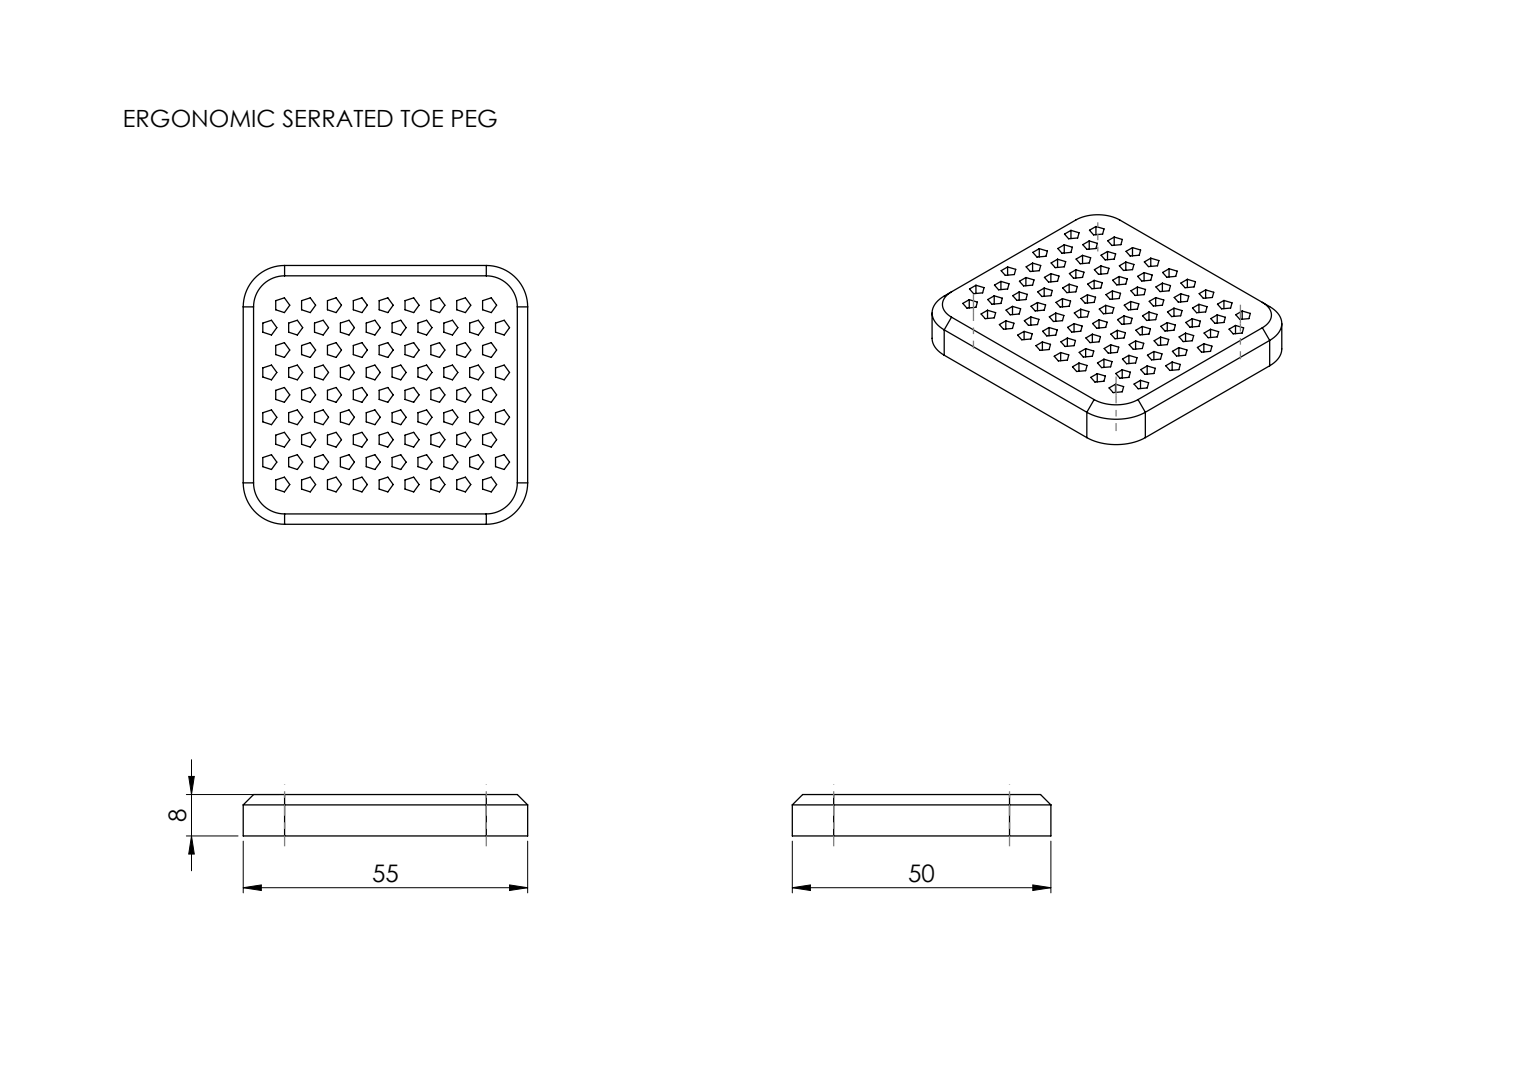
ISO-10303-21;
HEADER;
FILE_DESCRIPTION (('STEP AP214'),
    '1' );
FILE_NAME ('Ergonomic Serrated Toe Peg.step',
    '2026-09-30T16:28:02',
    ( '' ),
    ( '' ),
    'SwSTEP 2.0',
    'SolidWorks 2026',
    '' );
FILE_SCHEMA (( 'AUTOMOTIVE_DESIGN' ));
ENDSEC;

DATA;
#1=CARTESIAN_POINT ( 'NONE',  ( 171.1922820468852819, -9.999999999999996447, -4.936203717676158398 ) ) ;
#2=LINE ( 'NONE', #9287, #2166 ) ;
#6=ORIENTED_EDGE ( 'NONE', *, *, #8201, .T. ) ;
#8=EDGE_LOOP ( 'NONE', ( #13410, #18933, #24855, #7147 ) ) ;
#9=CARTESIAN_POINT ( 'NONE',  ( 158.6922820468853104, -1.999999999999974909, -0.6060766987539614181 ) ) ;
#13=AXIS2_PLACEMENT_3D ( 'NONE', #28994, #19329, #14737 ) ;
#14=VERTEX_POINT ( 'NONE', #15281 ) ;
#16=CARTESIAN_POINT ( 'NONE',  ( 176.1922820468852535, -9.999999999999994671, -4.936203717676158398 ) ) ;
#19=CARTESIAN_POINT ( 'NONE',  ( 129.5152310637605524, -10.00000000000000888, -21.71180489736090991 ) ) ;
#20=LINE ( 'NONE', #28431, #3804 ) ;
#22=ORIENTED_EDGE ( 'NONE', *, *, #9858, .T. ) ;
#23=DIRECTION ( 'NONE',  ( -0.5877852522924731371, 0.000000000000000000, 0.8090169943749474513 ) ) ;
#24=EDGE_LOOP ( 'NONE', ( #18208, #203, #15820, #9762, #20509 ) ) ;
#27=EDGE_CURVE ( 'NONE', #25495, #12783, #12701, .T. ) ;
#30=ORIENTED_EDGE ( 'NONE', *, *, #5505, .F. ) ;
#31=EDGE_CURVE ( 'NONE', #25811, #28060, #3559, .T. ) ;
#32=FACE_OUTER_BOUND ( 'NONE', #14723, .T. ) ;
#33=CARTESIAN_POINT ( 'NONE',  ( 142.0152310637605524, -1.999999999999978684, 1.702185954127501066 ) ) ;
#34=VECTOR ( 'NONE', #18733, 1000.000000000000000 ) ;
#36=AXIS2_PLACEMENT_3D ( 'NONE', #24795, #28817, #15305 ) ;
#38=VECTOR ( 'NONE', #16062, 999.9999999999998863 ) ;
#40=ORIENTED_EDGE ( 'NONE', *, *, #8836, .F. ) ;
#41=DIRECTION ( 'NONE',  ( -2.698458740408365879E-16, 1.000000000000000000, 0.000000000000000000 ) ) ;
#43=EDGE_LOOP ( 'NONE', ( #10791, #17120, #27313, #27403, #18272 ) ) ;
#45=DIRECTION ( 'NONE',  ( 2.908569913943825554E-16, -1.000000000000000000, 0.000000000000000000 ) ) ;
#46=ORIENTED_EDGE ( 'NONE', *, *, #12896, .F. ) ;
#47=CARTESIAN_POINT ( 'NONE',  ( 149.7287565553229456, -10.00000000000000355, 0.8205080756887930260 ) ) ;
#49=LINE ( 'NONE', #2798, #15810 ) ;
#50=EDGE_LOOP ( 'NONE', ( #6565, #21196, #16941, #11430, #26912 ) ) ;
#52=EDGE_LOOP ( 'NONE', ( #7879, #12886, #2199, #3337, #17093, #20123 ) ) ;
#55=ORIENTED_EDGE ( 'NONE', *, *, #7367, .F. ) ;
#57=CARTESIAN_POINT ( 'NONE',  ( 142.2287565553230309, -10.00000000000000533, -29.49038105676660138 ) ) ;
#59=ORIENTED_EDGE ( 'NONE', *, *, #1895, .T. ) ;
#60=LINE ( 'NONE', #7229, #30116 ) ;
#62=EDGE_CURVE ( 'NONE', #29710, #22500, #27244, .T. ) ;
#65=ADVANCED_FACE ( 'NONE', ( #1579 ), #24770, .T. ) ;
#69=EDGE_LOOP ( 'NONE', ( #19720, #1724, #9767, #14173 ) ) ;
#70=PLANE ( 'NONE',  #26676 ) ;
#71=ORIENTED_EDGE ( 'NONE', *, *, #5370, .F. ) ;
#75=ORIENTED_EDGE ( 'NONE', *, *, #15408, .T. ) ;
#76=VECTOR ( 'NONE', #4215, 1000.000000000000000 ) ;
#77=CARTESIAN_POINT ( 'NONE',  ( 133.7287565553229456, -4.999999999999982236, 3.500000000000003109 ) ) ;
#78=VECTOR ( 'NONE', #21293, 999.9999999999998863 ) ;
#79=LINE ( 'NONE', #18686, #13812 ) ;
#80=DIRECTION ( 'NONE',  ( 0.9510565162951536422, 0.000000000000000000, -0.3090169943749475623 ) ) ;
#81=CARTESIAN_POINT ( 'NONE',  ( 164.5152310637605240, -9.999999999999996447, -28.60870317832789667 ) ) ;
#82=DIRECTION ( 'NONE',  ( -1.110223024625156540E-16, 0.000000000000000000, -1.000000000000000000 ) ) ;
#86=EDGE_CURVE ( 'NONE', #12166, #722, #15592, .T. ) ;
#90=PLANE ( 'NONE',  #29362 ) ;
#91=DIRECTION ( 'NONE',  ( -2.698458740408365879E-16, 1.000000000000000000, 0.000000000000000000 ) ) ;
#92=DIRECTION ( 'NONE',  ( -0.9510565162951536422, 0.000000000000000000, -0.3090169943749472292 ) ) ;
#93=ORIENTED_EDGE ( 'NONE', *, *, #14811, .T. ) ;
#96=ORIENTED_EDGE ( 'NONE', *, *, #21204, .F. ) ;
#97=CARTESIAN_POINT ( 'NONE',  ( 164.5152310637604671, -9.999999999999998224, -11.28819510263909542 ) ) ;
#98=CARTESIAN_POINT ( 'NONE',  ( 152.0152310637604671, -4.999999999999976907, -0.06116980274991495881 ) ) ;
#99=ADVANCED_FACE ( 'NONE', ( #8123 ), #7974, .T. ) ;
#102=VERTEX_POINT ( 'NONE', #17428 ) ;
#105=EDGE_LOOP ( 'NONE', ( #1685, #5636, #6833, #29745, #13110 ) ) ;
#110=ORIENTED_EDGE ( 'NONE', *, *, #8360, .T. ) ;
#113=EDGE_LOOP ( 'NONE', ( #1842, #6412, #14178, #16562 ) ) ;
#114=CARTESIAN_POINT ( 'NONE',  ( 141.1922820468854525, -10.00000000000000533, -30.91696583120935671 ) ) ;
#115=CARTESIAN_POINT ( 'NONE',  ( 171.1922820468853388, -4.999999999999971578, -19.40354224447947828 ) ) ;
#117=VERTEX_POINT ( 'NONE', #8423 ) ;
#118=CARTESIAN_POINT ( 'NONE',  ( 134.5152310637605524, -1.999999999999980460, -4.391296821672111328 ) ) ;
#119=FACE_OUTER_BOUND ( 'NONE', #9403, .T. ) ;
#122=ORIENTED_EDGE ( 'NONE', *, *, #28451, .T. ) ;
#123=AXIS2_PLACEMENT_3D ( 'NONE', #1550, #9129, #25482 ) ;
#124=DIRECTION ( 'NONE',  ( 0.9510565162951536422, 0.000000000000000000, -0.3090169943749475623 ) ) ;
#125=CARTESIAN_POINT ( 'NONE',  ( 158.6922820468854241, -1.999999999999973133, -35.24709285013155835 ) ) ;
#128=CARTESIAN_POINT ( 'NONE',  ( 174.5152310637604955, -1.999999999999968914, -28.60870317832789667 ) ) ;
#130=DIRECTION ( 'NONE',  ( -0.5877852522924731371, -1.586114251531760728E-16, -0.8090169943749474513 ) ) ;
#131=EDGE_CURVE ( 'NONE', #19668, #13066, #17725, .T. ) ;
#132=LINE ( 'NONE', #2726, #539 ) ;
#133=VECTOR ( 'NONE', #22097, 1000.000000000000000 ) ;
#134=VERTEX_POINT ( 'NONE', #3860 ) ;
#136=LINE ( 'NONE', #8159, #30161 ) ;
#142=ORIENTED_EDGE ( 'NONE', *, *, #977, .F. ) ;
#144=FACE_OUTER_BOUND ( 'NONE', #11125, .T. ) ;
#146=DIRECTION ( 'NONE',  ( 0.5877852522924731371, 1.586114251531760728E-16, 0.8090169943749474513 ) ) ;
#148=AXIS2_PLACEMENT_3D ( 'NONE', #18004, #8395, #8543 ) ;
#152=LINE ( 'NONE', #16311, #22917 ) ;
#154=VECTOR ( 'NONE', #27172, 1000.000000000000000 ) ;
#155=EDGE_CURVE ( 'NONE', #6429, #19044, #27953, .T. ) ;
#161=ORIENTED_EDGE ( 'NONE', *, *, #1761, .F. ) ;
#162=LINE ( 'NONE', #17082, #29052 ) ;
#165=CARTESIAN_POINT ( 'NONE',  ( 21.73040598723229877, -5.000000000000011546, -66.87931276303945083 ) ) ;
#166=EDGE_LOOP ( 'NONE', ( #11300, #21186, #18431, #15934 ) ) ;
#167=VECTOR ( 'NONE', #27934, 1000.000000000000000 ) ;
#168=ORIENTED_EDGE ( 'NONE', *, *, #18099, .T. ) ;
#170=CARTESIAN_POINT ( 'NONE',  ( 125.7287565553229172, -4.000000000000003553, -33.50000000000000000 ) ) ;
#172=DIRECTION ( 'NONE',  ( -0.9510565162951536422, -2.566386769018988323E-16, 0.3090169943749475623 ) ) ;
#173=CARTESIAN_POINT ( 'NONE',  ( 136.1922820468854241, -1.999999999999980460, -19.40354224447947473 ) ) ;
#176=CARTESIAN_POINT ( 'NONE',  ( 168.6922820468853104, -9.999999999999998224, -6.413161187712876909 ) ) ;
#177=ORIENTED_EDGE ( 'NONE', *, *, #22974, .T. ) ;
#178=EDGE_CURVE ( 'NONE', #21232, #6302, #23638, .T. ) ;
#180=ORIENTED_EDGE ( 'NONE', *, *, #14435, .F. ) ;
#185=LINE ( 'NONE', #484, #11097 ) ;
#187=DIRECTION ( 'NONE',  ( -0.5877852522924731371, -1.586114251531760728E-16, -0.8090169943749474513 ) ) ;
#191=ORIENTED_EDGE ( 'NONE', *, *, #12444, .F. ) ;
#192=FACE_BOUND ( 'NONE', #6466, .T. ) ;
#193=ORIENTED_EDGE ( 'NONE', *, *, #2861, .F. ) ;
#194=EDGE_CURVE ( 'NONE', #21176, #29420, #19051, .T. ) ;
#195=ADVANCED_FACE ( 'NONE', ( #2293 ), #12020, .T. ) ;
#196=FACE_OUTER_BOUND ( 'NONE', #7916, .T. ) ;
#197=DIRECTION ( 'NONE',  ( -0.5877852522924731371, -1.586114251531760728E-16, -0.8090169943749474513 ) ) ;
#198=LINE ( 'NONE', #11177, #23639 ) ;
#199=VECTOR ( 'NONE', #16621, 1000.000000000000000 ) ;
#201=CARTESIAN_POINT ( 'NONE',  ( 11.95300070842526274, -5.000000000000014211, 36.78755350016455594 ) ) ;
#203=ORIENTED_EDGE ( 'NONE', *, *, #27651, .T. ) ;
#205=ORIENTED_EDGE ( 'NONE', *, *, #21724, .F. ) ;
#207=DIRECTION ( 'NONE',  ( -0.9510565162951536422, -2.566386769018988323E-16, 0.3090169943749475623 ) ) ;
#208=CARTESIAN_POINT ( 'NONE',  ( 161.1922820468853388, -9.999999999999998224, -13.59645775552055902 ) ) ;
#209=VERTEX_POINT ( 'NONE', #7460 ) ;
#212=FACE_OUTER_BOUND ( 'NONE', #25235, .T. ) ;
#214=ORIENTED_EDGE ( 'NONE', *, *, #14160, .F. ) ;
#216=CARTESIAN_POINT ( 'NONE',  ( 172.7287565553229456, -1.999999999999974021, -33.50000000000000000 ) ) ;
#217=ORIENTED_EDGE ( 'NONE', *, *, #1804, .F. ) ;
#218=CARTESIAN_POINT ( 'NONE',  ( 164.5152310637604671, -4.999999999999973355, -1.826485974285146553E-14 ) ) ;
#220=VERTEX_POINT ( 'NONE', #14001 ) ;
#221=DIRECTION ( 'NONE',  ( 0.9510565162951536422, 0.000000000000000000, -0.3090169943749475623 ) ) ;
#222=ORIENTED_EDGE ( 'NONE', *, *, #14772, .T. ) ;
#225=VECTOR ( 'NONE', #26675, 1000.000000000000000 ) ;
#226=ORIENTED_EDGE ( 'NONE', *, *, #24841, .F. ) ;
#227=ORIENTED_EDGE ( 'NONE', *, *, #21857, .F. ) ;
#228=CARTESIAN_POINT ( 'NONE',  ( 163.6922820468852819, -9.999999999999998224, -0.6060766987539614181 ) ) ;
#229=CARTESIAN_POINT ( 'NONE',  ( 151.1922820468853672, -1.999999999999976685, -2.083034168790677043 ) ) ;
#230=EDGE_CURVE ( 'NONE', #17843, #12321, #21337, .T. ) ;
#231=EDGE_CURVE ( 'NONE', #23545, #23604, #24924, .T. ) ;
#232=DIRECTION ( 'NONE',  ( -2.698458740408365879E-16, 1.000000000000000000, 0.000000000000000000 ) ) ;
#233=DIRECTION ( 'NONE',  ( -2.698458740408365879E-16, 1.000000000000000000, 0.000000000000000000 ) ) ;
#234=EDGE_CURVE ( 'NONE', #25907, #1746, #23486, .T. ) ;
#235=DIRECTION ( 'NONE',  ( 0.3090169943749475623, 8.338696094058001131E-17, 0.9510565162951536422 ) ) ;
#236=EDGE_LOOP ( 'NONE', ( #22910, #13879, #24086, #12025 ) ) ;
#237=ADVANCED_FACE ( 'NONE', ( #2593 ), #18453, .T. ) ;
#244=DIRECTION ( 'NONE',  ( 0.3090169943749475623, 8.338696094058001131E-17, 0.9510565162951536422 ) ) ;
#245=VECTOR ( 'NONE', #20484, 999.9999999999998863 ) ;
#246=CARTESIAN_POINT ( 'NONE',  ( 157.0152310637605808, -4.999999999999975131, -32.93883019725009120 ) ) ;
#247=DIRECTION ( 'NONE',  ( -0.9510565162951536422, -2.566386769018988816E-16, -0.3090169943749472292 ) ) ;
#250=CARTESIAN_POINT ( 'NONE',  ( 169.5152310637604955, -1.999999999999970024, -30.37205893520531319 ) ) ;
#252=EDGE_LOOP ( 'NONE', ( #8891, #22753, #23266, #17300 ) ) ;
#253=LINE ( 'NONE', #12283, #20751 ) ;
#254=LINE ( 'NONE', #28368, #19057 ) ;
#263=ORIENTED_EDGE ( 'NONE', *, *, #16267, .F. ) ;
#264=AXIS2_PLACEMENT_3D ( 'NONE', #8989, #18309, #27664 ) ;
#265=ORIENTED_EDGE ( 'NONE', *, *, #4022, .T. ) ;
#266=DIRECTION ( 'NONE',  ( 0.9510565162951536422, 0.000000000000000000, -0.3090169943749475623 ) ) ;
#267=PLANE ( 'NONE',  #1442 ) ;
#269=PLANE ( 'NONE',  #1205 ) ;
#270=EDGE_CURVE ( 'NONE', #13418, #14798, #2444, .T. ) ;
#271=DIRECTION ( 'NONE',  ( -2.698458740408365879E-16, 1.000000000000000000, 0.000000000000000000 ) ) ;
#274=ORIENTED_EDGE ( 'NONE', *, *, #12172, .T. ) ;
#275=LINE ( 'NONE', #12157, #28348 ) ;
#276=DIRECTION ( 'NONE',  ( 0.9510565162951536422, 0.000000000000000000, -0.3090169943749475623 ) ) ;
#278=DIRECTION ( 'NONE',  ( -2.698458740408365879E-16, 1.000000000000000000, 0.000000000000000000 ) ) ;
#279=DIRECTION ( 'NONE',  ( -0.5877852522924731371, -1.586114251531760728E-16, -0.8090169943749474513 ) ) ;
#280=VERTEX_POINT ( 'NONE', #21039 ) ;
#281=VECTOR ( 'NONE', #14887, 1000.000000000000000 ) ;
#282=DIRECTION ( 'NONE',  ( -0.8090169943749474513, -2.183098979609982436E-16, 0.5877852522924731371 ) ) ;
#284=LINE ( 'NONE', #14293, #25869 ) ;
#285=ORIENTED_EDGE ( 'NONE', *, *, #11613, .T. ) ;
#286=ORIENTED_EDGE ( 'NONE', *, *, #25521, .T. ) ;
#287=DIRECTION ( 'NONE',  ( 0.9510565162951536422, 2.566386769018988816E-16, 0.3090169943749472292 ) ) ;
#288=VERTEX_POINT ( 'NONE', #4857 ) ;
#292=DIRECTION ( 'NONE',  ( -0.5877852522924731371, -1.586114251531760235E-16, 0.8090169943749474513 ) ) ;
#294=CARTESIAN_POINT ( 'NONE',  ( 176.1922820468852535, -1.999999999999970024, -4.936203717676158398 ) ) ;
#295=EDGE_CURVE ( 'NONE', #18615, #29151, #11869, .T. ) ;
#297=VECTOR ( 'NONE', #130, 1000.000000000000000 ) ;
#298=ORIENTED_EDGE ( 'NONE', *, *, #1039, .F. ) ;
#299=DIRECTION ( 'NONE',  ( -0.9510565162951536422, -2.566386769018988323E-16, 0.3090169943749475623 ) ) ;
#300=LINE ( 'NONE', #23185, #15709 ) ;
#301=VECTOR ( 'NONE', #6965, 1000.000000000000000 ) ;
#305=AXIS2_PLACEMENT_3D ( 'NONE', #1101, #17395, #12671 ) ;
#306=CARTESIAN_POINT ( 'NONE',  ( 169.7287565553228887, -9.999999999999998224, -7.839745962155603820 ) ) ;
#307=EDGE_CURVE ( 'NONE', #30043, #633, #23795, .T. ) ;
#308=EDGE_CURVE ( 'NONE', #11681, #9083, #21945, .T. ) ;
#315=DIRECTION ( 'NONE',  ( -0.5877852522924731371, -1.586114251531760728E-16, -0.8090169943749474513 ) ) ;
#318=FACE_BOUND ( 'NONE', #13580, .T. ) ;
#319=VERTEX_POINT ( 'NONE', #1201 ) ;
#320=ORIENTED_EDGE ( 'NONE', *, *, #6013, .F. ) ;
#322=CARTESIAN_POINT ( 'NONE',  ( 174.7287565553229172, -9.999999999999994671, -25.16025403784440329 ) ) ;
#325=DIRECTION ( 'NONE',  ( -0.5877852522924731371, -1.586114251531760235E-16, 0.8090169943749474513 ) ) ;
#326=PLANE ( 'NONE',  #24744 ) ;
#327=ORIENTED_EDGE ( 'NONE', *, *, #10733, .F. ) ;
#332=VECTOR ( 'NONE', #22511, 1000.000000000000000 ) ;
#336=VECTOR ( 'NONE', #15406, 1000.000000000000000 ) ;
#343=FACE_BOUND ( 'NONE', #27021, .T. ) ;
#344=VECTOR ( 'NONE', #10715, 1000.000000000000000 ) ;
#345=ORIENTED_EDGE ( 'NONE', *, *, #10601, .T. ) ;
#346=ADVANCED_FACE ( 'NONE', ( #19194 ), #5318, .T. ) ;
#348=PLANE ( 'NONE',  #22330 ) ;
#349=LINE ( 'NONE', #4913, #4348 ) ;
#350=VECTOR ( 'NONE', #1226, 1000.000000000000000 ) ;
#352=AXIS2_PLACEMENT_3D ( 'NONE', #15421, #11403, #30099 ) ;
#354=CARTESIAN_POINT ( 'NONE',  ( 151.1922820468853672, -4.999999999999976907, -4.936203717676158398 ) ) ;
#355=AXIS2_PLACEMENT_3D ( 'NONE', #20040, #29561, #1592 ) ;
#356=FACE_OUTER_BOUND ( 'NONE', #20596, .T. ) ;
#357=VERTEX_POINT ( 'NONE', #9882 ) ;
#362=CARTESIAN_POINT ( 'NONE',  ( 180.7287565553229456, -3.999999999999989786, 0.5000000000000029976 ) ) ;
#364=LINE ( 'NONE', #23553, #20283 ) ;
#366=ORIENTED_EDGE ( 'NONE', *, *, #25702, .F. ) ;
#368=LINE ( 'NONE', #18674, #9316 ) ;
#369=CARTESIAN_POINT ( 'NONE',  ( 173.6922820468853104, -9.999999999999994671, -17.92658477444275889 ) ) ;
#372=ORIENTED_EDGE ( 'NONE', *, *, #2420, .F. ) ;
#374=EDGE_CURVE ( 'NONE', #25209, #19520, #2893, .T. ) ;
#376=CIRCLE ( 'NONE', #18872, 3.000000000000002665 ) ;
#378=ORIENTED_EDGE ( 'NONE', *, *, #6683, .T. ) ;
#380=CARTESIAN_POINT ( 'NONE',  ( 144.5152310637605240, -4.999999999999978684, -4.391296821672111328 ) ) ;
#381=CARTESIAN_POINT ( 'NONE',  ( 172.7287565553229456, -3.999999999999989786, -41.50000000000000711 ) ) ;
#384=CARTESIAN_POINT ( 'NONE',  ( 174.5152310637604103, -4.999999999999970690, -1.937508276747661576E-14 ) ) ;
#385=AXIS2_PLACEMENT_3D ( 'NONE', #29992, #3996, #22923 ) ;
#386=ORIENTED_EDGE ( 'NONE', *, *, #10034, .F. ) ;
#391=ORIENTED_EDGE ( 'NONE', *, *, #6783, .T. ) ;
#393=LINE ( 'NONE', #19002, #17550 ) ;
#394=CARTESIAN_POINT ( 'NONE',  ( 151.1922820468853956, -10.00000000000000178, -10.74328820663507678 ) ) ;
#402=EDGE_LOOP ( 'NONE', ( #24156, #22408, #9241, #18567 ) ) ;
#406=ORIENTED_EDGE ( 'NONE', *, *, #21308, .T. ) ;
#408=ADVANCED_FACE ( 'NONE', ( #24392 ), #12626, .T. ) ;
#411=EDGE_CURVE ( 'NONE', #18619, #29440, #26701, .T. ) ;
#413=VECTOR ( 'NONE', #9450, 1000.000000000000000 ) ;
#415=VECTOR ( 'NONE', #2292, 1000.000000000000000 ) ;
#416=ORIENTED_EDGE ( 'NONE', *, *, #15789, .T. ) ;
#417=DIRECTION ( 'NONE',  ( 0.3090169943749475623, 8.338696094058001131E-17, 0.9510565162951536422 ) ) ;
#418=DIRECTION ( 'NONE',  ( -2.698458740408365879E-16, 1.000000000000000000, 0.000000000000000000 ) ) ;
#419=EDGE_LOOP ( 'NONE', ( #26721, #25285, #4227, #20986 ) ) ;
#420=DIRECTION ( 'NONE',  ( 0.3090169943749475623, 8.338696094058001131E-17, 0.9510565162951536422 ) ) ;
#421=LINE ( 'NONE', #18729, #12178 ) ;
#424=ORIENTED_EDGE ( 'NONE', *, *, #5508, .F. ) ;
#425=CARTESIAN_POINT ( 'NONE',  ( 18.07240892486890615, -5.000000000000012434, -55.62115542516819744 ) ) ;
#426=CARTESIAN_POINT ( 'NONE',  ( 131.1922820468854241, -1.999999999999981792, -28.06379628232387446 ) ) ;
#429=LINE ( 'NONE', #19037, #21295 ) ;
#430=ORIENTED_EDGE ( 'NONE', *, *, #4985, .T. ) ;
#431=VECTOR ( 'NONE', #12408, 1000.000000000000000 ) ;
#432=CARTESIAN_POINT ( 'NONE',  ( 159.5152310637604955, -4.999999999999974243, -11.28819510263909542 ) ) ;
#435=CARTESIAN_POINT ( 'NONE',  ( 134.5152310637605524, -1.999999999999980460, -13.05155085951650840 ) ) ;
#436=VERTEX_POINT ( 'NONE', #19791 ) ;
#439=EDGE_CURVE ( 'NONE', #26227, #4517, #895, .T. ) ;
#442=EDGE_CURVE ( 'NONE', #18552, #1065, #26238, .T. ) ;
#444=LINE ( 'NONE', #2443, #25266 ) ;
#446=EDGE_CURVE ( 'NONE', #20723, #20491, #23957, .T. ) ;
#449=ORIENTED_EDGE ( 'NONE', *, *, #11568, .T. ) ;
#450=DIRECTION ( 'NONE',  ( -1.110223024625156540E-16, 0.000000000000000000, -1.000000000000000000 ) ) ;
#452=VECTOR ( 'NONE', #19393, 1000.000000000000000 ) ;
#453=DIRECTION ( 'NONE',  ( 0.3090169943749472292, 8.338696094057992503E-17, -0.9510565162951536422 ) ) ;
#455=LINE ( 'NONE', #21049, #14790 ) ;
#457=DIRECTION ( 'NONE',  ( 1.000000000000000000, 2.698458740408365879E-16, -1.110223024625156540E-16 ) ) ;
#459=ORIENTED_EDGE ( 'NONE', *, *, #24414, .T. ) ;
#468=ORIENTED_EDGE ( 'NONE', *, *, #9842, .F. ) ;
#470=FACE_OUTER_BOUND ( 'NONE', #17896, .T. ) ;
#472=FACE_OUTER_BOUND ( 'NONE', #16901, .T. ) ;
#473=ORIENTED_EDGE ( 'NONE', *, *, #13528, .T. ) ;
#475=VERTEX_POINT ( 'NONE', #12779 ) ;
#477=ORIENTED_EDGE ( 'NONE', *, *, #15791, .T. ) ;
#482=ORIENTED_EDGE ( 'NONE', *, *, #14397, .T. ) ;
#483=EDGE_CURVE ( 'NONE', #29391, #7152, #10029, .T. ) ;
#484=CARTESIAN_POINT ( 'NONE',  ( 12.50940683846913970, -5.000000000000014211, 38.49999548658399107 ) ) ;
#485=EDGE_CURVE ( 'NONE', #18308, #9388, #28550, .T. ) ;
#486=VERTEX_POINT ( 'NONE', #7602 ) ;
#487=EDGE_CURVE ( 'NONE', #4418, #10786, #7903, .T. ) ;
#490=DIRECTION ( 'NONE',  ( -2.698458740408365879E-16, 1.000000000000000000, 0.000000000000000000 ) ) ;
#494=ORIENTED_EDGE ( 'NONE', *, *, #2114, .T. ) ;
#495=FACE_BOUND ( 'NONE', #28944, .T. ) ;
#499=VECTOR ( 'NONE', #27812, 1000.000000000000000 ) ;
#500=DIRECTION ( 'NONE',  ( 0.9510565162951536422, 2.566386769018988816E-16, 0.3090169943749472292 ) ) ;
#504=DIRECTION ( 'NONE',  ( -2.698458740408365879E-16, 1.000000000000000000, 0.000000000000000000 ) ) ;
#505=CARTESIAN_POINT ( 'NONE',  ( 162.0152310637605240, -9.999999999999998224, -34.70218595412750773 ) ) ;
#506=VERTEX_POINT ( 'NONE', #26086 ) ;
#509=LINE ( 'NONE', #21850, #18033 ) ;
#510=LINE ( 'NONE', #23703, #12518 ) ;
#511=CARTESIAN_POINT ( 'NONE',  ( 137.0152310637605808, -1.999999999999980016, 1.702185954127501066 ) ) ;
#512=ORIENTED_EDGE ( 'NONE', *, *, #5043, .F. ) ;
#513=LINE ( 'NONE', #12092, #15899 ) ;
#518=VECTOR ( 'NONE', #4177, 1000.000000000000000 ) ;
#520=EDGE_CURVE ( 'NONE', #12932, #5386, #5166, .T. ) ;
#521=CARTESIAN_POINT ( 'NONE',  ( 130.7287565553229456, -4.999999999999983125, 3.500000000000003109 ) ) ;
#524=ADVANCED_FACE ( 'NONE', ( #22562 ), #3633, .T. ) ;
#525=ORIENTED_EDGE ( 'NONE', *, *, #27075, .F. ) ;
#526=ADVANCED_FACE ( 'NONE', ( #15359 ), #12926, .T. ) ;
#527=LINE ( 'NONE', #9813, #17849 ) ;
#532=VECTOR ( 'NONE', #22824, 1000.000000000000000 ) ;
#534=LINE ( 'NONE', #822, #24024 ) ;
#535=EDGE_LOOP ( 'NONE', ( #7211, #6231, #28486, #4893 ) ) ;
#536=ORIENTED_EDGE ( 'NONE', *, *, #4318, .F. ) ;
#537=CARTESIAN_POINT ( 'NONE',  ( 146.1922820468854525, -10.00000000000000178, -22.25671179336496053 ) ) ;
#538=CARTESIAN_POINT ( 'NONE',  ( 139.5152310637605808, -10.00000000000000533, -21.71180489736090991 ) ) ;
#539=VECTOR ( 'NONE', #19186, 999.9999999999998863 ) ;
#541=DIRECTION ( 'NONE',  ( 0.000000000000000000, 0.000000000000000000, -1.000000000000000000 ) ) ;
#542=VECTOR ( 'NONE', #24235, 1000.000000000000000 ) ;
#543=CARTESIAN_POINT ( 'NONE',  ( 12.10607290817362092, -5.000000000000014211, -37.25866128932931787 ) ) ;
#544=ORIENTED_EDGE ( 'NONE', *, *, #13525, .F. ) ;
#548=EDGE_CURVE ( 'NONE', #20384, #24083, #19953, .T. ) ;
#550=ORIENTED_EDGE ( 'NONE', *, *, #23991, .F. ) ;
#552=DIRECTION ( 'NONE',  ( 0.9510565162951536422, 0.000000000000000000, -0.3090169943749475623 ) ) ;
#554=CARTESIAN_POINT ( 'NONE',  ( 148.6922820468854525, -4.999999999999976907, -23.73366926340167637 ) ) ;
#556=EDGE_LOOP ( 'NONE', ( #3105, #12356, #15207, #22632, #19486 ) ) ;
#557=FACE_OUTER_BOUND ( 'NONE', #419, .T. ) ;
#559=LINE ( 'NONE', #9844, #18339 ) ;
#560=DIRECTION ( 'NONE',  ( 2.698458740408365879E-16, -1.000000000000000000, 0.000000000000000000 ) ) ;
#563=VERTEX_POINT ( 'NONE', #10643 ) ;
#567=AXIS2_PLACEMENT_3D ( 'NONE', #11521, #19011, #13959 ) ;
#571=CARTESIAN_POINT ( 'NONE',  ( 129.5152310637605808, -10.00000000000000888, -11.28819510263909187 ) ) ;
#572=DIRECTION ( 'NONE',  ( -0.9510565162951536422, 0.000000000000000000, -0.3090169943749472292 ) ) ;
#573=ORIENTED_EDGE ( 'NONE', *, *, #19437, .T. ) ;
#574=DIRECTION ( 'NONE',  ( -0.8090169943749474513, -2.183098979609982436E-16, -0.5877852522924731371 ) ) ;
#575=DIRECTION ( 'NONE',  ( 0.9510565162951536422, 0.000000000000000000, -0.3090169943749475623 ) ) ;
#576=ADVANCED_FACE ( 'NONE', ( #3939 ), #15213, .T. ) ;
#581=DIRECTION ( 'NONE',  ( 0.3090169943749472292, 8.338696094057992503E-17, -0.9510565162951536422 ) ) ;
#582=CARTESIAN_POINT ( 'NONE',  ( 106.2677862141057545, -4.999999999999988454, -77.20806604152963359 ) ) ;
#584=CARTESIAN_POINT ( 'NONE',  ( 138.6922820468854525, -4.999999999999980460, -23.73366926340167282 ) ) ;
#585=CARTESIAN_POINT ( 'NONE',  ( 153.6922820468854241, -1.999999999999974465, -23.73366926340167637 ) ) ;
#587=DIRECTION ( 'NONE',  ( -0.5877852522924731371, 0.000000000000000000, 0.8090169943749474513 ) ) ;
#588=CARTESIAN_POINT ( 'NONE',  ( 142.0152310637605808, -1.999999999999978018, -26.04193191628310800 ) ) ;
#590=VERTEX_POINT ( 'NONE', #3789 ) ;
#591=EDGE_LOOP ( 'NONE', ( #6929, #8428, #23827, #25905 ) ) ;
#592=ORIENTED_EDGE ( 'NONE', *, *, #18201, .T. ) ;
#596=CARTESIAN_POINT ( 'NONE',  ( 143.6922820468854525, -10.00000000000000355, -17.92658477444275889 ) ) ;
#598=VECTOR ( 'NONE', #146, 1000.000000000000000 ) ;
#599=CARTESIAN_POINT ( 'NONE',  ( 15.12871522451188788, -5.000000000000013323, -46.56139778509288618 ) ) ;
#600=VERTEX_POINT ( 'NONE', #24546 ) ;
#601=CARTESIAN_POINT ( 'NONE',  ( 175.7287565553229456, -4.999999999999969802, -4.785595155761525277 ) ) ;
#604=CARTESIAN_POINT ( 'NONE',  ( 148.6922820468854525, -1.999999999999977129, -32.39392330124607611 ) ) ;
#606=ADVANCED_FACE ( 'NONE', ( #5928 ), #17657, .T. ) ;
#607=ADVANCED_FACE ( 'NONE', ( #6073 ), #13083, .T. ) ;
#608=PLANE ( 'NONE',  #6779 ) ;
#610=ORIENTED_EDGE ( 'NONE', *, *, #3790, .F. ) ;
#612=EDGE_CURVE ( 'NONE', #12774, #3207, #13241, .T. ) ;
#613=FACE_OUTER_BOUND ( 'NONE', #14035, .T. ) ;
#614=AXIS2_PLACEMENT_3D ( 'NONE', #19499, #24547, #12781 ) ;
#615=ADVANCED_FACE ( 'NONE', ( #17802 ), #27165, .T. ) ;
#618=CARTESIAN_POINT ( 'NONE',  ( 162.0152310637604955, -4.999999999999974243, -26.04193191628311155 ) ) ;
#619=VERTEX_POINT ( 'NONE', #5420 ) ;
#623=CARTESIAN_POINT ( 'NONE',  ( 175.7287565553229456, -9.999999999999971578, 0.5000000000000029976 ) ) ;
#624=ORIENTED_EDGE ( 'NONE', *, *, #10904, .F. ) ;
#625=CARTESIAN_POINT ( 'NONE',  ( 173.6922820468853388, -9.999999999999994671, -26.58683881228715862 ) ) ;
#626=ORIENTED_EDGE ( 'NONE', *, *, #26015, .T. ) ;
#628=ORIENTED_EDGE ( 'NONE', *, *, #27617, .T. ) ;
#633=VERTEX_POINT ( 'NONE', #8295 ) ;
#635=CARTESIAN_POINT ( 'NONE',  ( 112.3900446700832845, -4.999999999999986677, -81.65614717723775584 ) ) ;
#638=VECTOR ( 'NONE', #15059, 1000.000000000000000 ) ;
#640=FACE_BOUND ( 'NONE', #17221, .T. ) ;
#641=ORIENTED_EDGE ( 'NONE', *, *, #6603, .T. ) ;
#642=CARTESIAN_POINT ( 'NONE',  ( 17.67390002678752126, -5.000000000000013323, -54.39467115012526932 ) ) ;
#644=CARTESIAN_POINT ( 'NONE',  ( 95.18167920860219056, -4.999999999999991118, -69.15353783201314286 ) ) ;
#646=DIRECTION ( 'NONE',  ( -0.9510565162951536422, -2.566386769018988323E-16, 0.3090169943749475623 ) ) ;
#647=EDGE_CURVE ( 'NONE', #21669, #19416, #14705, .T. ) ;
#652=FACE_OUTER_BOUND ( 'NONE', #21709, .T. ) ;
#655=VECTOR ( 'NONE', #19725, 1000.000000000000000 ) ;
#658=CARTESIAN_POINT ( 'NONE',  ( 10.52062816623737618, -5.000000000000015099, 32.37916410797102884 ) ) ;
#659=DIRECTION ( 'NONE',  ( -0.8090169943749474513, -2.183098979609982436E-16, -0.5877852522924731371 ) ) ;
#660=DIRECTION ( 'NONE',  ( 0.9510565162951536422, 0.000000000000000000, -0.3090169943749475623 ) ) ;
#665=DIRECTION ( 'NONE',  ( -0.5877852522924731371, 0.000000000000000000, 0.8090169943749474513 ) ) ;
#667=EDGE_LOOP ( 'NONE', ( #22957, #26404, #26057, #11822 ) ) ;
#668=PLANE ( 'NONE',  #10055 ) ;
#672=FACE_OUTER_BOUND ( 'NONE', #3393, .T. ) ;
#673=ORIENTED_EDGE ( 'NONE', *, *, #5089, .F. ) ;
#676=AXIS2_PLACEMENT_3D ( 'NONE', #24862, #20114, #1970 ) ;
#679=LINE ( 'NONE', #23575, #7743 ) ;
#680=EDGE_CURVE ( 'NONE', #19492, #2298, #29262, .T. ) ;
#681=EDGE_CURVE ( 'NONE', #10452, #25209, #7995, .T. ) ;
#685=EDGE_CURVE ( 'NONE', #16894, #18003, #12723, .T. ) ;
#689=ORIENTED_EDGE ( 'NONE', *, *, #5256, .F. ) ;
#690=CARTESIAN_POINT ( 'NONE',  ( 173.6922820468853388, -1.999999999999969580, -26.58683881228715862 ) ) ;
#693=DIRECTION ( 'NONE',  ( -2.698458740408365879E-16, 1.000000000000000000, 0.000000000000000000 ) ) ;
#696=ORIENTED_EDGE ( 'NONE', *, *, #23243, .F. ) ;
#697=CARTESIAN_POINT ( 'NONE',  ( 137.2287565553230309, -10.00000000000000533, -12.16987298107780013 ) ) ;
#699=DIRECTION ( 'NONE',  ( 1.000000000000000000, 2.908569913943825554E-16, -6.938893903907227392E-16 ) ) ;
#701=ORIENTED_EDGE ( 'NONE', *, *, #6410, .F. ) ;
#710=CARTESIAN_POINT ( 'NONE',  ( 143.6922820468854525, -1.999999999999977573, -32.39392330124607611 ) ) ;
#711=LINE ( 'NONE', #7438, #3635 ) ;
#712=VECTOR ( 'NONE', #11065, 1000.000000000000000 ) ;
#717=CARTESIAN_POINT ( 'NONE',  ( 174.5152310637604103, -9.999999999999994671, -13.05155085951651195 ) ) ;
#718=CARTESIAN_POINT ( 'NONE',  ( 19.66267869901929188, -5.000000000000012434, -60.51550252873825286 ) ) ;
#722=VERTEX_POINT ( 'NONE', #26337 ) ;
#723=FACE_OUTER_BOUND ( 'NONE', #23667, .T. ) ;
#724=PLANE ( 'NONE',  #2987 ) ;
#725=ORIENTED_EDGE ( 'NONE', *, *, #25327, .F. ) ;
#726=ORIENTED_EDGE ( 'NONE', *, *, #7705, .F. ) ;
#727=ORIENTED_EDGE ( 'NONE', *, *, #5882, .T. ) ;
#731=DIRECTION ( 'NONE',  ( -0.5877852522924731371, -1.586114251531760235E-16, 0.8090169943749474513 ) ) ;
#733=CARTESIAN_POINT ( 'NONE',  ( 175.7287565553229456, -9.999999999999971578, 3.500000000000003109 ) ) ;
#734=ADVANCED_FACE ( 'NONE', ( #24048 ), #17453, .T. ) ;
#735=PRODUCT_DEFINITION ( 'UNKNOWN', '', #23906, #23852 ) ;
#737=ORIENTED_EDGE ( 'NONE', *, *, #24223, .F. ) ;
#738=FACE_OUTER_BOUND ( 'NONE', #7045, .T. ) ;
#739=CARTESIAN_POINT ( 'NONE',  ( 162.0152310637604387, -9.999999999999998224, -8.721423840594312082 ) ) ;
#740=LINE ( 'NONE', #17220, #4845 ) ;
#741=LINE ( 'NONE', #28713, #2500 ) ;
#744=CARTESIAN_POINT ( 'NONE',  ( 173.6922820468853388, -1.999999999999969580, -26.58683881228715862 ) ) ;
#746=ORIENTED_EDGE ( 'NONE', *, *, #23165, .F. ) ;
#748=PLANE ( 'NONE',  #14393 ) ;
#749=VECTOR ( 'NONE', #646, 999.9999999999998863 ) ;
#754=ORIENTED_EDGE ( 'NONE', *, *, #14477, .F. ) ;
#755=ORIENTED_EDGE ( 'NONE', *, *, #24801, .T. ) ;
#756=VERTEX_POINT ( 'NONE', #10428 ) ;
#758=LINE ( 'NONE', #26413, #24784 ) ;
#760=PLANE ( 'NONE',  #1860 ) ;
#763=CARTESIAN_POINT ( 'NONE',  ( 154.7287565553229456, -10.00000000000000178, -7.839745962155603820 ) ) ;
#764=EDGE_LOOP ( 'NONE', ( #22617, #12498, #2134, #26269 ) ) ;
#766=VECTOR ( 'NONE', #5113, 1000.000000000000000 ) ;
#767=ORIENTED_EDGE ( 'NONE', *, *, #14651, .T. ) ;
#771=AXIS2_PLACEMENT_3D ( 'NONE', #11121, #24875, #20422 ) ;
#772=CARTESIAN_POINT ( 'NONE',  ( 131.1922820468854241, -10.00000000000000888, -28.06379628232387446 ) ) ;
#776=EDGE_CURVE ( 'NONE', #8035, #18677, #840, .T. ) ;
#778=VECTOR ( 'NONE', #13223, 1000.000000000000000 ) ;
#779=EDGE_CURVE ( 'NONE', #2626, #23142, #19737, .T. ) ;
#782=ORIENTED_EDGE ( 'NONE', *, *, #29502, .F. ) ;
#784=DIRECTION ( 'NONE',  ( -2.698458740408365879E-16, 1.000000000000000000, 0.000000000000000000 ) ) ;
#785=LINE ( 'NONE', #3830, #14240 ) ;
#787=CARTESIAN_POINT ( 'NONE',  ( 173.6922820468852819, -1.999999999999970468, -9.266330736598359152 ) ) ;
#788=DIRECTION ( 'NONE',  ( -0.5877852522924731371, -1.586114251531760235E-16, 0.8090169943749474513 ) ) ;
#791=VECTOR ( 'NONE', #22194, 1000.000000000000000 ) ;
#793=DIRECTION ( 'NONE',  ( -0.8090169943749474513, -2.183098979609982436E-16, 0.5877852522924731371 ) ) ;
#795=LINE ( 'NONE', #12527, #27612 ) ;
#796=ORIENTED_EDGE ( 'NONE', *, *, #28150, .F. ) ;
#797=CIRCLE ( 'NONE', #26173, 8.000000000000003553 ) ;
#799=EDGE_LOOP ( 'NONE', ( #24798, #19228, #20118, #16821 ) ) ;
#800=VECTOR ( 'NONE', #21735, 1000.000000000000000 ) ;
#802=CARTESIAN_POINT ( 'NONE',  ( 152.0152310637604955, -4.999999999999976907, 1.702185954127501066 ) ) ;
#803=LINE ( 'NONE', #7961, #4727 ) ;
#804=CARTESIAN_POINT ( 'NONE',  ( 133.6922820468854241, -10.00000000000000711, -23.73366926340167282 ) ) ;
#805=LINE ( 'NONE', #26606, #5198 ) ;
#806=ORIENTED_EDGE ( 'NONE', *, *, #20326, .T. ) ;
#808=ORIENTED_EDGE ( 'NONE', *, *, #14405, .T. ) ;
#811=CARTESIAN_POINT ( 'NONE',  ( 132.2287565553230024, -1.999999999999981348, -20.83012701892220164 ) ) ;
#813=ORIENTED_EDGE ( 'NONE', *, *, #2594, .T. ) ;
#814=CARTESIAN_POINT ( 'NONE',  ( 137.0152310637605808, -4.999999999999980460, -8.721423840594312082 ) ) ;
#817=EDGE_CURVE ( 'NONE', #1754, #23532, #7703, .T. ) ;
#819=EDGE_CURVE ( 'NONE', #18037, #28074, #13165, .T. ) ;
#822=CARTESIAN_POINT ( 'NONE',  ( 168.6922820468853388, -9.999999999999996447, -17.92658477444275889 ) ) ;
#823=EDGE_CURVE ( 'NONE', #15263, #5003, #24622, .T. ) ;
#824=EDGE_LOOP ( 'NONE', ( #12649, #746, #9170, #22264 ) ) ;
#825=CARTESIAN_POINT ( 'NONE',  ( 134.7287565553230024, -10.00000000000000711, -16.50000000000000000 ) ) ;
#826=AXIS2_PLACEMENT_3D ( 'NONE', #24727, #13267, #11272 ) ;
#829=CARTESIAN_POINT ( 'NONE',  ( 110.8088082477345750, -4.999999999999987566, -80.50731166957035612 ) ) ;
#830=VECTOR ( 'NONE', #26631, 1000.000000000000000 ) ;
#831=LINE ( 'NONE', #16848, #1420 ) ;
#838=DIRECTION ( 'NONE',  ( 0.5877852522924731371, 1.586114251531760728E-16, -0.8090169943749474513 ) ) ;
#839=FACE_OUTER_BOUND ( 'NONE', #11884, .T. ) ;
#840=LINE ( 'NONE', #12570, #26282 ) ;
#842=VECTOR ( 'NONE', #21103, 1000.000000000000000 ) ;
#843=LINE ( 'NONE', #28961, #20475 ) ;
#847=DIRECTION ( 'NONE',  ( -0.9510565162951536422, -2.566386769018988323E-16, 0.3090169943749475623 ) ) ;
#850=LINE ( 'NONE', #11826, #24678 ) ;
#851=DIRECTION ( 'NONE',  ( -0.9510565162951536422, -2.566386769018988323E-16, 0.3090169943749475623 ) ) ;
#855=ORIENTED_EDGE ( 'NONE', *, *, #1035, .F. ) ;
#860=ADVANCED_FACE ( 'NONE', ( #29558 ), #23186, .T. ) ;
#861=EDGE_CURVE ( 'NONE', #7930, #18591, #27811, .T. ) ;
#862=ADVANCED_FACE ( 'NONE', ( #11571 ), #27254, .T. ) ;
#863=ORIENTED_EDGE ( 'NONE', *, *, #8321, .F. ) ;
#865=VECTOR ( 'NONE', #21365, 1000.000000000000000 ) ;
#866=ORIENTED_EDGE ( 'NONE', *, *, #19340, .T. ) ;
#868=ORIENTED_EDGE ( 'NONE', *, *, #10306, .T. ) ;
#872=PLANE ( 'NONE',  #23612 ) ;
#877=DIRECTION ( 'NONE',  ( 0.5877852522924731371, 0.000000000000000000, 0.8090169943749474513 ) ) ;
#880=FACE_OUTER_BOUND ( 'NONE', #27488, .T. ) ;
#881=DIRECTION ( 'NONE',  ( 0.3090169943749472292, 8.338696094057992503E-17, -0.9510565162951536422 ) ) ;
#882=EDGE_LOOP ( 'NONE', ( #8366, #4789, #29727, #9280 ) ) ;
#884=CARTESIAN_POINT ( 'NONE',  ( 153.6922820468854525, -4.999999999999976907, -35.24709285013155835 ) ) ;
#886=DIRECTION ( 'NONE',  ( -2.698458740408365879E-16, 1.000000000000000000, 0.000000000000000000 ) ) ;
#888=VERTEX_POINT ( 'NONE', #12859 ) ;
#890=VECTOR ( 'NONE', #25219, 1000.000000000000000 ) ;
#892=EDGE_CURVE ( 'NONE', #29509, #10549, #17732, .T. ) ;
#894=CARTESIAN_POINT ( 'NONE',  ( 161.1922820468853672, -4.999999999999974243, -22.25671179336496053 ) ) ;
#895=LINE ( 'NONE', #15056, #12119 ) ;
#896=DIRECTION ( 'NONE',  ( -2.698458740408365879E-16, 1.000000000000000000, 0.000000000000000000 ) ) ;
#897=EDGE_CURVE ( 'NONE', #28202, #19572, #20324, .T. ) ;
#898=DIRECTION ( 'NONE',  ( -0.9510565162951536422, 0.000000000000000000, -0.3090169943749472292 ) ) ;
#899=DIRECTION ( 'NONE',  ( -0.8090169943749474513, -2.183098979609982436E-16, 0.5877852522924731371 ) ) ;
#900=LINE ( 'NONE', #27023, #12161 ) ;
#901=CIRCLE ( 'NONE', #17942, 3.000000000000002665 ) ;
#902=FACE_OUTER_BOUND ( 'NONE', #26467, .T. ) ;
#903=DIRECTION ( 'NONE',  ( -0.9510565162951536422, -2.566386769018988323E-16, 0.3090169943749475623 ) ) ;
#907=ORIENTED_EDGE ( 'NONE', *, *, #8004, .T. ) ;
#911=FACE_BOUND ( 'NONE', #4279, .T. ) ;
#912=VECTOR ( 'NONE', #20314, 1000.000000000000000 ) ;
#914=VECTOR ( 'NONE', #25269, 1000.000000000000000 ) ;
#915=ORIENTED_EDGE ( 'NONE', *, *, #8153, .T. ) ;
#916=CARTESIAN_POINT ( 'NONE',  ( 162.0152310637604671, -1.999999999999973133, -6.958068083716895558 ) ) ;
#918=LINE ( 'NONE', #1085, #25237 ) ;
#919=ORIENTED_EDGE ( 'NONE', *, *, #21721, .F. ) ;
#920=ORIENTED_EDGE ( 'NONE', *, *, #6229, .F. ) ;
#921=DIRECTION ( 'NONE',  ( 0.9510565162951535312, 2.566386769018988816E-16, -0.3090169943749475623 ) ) ;
#924=EDGE_LOOP ( 'NONE', ( #4638, #12101, #16492, #28325 ) ) ;
#929=VERTEX_POINT ( 'NONE', #8132 ) ;
#932=DIRECTION ( 'NONE',  ( -1.000000000000000000, -2.698458740408365879E-16, -0.000000000000000000 ) ) ;
#933=ORIENTED_EDGE ( 'NONE', *, *, #13523, .T. ) ;
#934=ADVANCED_FACE ( 'NONE', ( #1735 ), #10868, .T. ) ;
#935=CARTESIAN_POINT ( 'NONE',  ( 116.9310667037121618, -4.999999999999985789, -84.95539280527852100 ) ) ;
#939=VECTOR ( 'NONE', #6224, 1000.000000000000000 ) ;
#943=FACE_BOUND ( 'NONE', #7642, .T. ) ;
#944=LINE ( 'NONE', #28304, #14996 ) ;
#946=DIRECTION ( 'NONE',  ( 0.000000000000000000, -0.000000000000000000, 1.000000000000000000 ) ) ;
#947=DIRECTION ( 'NONE',  ( -0.8090169943749474513, -2.183098979609982436E-16, 0.5877852522924731371 ) ) ;
#950=EDGE_CURVE ( 'NONE', #2754, #23037, #3716, .T. ) ;
#954=DIRECTION ( 'NONE',  ( 0.5877852522924731371, 1.586114251531760728E-16, -0.8090169943749474513 ) ) ;
#955=ORIENTED_EDGE ( 'NONE', *, *, #19484, .F. ) ;
#957=EDGE_CURVE ( 'NONE', #10350, #9967, #5858, .T. ) ;
#960=LINE ( 'NONE', #16817, #5391 ) ;
#961=FACE_OUTER_BOUND ( 'NONE', #9465, .T. ) ;
#962=LINE ( 'NONE', #19256, #20960 ) ;
#963=AXIS2_PLACEMENT_3D ( 'NONE', #19317, #1029, #19468 ) ;
#964=ORIENTED_EDGE ( 'NONE', *, *, #15893, .F. ) ;
#965=CARTESIAN_POINT ( 'NONE',  ( 130.7287565553229456, -4.999999999999983125, -13.44584919360585928 ) ) ;
#966=VERTEX_POINT ( 'NONE', #15601 ) ;
#968=VERTEX_POINT ( 'NONE', #15141 ) ;
#972=LINE ( 'NONE', #10255, #5266 ) ;
#975=CARTESIAN_POINT ( 'NONE',  ( 168.6922820468853104, -9.999999999999998224, -9.266330736598359152 ) ) ;
#977=EDGE_CURVE ( 'NONE', #15701, #26572, #20177, .T. ) ;
#983=VERTEX_POINT ( 'NONE', #25625 ) ;
#985=AXIS2_PLACEMENT_3D ( 'NONE', #22908, #27222, #11143 ) ;
#987=DIRECTION ( 'NONE',  ( -0.9510565162951536422, -2.566386769018988816E-16, -0.3090169943749472292 ) ) ;
#990=DIRECTION ( 'NONE',  ( -2.698458740408365879E-16, 1.000000000000000000, 0.000000000000000000 ) ) ;
#991=LINE ( 'NONE', #3138, #6095 ) ;
#996=VECTOR ( 'NONE', #1452, 1000.000000000000000 ) ;
#998=ORIENTED_EDGE ( 'NONE', *, *, #19067, .T. ) ;
#1000=CARTESIAN_POINT ( 'NONE',  ( 91.73376360168730059, -4.999999999999992006, 66.64848051061605361 ) ) ;
#1001=DIRECTION ( 'NONE',  ( 0.5877852522924731371, 1.586114251531760728E-16, -0.8090169943749474513 ) ) ;
#1002=VECTOR ( 'NONE', #17125, 1000.000000000000000 ) ;
#1003=DIRECTION ( 'NONE',  ( 1.000000000000000000, 2.698458740408365879E-16, -1.110223024625156540E-16 ) ) ;
#1005=DIRECTION ( 'NONE',  ( -2.698458740408365879E-16, 1.000000000000000000, 0.000000000000000000 ) ) ;
#1006=CARTESIAN_POINT ( 'NONE',  ( 169.5152310637604671, -9.999999999999996447, -11.28819510263909542 ) ) ;
#1007=ADVANCED_FACE ( 'NONE', ( #23338 ), #28556, .T. ) ;
#1009=ORIENTED_EDGE ( 'NONE', *, *, #19272, .F. ) ;
#1010=LINE ( 'NONE', #28820, #28606 ) ;
#1012=VECTOR ( 'NONE', #14521, 1000.000000000000000 ) ;
#1013=LINE ( 'NONE', #17759, #10031 ) ;
#1014=CARTESIAN_POINT ( 'NONE',  ( 146.1922820468853956, -1.999999999999978018, -4.936203717676158398 ) ) ;
#1015=VECTOR ( 'NONE', #8319, 1000.000000000000000 ) ;
#1017=LINE ( 'NONE', #22058, #24247 ) ;
#1019=ORIENTED_EDGE ( 'NONE', *, *, #21791, .T. ) ;
#1026=VECTOR ( 'NONE', #2101, 1000.000000000000000 ) ;
#1027=PLANE ( 'NONE',  #29947 ) ;
#1028=ORIENTED_EDGE ( 'NONE', *, *, #20544, .T. ) ;
#1029=DIRECTION ( 'NONE',  ( 0.3090169943749475623, 8.338696094058001131E-17, 0.9510565162951536422 ) ) ;
#1030=PLANE ( 'NONE',  #3315 ) ;
#1031=DIRECTION ( 'NONE',  ( -0.9510565162951536422, 0.000000000000000000, -0.3090169943749472292 ) ) ;
#1032=CARTESIAN_POINT ( 'NONE',  ( 137.0152310637605808, -1.999999999999979572, -8.721423840594312082 ) ) ;
#1035=EDGE_CURVE ( 'NONE', #19382, #17985, #28108, .T. ) ;
#1036=CARTESIAN_POINT ( 'NONE',  ( 175.7287565553229456, -4.999999999999970690, -13.44584919360591257 ) ) ;
#1039=EDGE_CURVE ( 'NONE', #12109, #19638, #23490, .T. ) ;
#1042=EDGE_CURVE ( 'NONE', #18885, #9954, #9589, .T. ) ;
#1043=CARTESIAN_POINT ( 'NONE',  ( 175.7287565553229456, -4.999999999999970690, 3.500000000000003109 ) ) ;
#1044=VECTOR ( 'NONE', #19933, 999.9999999999998863 ) ;
#1045=EDGE_LOOP ( 'NONE', ( #15324, #2019, #2265, #5446 ) ) ;
#1048=DIRECTION ( 'NONE',  ( -0.8090169943749474513, -2.183098979609982436E-16, 0.5877852522924731371 ) ) ;
#1049=CARTESIAN_POINT ( 'NONE',  ( 15.37415192284491638, -5.000000000000013323, 47.31677427097104527 ) ) ;
#1051=ORIENTED_EDGE ( 'NONE', *, *, #13820, .T. ) ;
#1058=CARTESIAN_POINT ( 'NONE',  ( 136.1922820468854241, -1.999999999999980460, -13.59645775552055547 ) ) ;
#1059=LINE ( 'NONE', #26702, #13282 ) ;
#1060=ORIENTED_EDGE ( 'NONE', *, *, #27134, .T. ) ;
#1061=DIRECTION ( 'NONE',  ( -2.698458740408365879E-16, 1.000000000000000000, 0.000000000000000000 ) ) ;
#1063=CARTESIAN_POINT ( 'NONE',  ( 157.2287565553229456, -1.999999999999974021, -12.16987298107780369 ) ) ;
#1065=VERTEX_POINT ( 'NONE', #9889 ) ;
#1068=CARTESIAN_POINT ( 'NONE',  ( 142.0152310637605524, -10.00000000000000355, -8.721423840594312082 ) ) ;
#1070=EDGE_LOOP ( 'NONE', ( #27500, #26319, #424, #13784 ) ) ;
#1072=ORIENTED_EDGE ( 'NONE', *, *, #2270, .F. ) ;
#1074=PRODUCT ( 'Ergonomic Serrated Toe Peg', 'Ergonomic Serrated Toe Peg', '', ( #14944 ) ) ;
#1075=EDGE_CURVE ( 'NONE', #18592, #20355, #19201, .T. ) ;
#1077=ADVANCED_FACE ( 'NONE', ( #25938 ), #14310, .T. ) ;
#1079=FACE_BOUND ( 'NONE', #21974, .T. ) ;
#1081=VERTEX_POINT ( 'NONE', #21346 ) ;
#1082=EDGE_LOOP ( 'NONE', ( #14610, #10358, #28180, #8654 ) ) ;
#1085=CARTESIAN_POINT ( 'NONE',  ( 18.47091782295028395, -5.000000000000012434, -56.84763970021110424 ) ) ;
#1086=ORIENTED_EDGE ( 'NONE', *, *, #25834, .F. ) ;
#1087=CARTESIAN_POINT ( 'NONE',  ( 161.1922820468853956, -9.999999999999998224, -28.06379628232387802 ) ) ;
#1088=VERTEX_POINT ( 'NONE', #16914 ) ;
#1090=ORIENTED_EDGE ( 'NONE', *, *, #23380, .T. ) ;
#1094=ORIENTED_EDGE ( 'NONE', *, *, #17074, .F. ) ;
#1097=ORIENTED_EDGE ( 'NONE', *, *, #3574, .T. ) ;
#1101=CARTESIAN_POINT ( 'NONE',  ( 168.6922820468853956, -9.999999999999996447, -35.24709285013155835 ) ) ;
#1102=FACE_BOUND ( 'NONE', #26455, .T. ) ;
#1104=LINE ( 'NONE', #24437, #1621 ) ;
#1105=CARTESIAN_POINT ( 'NONE',  ( 132.0152310637605524, -1.999999999999981348, -0.06116980274991495881 ) ) ;
#1106=CARTESIAN_POINT ( 'NONE',  ( 153.6922820468853672, -10.00000000000000178, -6.413161187712876909 ) ) ;
#1107=LINE ( 'NONE', #19843, #27108 ) ;
#1109=EDGE_CURVE ( 'NONE', #15010, #3555, #29256, .T. ) ;
#1110=CARTESIAN_POINT ( 'NONE',  ( 157.0152310637604671, -10.00000000000000000, 1.702185954127501066 ) ) ;
#1111=CARTESIAN_POINT ( 'NONE',  ( 148.6922820468854525, -10.00000000000000178, -32.39392330124607611 ) ) ;
#1112=EDGE_LOOP ( 'NONE', ( #26693, #23174, #25311, #28389 ) ) ;
#1114=VERTEX_POINT ( 'NONE', #16770 ) ;
#1115=VECTOR ( 'NONE', #2153, 1000.000000000000000 ) ;
#1120=EDGE_LOOP ( 'NONE', ( #11525, #6792, #20761, #8444 ) ) ;
#1122=ORIENTED_EDGE ( 'NONE', *, *, #9629, .T. ) ;
#1126=CARTESIAN_POINT ( 'NONE',  ( 163.6922820468853956, -4.999999999999973355, -35.24709285013155835 ) ) ;
#1127=VECTOR ( 'NONE', #896, 1000.000000000000000 ) ;
#1130=DIRECTION ( 'NONE',  ( -2.698458740408365879E-16, 1.000000000000000000, 0.000000000000000000 ) ) ;
#1134=ADVANCED_FACE ( 'NONE', ( #23801 ), #21499, .T. ) ;
#1135=EDGE_CURVE ( 'NONE', #14797, #15637, #8052, .T. ) ;
#1136=CARTESIAN_POINT ( 'NONE',  ( 161.1922820468853672, -9.999999999999998224, -19.40354224447947828 ) ) ;
#1137=DIRECTION ( 'NONE',  ( 1.000000000000000000, 2.698458740408365879E-16, 0.000000000000000000 ) ) ;
#1141=AXIS2_PLACEMENT_3D ( 'NONE', #20849, #9242, #6980 ) ;
#1145=ORIENTED_EDGE ( 'NONE', *, *, #2863, .T. ) ;
#1146=CARTESIAN_POINT ( 'NONE',  ( 125.7287565553229456, -4.000000000000003553, 0.5000000000000143219 ) ) ;
#1147=CARTESIAN_POINT ( 'NONE',  ( 133.6922820468854241, -10.00000000000000711, -0.6060766987539614181 ) ) ;
#1149=DIRECTION ( 'NONE',  ( -2.698458740408365879E-16, 1.000000000000000000, 0.000000000000000000 ) ) ;
#1150=CARTESIAN_POINT ( 'NONE',  ( 175.7287565553229456, -9.999999999999994671, -28.21440484423853690 ) ) ;
#1151=CARTESIAN_POINT ( 'NONE',  ( 174.7287565553228319, -1.999999999999970024, 0.8205080756887930260 ) ) ;
#1153=ORIENTED_EDGE ( 'NONE', *, *, #17753, .F. ) ;
#1154=ORIENTED_EDGE ( 'NONE', *, *, #23808, .T. ) ;
#1155=CARTESIAN_POINT ( 'NONE',  ( 139.5152310637606092, -1.999999999999978684, -28.60870317832789311 ) ) ;
#1158=CARTESIAN_POINT ( 'NONE',  ( 132.0152310637605524, -1.999999999999981348, -34.70218595412750773 ) ) ;
#1160=LINE ( 'NONE', #1616, #29159 ) ;
#1162=ORIENTED_EDGE ( 'NONE', *, *, #30234, .F. ) ;
#1163=CARTESIAN_POINT ( 'NONE',  ( 147.2287565553230309, -1.999999999999976241, -29.49038105676660138 ) ) ;
#1166=VECTOR ( 'NONE', #19580, 1000.000000000000000 ) ;
#1167=ORIENTED_EDGE ( 'NONE', *, *, #26607, .F. ) ;
#1170=CARTESIAN_POINT ( 'NONE',  ( 151.1922820468854525, -1.999999999999974909, -28.06379628232387802 ) ) ;
#1171=ADVANCED_FACE ( 'NONE', ( #19504 ), #21952, .T. ) ;
#1173=ADVANCED_FACE ( 'NONE', ( #24550 ), #12478, .T. ) ;
#1174=DIRECTION ( 'NONE',  ( 0.3090169943749472292, 8.338696094057992503E-17, -0.9510565162951536422 ) ) ;
#1177=CARTESIAN_POINT ( 'NONE',  ( 143.6922820468854525, -4.999999999999978684, -35.24709285013155835 ) ) ;
#1178=DIRECTION ( 'NONE',  ( 0.5877852522924731371, 1.586114251531760728E-16, 0.8090169943749474513 ) ) ;
#1188=CARTESIAN_POINT ( 'NONE',  ( 174.5152310637604103, -1.999999999999969580, -13.05155085951651195 ) ) ;
#1189=EDGE_LOOP ( 'NONE', ( #30137, #13203, #16635, #25070, #21703 ) ) ;
#1190=CARTESIAN_POINT ( 'NONE',  ( 129.5152310637605524, -10.00000000000000888, -13.05155085951650840 ) ) ;
#1191=CARTESIAN_POINT ( 'NONE',  ( 10.44167955025612926, -5.000000000000015099, 32.13618525228277889 ) ) ;
#1192=DIRECTION ( 'NONE',  ( -2.698458740408365879E-16, 1.000000000000000000, 0.000000000000000000 ) ) ;
#1193=EDGE_LOOP ( 'NONE', ( #18358, #3083, #23610, #782 ) ) ;
#1194=VERTEX_POINT ( 'NONE', #21803 ) ;
#1195=ORIENTED_EDGE ( 'NONE', *, *, #86, .T. ) ;
#1197=ORIENTED_EDGE ( 'NONE', *, *, #25697, .T. ) ;
#1200=CARTESIAN_POINT ( 'NONE',  ( 138.6922820468854525, -1.999999999999979572, -26.58683881228715506 ) ) ;
#1201=CARTESIAN_POINT ( 'NONE',  ( 138.6922820468854525, -4.999999999999980460, -9.266330736598359152 ) ) ;
#1202=DIRECTION ( 'NONE',  ( 0.3090169943749472292, 8.338696094057992503E-17, -0.9510565162951536422 ) ) ;
#1203=EDGE_CURVE ( 'NONE', #20918, #28729, #900, .T. ) ;
#1204=ADVANCED_FACE ( 'NONE', ( #14760 ), #29330, .T. ) ;
#1205=AXIS2_PLACEMENT_3D ( 'NONE', #17330, #24367, #28843 ) ;
#1206=ORIENTED_EDGE ( 'NONE', *, *, #21520, .T. ) ;
#1208=DIRECTION ( 'NONE',  ( 0.9510565162951536422, 2.566386769018988816E-16, 0.3090169943749472292 ) ) ;
#1210=CARTESIAN_POINT ( 'NONE',  ( 168.6922820468853388, -1.999999999999971356, -15.07341522555727664 ) ) ;
#1211=CARTESIAN_POINT ( 'NONE',  ( 131.1922820468854241, -10.00000000000000888, -2.083034168790677043 ) ) ;
#1214=ORIENTED_EDGE ( 'NONE', *, *, #194, .T. ) ;
#1218=FACE_BOUND ( 'NONE', #105, .T. ) ;
#1219=EDGE_LOOP ( 'NONE', ( #14532, #205, #5357, #26295 ) ) ;
#1220=PLANE ( 'NONE',  #21848 ) ;
#1221=VECTOR ( 'NONE', #25377, 1000.000000000000000 ) ;
#1223=DIRECTION ( 'NONE',  ( 0.5877852522924731371, 1.586114251531760728E-16, 0.8090169943749474513 ) ) ;
#1224=ORIENTED_EDGE ( 'NONE', *, *, #18694, .F. ) ;
#1225=ORIENTED_EDGE ( 'NONE', *, *, #29517, .T. ) ;
#1226=DIRECTION ( 'NONE',  ( -2.698458740408365879E-16, 1.000000000000000000, 0.000000000000000000 ) ) ;
#1229=EDGE_LOOP ( 'NONE', ( #14138, #4239, #19331, #10820, #23032 ) ) ;
#1232=ORIENTED_EDGE ( 'NONE', *, *, #25979, .F. ) ;
#1234=ORIENTED_EDGE ( 'NONE', *, *, #23247, .T. ) ;
#1237=VECTOR ( 'NONE', #26071, 1000.000000000000000 ) ;
#1240=EDGE_CURVE ( 'NONE', #9967, #24305, #740, .T. ) ;
#1241=CARTESIAN_POINT ( 'NONE',  ( 144.5152310637605240, -10.00000000000000355, -4.391296821672111328 ) ) ;
#1242=EDGE_CURVE ( 'NONE', #20723, #18076, #17360, .T. ) ;
#1243=CARTESIAN_POINT ( 'NONE',  ( 162.0152310637605240, -9.999999999999998224, -24.27857615940569502 ) ) ;
#1244=VECTOR ( 'NONE', #10046, 1000.000000000000000 ) ;
#1245=DIRECTION ( 'NONE',  ( -2.698458740408365879E-16, 1.000000000000000000, 0.000000000000000000 ) ) ;
#1247=LINE ( 'NONE', #10385, #19941 ) ;
#1248=CARTESIAN_POINT ( 'NONE',  ( 161.1922820468853104, -10.00000000000000000, -4.936203717676158398 ) ) ;
#1250=CARTESIAN_POINT ( 'NONE',  ( 143.6922820468854525, -4.999999999999978684, -32.39392330124607611 ) ) ;
#1254=EDGE_LOOP ( 'NONE', ( #813, #8774, #21079, #1162 ) ) ;
#1256=ORIENTED_EDGE ( 'NONE', *, *, #10863, .F. ) ;
#1257=AXIS2_PLACEMENT_3D ( 'NONE', #13555, #9262, #9415 ) ;
#1259=DIRECTION ( 'NONE',  ( 0.5877852522924731371, 1.586114251531760728E-16, 0.8090169943749474513 ) ) ;
#1260=CARTESIAN_POINT ( 'NONE',  ( 167.2287565553228887, -9.999999999999998224, -3.509618943233403510 ) ) ;
#1261=ORIENTED_EDGE ( 'NONE', *, *, #2384, .T. ) ;
#1262=ORIENTED_EDGE ( 'NONE', *, *, #18176, .T. ) ;
#1263=CARTESIAN_POINT ( 'NONE',  ( 130.7287565553229172, -4.999999999999983125, -4.785595155761463104 ) ) ;
#1264=ORIENTED_EDGE ( 'NONE', *, *, #29614, .F. ) ;
#1266=VECTOR ( 'NONE', #954, 1000.000000000000000 ) ;
#1269=ORIENTED_EDGE ( 'NONE', *, *, #25835, .F. ) ;
#1270=ORIENTED_EDGE ( 'NONE', *, *, #7022, .T. ) ;
#1271=LINE ( 'NONE', #10560, #11580 ) ;
#1273=CARTESIAN_POINT ( 'NONE',  ( 151.1922820468854525, -10.00000000000000178, -30.91696583120936026 ) ) ;
#1277=EDGE_CURVE ( 'NONE', #21320, #24253, #5934, .T. ) ;
#1279=ORIENTED_EDGE ( 'NONE', *, *, #13693, .T. ) ;
#1280=ORIENTED_EDGE ( 'NONE', *, *, #28806, .T. ) ;
#1282=CARTESIAN_POINT ( 'NONE',  ( 153.6922820468853672, -1.999999999999975797, -9.266330736598359152 ) ) ;
#1283=VECTOR ( 'NONE', #27792, 1000.000000000000000 ) ;
#1284=CARTESIAN_POINT ( 'NONE',  ( 167.0152310637605240, -4.999999999999972466, -24.27857615940569502 ) ) ;
#1285=DIRECTION ( 'NONE',  ( 0.5877852522924731371, 1.586114251531760728E-16, 0.8090169943749474513 ) ) ;
#1286=LINE ( 'NONE', #10577, #5814 ) ;
#1288=CARTESIAN_POINT ( 'NONE',  ( 142.0152310637606092, -4.999999999999979572, -24.27857615940569147 ) ) ;
#1294=DIRECTION ( 'NONE',  ( -0.8090169943749474513, -2.183098979609982436E-16, 0.5877852522924731371 ) ) ;
#1296=DIRECTION ( 'NONE',  ( 0.9510565162951535312, 2.566386769018988816E-16, -0.3090169943749475623 ) ) ;
#1300=ORIENTED_EDGE ( 'NONE', *, *, #3032, .F. ) ;
#1302=CARTESIAN_POINT ( 'NONE',  ( 148.6922820468854525, -4.999999999999977796, -32.39392330124607611 ) ) ;
#1307=DIRECTION ( 'NONE',  ( 0.9510565162951535312, 2.566386769018988816E-16, -0.3090169943749475623 ) ) ;
#1310=DIRECTION ( 'NONE',  ( -2.698458740408365879E-16, 1.000000000000000000, 0.000000000000000000 ) ) ;
#1312=ORIENTED_EDGE ( 'NONE', *, *, #16099, .F. ) ;
#1313=CARTESIAN_POINT ( 'NONE',  ( 166.1922820468853672, -4.999999999999973355, -30.91696583120936026 ) ) ;
#1315=VECTOR ( 'NONE', #24304, 1000.000000000000000 ) ;
#1317=VECTOR ( 'NONE', #2050, 1000.000000000000000 ) ;
#1319=ORIENTED_EDGE ( 'NONE', *, *, #27218, .F. ) ;
#1321=DIRECTION ( 'NONE',  ( 0.5877852522924731371, 0.000000000000000000, 0.8090169943749474513 ) ) ;
#1322=PLANE ( 'NONE',  #24864 ) ;
#1323=CARTESIAN_POINT ( 'NONE',  ( 153.6922820468853672, -1.999999999999975797, -6.413161187712877798 ) ) ;
#1324=CARTESIAN_POINT ( 'NONE',  ( 158.6922820468853388, -10.00000000000000000, -6.413161187712876909 ) ) ;
#1326=CARTESIAN_POINT ( 'NONE',  ( 154.5152310637604671, -10.00000000000000178, -4.391296821672111328 ) ) ;
#1330=CARTESIAN_POINT ( 'NONE',  ( 169.5152310637604103, -1.999999999999971356, -4.391296821672111328 ) ) ;
#1333=VECTOR ( 'NONE', #15989, 1000.000000000000000 ) ;
#1335=FACE_OUTER_BOUND ( 'NONE', #23321, .T. ) ;
#1341=ORIENTED_EDGE ( 'NONE', *, *, #24841, .T. ) ;
#1342=ADVANCED_FACE ( 'NONE', ( #19799 ), #12325, .T. ) ;
#1343=EDGE_LOOP ( 'NONE', ( #9182, #27199, #3969, #12528, #1225 ) ) ;
#1345=DIRECTION ( 'NONE',  ( -0.9510565162951536422, -2.566386769018988816E-16, -0.3090169943749472292 ) ) ;
#1346=EDGE_CURVE ( 'NONE', #13830, #17432, #3201, .T. ) ;
#1347=LINE ( 'NONE', #5613, #2489 ) ;
#1348=ORIENTED_EDGE ( 'NONE', *, *, #20074, .F. ) ;
#1350=ORIENTED_EDGE ( 'NONE', *, *, #7117, .F. ) ;
#1353=AXIS2_PLACEMENT_3D ( 'NONE', #29693, #27677, #13439 ) ;
#1354=FACE_OUTER_BOUND ( 'NONE', #2002, .T. ) ;
#1355=CARTESIAN_POINT ( 'NONE',  ( 101.7267641804769056, -4.999999999999989342, -73.90882041348888265 ) ) ;
#1356=LINE ( 'NONE', #19643, #3062 ) ;
#1358=EDGE_LOOP ( 'NONE', ( #8368, #24068, #2089, #226 ) ) ;
#1359=CARTESIAN_POINT ( 'NONE',  ( 143.6922820468854525, -4.999999999999978684, -15.07341522555727664 ) ) ;
#1361=CARTESIAN_POINT ( 'NONE',  ( 152.0152310637605808, -10.00000000000000000, -24.27857615940569502 ) ) ;
#1363=LINE ( 'NONE', #8657, #3133 ) ;
#1366=VERTEX_POINT ( 'NONE', #1668 ) ;
#1369=VECTOR ( 'NONE', #21068, 1000.000000000000000 ) ;
#1372=FACE_BOUND ( 'NONE', #2319, .T. ) ;
#1373=EDGE_CURVE ( 'NONE', #26457, #18739, #13247, .T. ) ;
#1375=DIRECTION ( 'NONE',  ( -0.9510565162951536422, -2.566386769018988323E-16, 0.3090169943749475623 ) ) ;
#1376=EDGE_CURVE ( 'NONE', #20136, #19188, #29491, .T. ) ;
#1378=DIRECTION ( 'NONE',  ( 1.110223024625156540E-16, 2.995891024602366092E-32, 1.000000000000000000 ) ) ;
#1379=EDGE_CURVE ( 'NONE', #9909, #26420, #29640, .T. ) ;
#1380=ORIENTED_EDGE ( 'NONE', *, *, #6468, .F. ) ;
#1381=ORIENTED_EDGE ( 'NONE', *, *, #25320, .T. ) ;
#1382=CARTESIAN_POINT ( 'NONE',  ( 139.5152310637605808, -10.00000000000000533, -21.71180489736090991 ) ) ;
#1383=ORIENTED_EDGE ( 'NONE', *, *, #3958, .F. ) ;
#1385=ORIENTED_EDGE ( 'NONE', *, *, #24357, .T. ) ;
#1388=ORIENTED_EDGE ( 'NONE', *, *, #13725, .F. ) ;
#1389=DIRECTION ( 'NONE',  ( -0.5877852522924731371, -1.586114251531760728E-16, -0.8090169943749474513 ) ) ;
#1390=ORIENTED_EDGE ( 'NONE', *, *, #27011, .F. ) ;
#1391=FACE_OUTER_BOUND ( 'NONE', #22443, .T. ) ;
#1394=LINE ( 'NONE', #11136, #2747 ) ;
#1395=FACE_BOUND ( 'NONE', #5957, .T. ) ;
#1396=VECTOR ( 'NONE', #22128, 1000.000000000000000 ) ;
#1397=VERTEX_POINT ( 'NONE', #18266 ) ;
#1399=PLANE ( 'NONE',  #23067 ) ;
#1403=VERTEX_POINT ( 'NONE', #27621 ) ;
#1404=LINE ( 'NONE', #24903, #16830 ) ;
#1407=VERTEX_POINT ( 'NONE', #11252 ) ;
#1409=VERTEX_POINT ( 'NONE', #4241 ) ;
#1412=PLANE ( 'NONE',  #7355 ) ;
#1415=EDGE_CURVE ( 'NONE', #24408, #23323, #4094, .T. ) ;
#1417=EDGE_CURVE ( 'NONE', #18587, #23159, #20697, .T. ) ;
#1418=ORIENTED_EDGE ( 'NONE', *, *, #6948, .T. ) ;
#1420=VECTOR ( 'NONE', #541, 1000.000000000000000 ) ;
#1423=ORIENTED_EDGE ( 'NONE', *, *, #28318, .F. ) ;
#1425=DIRECTION ( 'NONE',  ( -0.5877852522924731371, -1.586114251531760235E-16, 0.8090169943749474513 ) ) ;
#1426=ORIENTED_EDGE ( 'NONE', *, *, #17039, .T. ) ;
#1427=VECTOR ( 'NONE', #29243, 999.9999999999998863 ) ;
#1428=PLANE ( 'NONE',  #29908 ) ;
#1431=ORIENTED_EDGE ( 'NONE', *, *, #20132, .F. ) ;
#1435=DIRECTION ( 'NONE',  ( -2.698458740408365879E-16, 1.000000000000000000, 0.000000000000000000 ) ) ;
#1436=LINE ( 'NONE', #17593, #25213 ) ;
#1437=VECTOR ( 'NONE', #500, 1000.000000000000000 ) ;
#1439=DIRECTION ( 'NONE',  ( 0.5877852522924731371, 1.586114251531760728E-16, 0.8090169943749474513 ) ) ;
#1442=AXIS2_PLACEMENT_3D ( 'NONE', #27922, #25750, #6981 ) ;
#1446=DIRECTION ( 'NONE',  ( -1.110223024625156540E-16, 0.000000000000000000, -1.000000000000000000 ) ) ;
#1448=EDGE_LOOP ( 'NONE', ( #28288, #1390, #21032, #9698 ) ) ;
#1449=DIRECTION ( 'NONE',  ( -1.110223024625156540E-16, 0.000000000000000000, -1.000000000000000000 ) ) ;
#1450=EDGE_CURVE ( 'NONE', #2343, #15349, #27174, .T. ) ;
#1451=DIRECTION ( 'NONE',  ( 0.3090169943749475623, 8.338696094058001131E-17, 0.9510565162951536422 ) ) ;
#1452=DIRECTION ( 'NONE',  ( -2.698458740408365879E-16, 1.000000000000000000, 0.000000000000000000 ) ) ;
#1456=EDGE_LOOP ( 'NONE', ( #22399, #8781, #21563, #9519 ) ) ;
#1457=DIRECTION ( 'NONE',  ( -0.8090169943749474513, -2.183098979609982436E-16, -0.5877852522924731371 ) ) ;
#1458=EDGE_CURVE ( 'NONE', #28897, #29710, #30085, .T. ) ;
#1461=DIRECTION ( 'NONE',  ( 1.110223024625156540E-16, 2.995891024602366092E-32, 1.000000000000000000 ) ) ;
#1463=CARTESIAN_POINT ( 'NONE',  ( 132.0152310637605524, -4.999999999999982236, -1.465663491281971624E-14 ) ) ;
#1465=ORIENTED_EDGE ( 'NONE', *, *, #3746, .T. ) ;
#1470=VECTOR ( 'NONE', #4280, 1000.000000000000000 ) ;
#1471=VECTOR ( 'NONE', #20519, 1000.000000000000000 ) ;
#1472=EDGE_LOOP ( 'NONE', ( #27548, #7434, #25385, #2470 ) ) ;
#1474=DIRECTION ( 'NONE',  ( 0.3090169943749475623, 8.338696094058001131E-17, 0.9510565162951536422 ) ) ;
#1475=EDGE_LOOP ( 'NONE', ( #18969, #23899, #5441, #13330, #15759 ) ) ;
#1476=ORIENTED_EDGE ( 'NONE', *, *, #11789, .T. ) ;
#1478=FACE_OUTER_BOUND ( 'NONE', #12827, .T. ) ;
#1480=DIRECTION ( 'NONE',  ( 0.9510565162951536422, 0.000000000000000000, -0.3090169943749475623 ) ) ;
#1481=DIRECTION ( 'NONE',  ( 0.5877852522924731371, 1.586114251531760728E-16, -0.8090169943749474513 ) ) ;
#1485=DIRECTION ( 'NONE',  ( 0.5877852522924731371, 1.586114251531760728E-16, -0.8090169943749474513 ) ) ;
#1487=VECTOR ( 'NONE', #6963, 1000.000000000000000 ) ;
#1488=FACE_OUTER_BOUND ( 'NONE', #26207, .T. ) ;
#1490=VECTOR ( 'NONE', #16844, 1000.000000000000000 ) ;
#1491=CARTESIAN_POINT ( 'NONE',  ( 149.7287565553230309, -1.999999999999975353, -25.16025403784440329 ) ) ;
#1492=CARTESIAN_POINT ( 'NONE',  ( 7.817546131999246306, -5.000000000000015987, 24.05993303156214935 ) ) ;
#1494=LINE ( 'NONE', #10782, #14605 ) ;
#1495=LINE ( 'NONE', #24378, #14460 ) ;
#1497=EDGE_LOOP ( 'NONE', ( #806, #13423, #22171, #19869 ) ) ;
#1498=CARTESIAN_POINT ( 'NONE',  ( 169.5152310637604387, -1.999999999999971356, -2.627941064794695691 ) ) ;
#1499=CARTESIAN_POINT ( 'NONE',  ( 156.1922820468854241, -4.999999999999975131, -30.91696583120936026 ) ) ;
#1507=AXIS2_PLACEMENT_3D ( 'NONE', #14519, #26299, #14367 ) ;
#1509=LINE ( 'NONE', #27327, #12596 ) ;
#1510=DIRECTION ( 'NONE',  ( 0.5877852522924731371, 0.000000000000000000, 0.8090169943749474513 ) ) ;
#1513=ORIENTED_EDGE ( 'NONE', *, *, #29997, .T. ) ;
#1515=EDGE_CURVE ( 'NONE', #16280, #12464, #8946, .T. ) ;
#1517=ADVANCED_FACE ( 'NONE', ( #19026 ), #13971, .T. ) ;
#1520=CARTESIAN_POINT ( 'NONE',  ( 148.6922820468854525, -4.999999999999977796, -35.24709285013155835 ) ) ;
#1521=EDGE_LOOP ( 'NONE', ( #9352, #12123, #6100, #25034, #22361 ) ) ;
#1524=ORIENTED_EDGE ( 'NONE', *, *, #16902, .T. ) ;
#1527=ORIENTED_EDGE ( 'NONE', *, *, #18894, .T. ) ;
#1530=FACE_BOUND ( 'NONE', #1675, .T. ) ;
#1532=ORIENTED_EDGE ( 'NONE', *, *, #22031, .F. ) ;
#1533=FACE_OUTER_BOUND ( 'NONE', #8235, .T. ) ;
#1536=CARTESIAN_POINT ( 'NONE',  ( 129.5152310637605524, -10.00000000000000888, -21.71180489736090991 ) ) ;
#1537=ORIENTED_EDGE ( 'NONE', *, *, #14272, .F. ) ;
#1542=CARTESIAN_POINT ( 'NONE',  ( 137.2287565553230309, -10.00000000000000533, -3.509618943233403510 ) ) ;
#1543=ORIENTED_EDGE ( 'NONE', *, *, #3915, .F. ) ;
#1544=DIRECTION ( 'NONE',  ( -0.9510565162951536422, -2.566386769018988323E-16, 0.3090169943749475623 ) ) ;
#1546=VECTOR ( 'NONE', #15312, 1000.000000000000000 ) ;
#1548=DIRECTION ( 'NONE',  ( 0.3090169943749475623, 8.338696094058001131E-17, 0.9510565162951536422 ) ) ;
#1550=CARTESIAN_POINT ( 'NONE',  ( 133.6922820468854241, -10.00000000000000711, -32.39392330124607611 ) ) ;
#1551=ADVANCED_FACE ( 'NONE', ( #25908 ), #267, .T. ) ;
#1553=EDGE_CURVE ( 'NONE', #17394, #5801, #23609, .T. ) ;
#1554=VERTEX_POINT ( 'NONE', #21009 ) ;
#1555=DIRECTION ( 'NONE',  ( -2.698458740408365879E-16, 1.000000000000000000, 0.000000000000000000 ) ) ;
#1557=DIRECTION ( 'NONE',  ( -0.9510565162951536422, -2.566386769018988323E-16, 0.3090169943749475623 ) ) ;
#1558=VERTEX_POINT ( 'NONE', #115 ) ;
#1559=VERTEX_POINT ( 'NONE', #11990 ) ;
#1560=CARTESIAN_POINT ( 'NONE',  ( 142.2287565553230309, -10.00000000000000533, -20.83012701892220164 ) ) ;
#1563=ORIENTED_EDGE ( 'NONE', *, *, #29487, .F. ) ;
#1566=CARTESIAN_POINT ( 'NONE',  ( 147.0152310637605808, -4.999999999999977796, -1.632196944975745421E-14 ) ) ;
#1567=CARTESIAN_POINT ( 'NONE',  ( 159.5152310637605240, -4.999999999999974243, -1.770974823053889357E-14 ) ) ;
#1568=ORIENTED_EDGE ( 'NONE', *, *, #25832, .F. ) ;
#1569=CARTESIAN_POINT ( 'NONE',  ( 171.1922820468853672, -9.999999999999994671, -28.06379628232387802 ) ) ;
#1570=EDGE_LOOP ( 'NONE', ( #4552, #9961, #24216, #10666 ) ) ;
#1574=ORIENTED_EDGE ( 'NONE', *, *, #24026, .F. ) ;
#1576=VECTOR ( 'NONE', #20176, 1000.000000000000000 ) ;
#1577=ORIENTED_EDGE ( 'NONE', *, *, #23516, .F. ) ;
#1578=CARTESIAN_POINT ( 'NONE',  ( 175.7287565553229456, -4.999999999999970690, 3.500000000000003109 ) ) ;
#1579=FACE_OUTER_BOUND ( 'NONE', #11118, .T. ) ;
#1580=CARTESIAN_POINT ( 'NONE',  ( 157.0152310637605524, -1.999999999999973133, -34.70218595412750773 ) ) ;
#1584=AXIS2_PLACEMENT_3D ( 'NONE', #13450, #6749, #9158 ) ;
#1585=ORIENTED_EDGE ( 'NONE', *, *, #27651, .F. ) ;
#1587=EDGE_CURVE ( 'NONE', #4687, #30106, #5136, .T. ) ;
#1588=CARTESIAN_POINT ( 'NONE',  ( 172.0152310637604955, -4.999999999999970690, -1.909752701132033609E-14 ) ) ;
#1589=EDGE_CURVE ( 'NONE', #633, #15422, #14131, .T. ) ;
#1590=EDGE_CURVE ( 'NONE', #2176, #22297, #21310, .T. ) ;
#1591=LINE ( 'NONE', #26788, #10873 ) ;
#1592=DIRECTION ( 'NONE',  ( 0.5877852522924731371, 0.000000000000000000, 0.8090169943749474513 ) ) ;
#1593=LINE ( 'NONE', #17594, #22869 ) ;
#1594=AXIS2_PLACEMENT_3D ( 'NONE', #24585, #19543, #12977 ) ;
#1595=DIRECTION ( 'NONE',  ( -2.698458740408365879E-16, 1.000000000000000000, 0.000000000000000000 ) ) ;
#1600=ORIENTED_EDGE ( 'NONE', *, *, #8987, .F. ) ;
#1602=FACE_OUTER_BOUND ( 'NONE', #25544, .T. ) ;
#1605=VECTOR ( 'NONE', #1061, 1000.000000000000000 ) ;
#1606=DIRECTION ( 'NONE',  ( 0.5877852522924731371, 0.000000000000000000, 0.8090169943749474513 ) ) ;
#1608=CARTESIAN_POINT ( 'NONE',  ( 172.0152310637604387, -1.999999999999970468, -6.958068083716895558 ) ) ;
#1611=FACE_OUTER_BOUND ( 'NONE', #1958, .T. ) ;
#1616=CARTESIAN_POINT ( 'NONE',  ( 134.5152310637605808, -10.00000000000000533, -2.627941064794695691 ) ) ;
#1618=ORIENTED_EDGE ( 'NONE', *, *, #23668, .T. ) ;
#1621=VECTOR ( 'NONE', #1245, 1000.000000000000000 ) ;
#1623=VERTEX_POINT ( 'NONE', #11844 ) ;
#1624=ORIENTED_EDGE ( 'NONE', *, *, #12930, .T. ) ;
#1626=ADVANCED_FACE ( 'NONE', ( #28073 ), #2866, .T. ) ;
#1627=VECTOR ( 'NONE', #13245, 1000.000000000000000 ) ;
#1629=DIRECTION ( 'NONE',  ( -0.9510565162951536422, -2.566386769018988816E-16, -0.3090169943749472292 ) ) ;
#1631=CARTESIAN_POINT ( 'NONE',  ( 142.0152310637605808, -4.999999999999979572, -26.04193191628310800 ) ) ;
#1632=LINE ( 'NONE', #10768, #26740 ) ;
#1633=CARTESIAN_POINT ( 'NONE',  ( 161.1922820468853388, -9.999999999999998224, -10.74328820663507678 ) ) ;
#1638=LINE ( 'NONE', #26993, #5641 ) ;
#1640=LINE ( 'NONE', #10920, #10784 ) ;
#1641=PLANE ( 'NONE',  #21233 ) ;
#1643=CARTESIAN_POINT ( 'NONE',  ( 147.0152310637605240, -1.999999999999977573, 1.702185954127501066 ) ) ;
#1644=ORIENTED_EDGE ( 'NONE', *, *, #5603, .F. ) ;
#1647=VERTEX_POINT ( 'NONE', #7281 ) ;
#1650=CARTESIAN_POINT ( 'NONE',  ( 137.0152310637606092, -1.999999999999979572, -32.93883019725009120 ) ) ;
#1653=ORIENTED_EDGE ( 'NONE', *, *, #21161, .T. ) ;
#1656=EDGE_LOOP ( 'NONE', ( #22291, #16181, #17608, #21411, #15076, #18095 ) ) ;
#1659=CARTESIAN_POINT ( 'NONE',  ( 136.1922820468854241, -10.00000000000000533, -28.06379628232387446 ) ) ;
#1660=CARTESIAN_POINT ( 'NONE',  ( 138.6922820468854241, -10.00000000000000533, 2.247092850131519715 ) ) ;
#1661=EDGE_CURVE ( 'NONE', #22694, #16928, #9245, .T. ) ;
#1662=LINE ( 'NONE', #18415, #5967 ) ;
#1667=EDGE_CURVE ( 'NONE', #9897, #3706, #23152, .T. ) ;
#1668=CARTESIAN_POINT ( 'NONE',  ( 175.7287565553229456, -9.999999999999994671, -13.44584919360591613 ) ) ;
#1669=CARTESIAN_POINT ( 'NONE',  ( 172.0152310637604387, -1.999999999999970024, -17.38167787843871182 ) ) ;
#1670=VECTOR ( 'NONE', #23341, 1000.000000000000000 ) ;
#1673=ORIENTED_EDGE ( 'NONE', *, *, #15719, .T. ) ;
#1675=EDGE_LOOP ( 'NONE', ( #4454, #5179, #6577, #7624, #5321 ) ) ;
#1678=LINE ( 'NONE', #8960, #7786 ) ;
#1681=DIRECTION ( 'NONE',  ( 0.5877852522924731371, 1.586114251531760728E-16, -0.8090169943749474513 ) ) ;
#1682=CARTESIAN_POINT ( 'NONE',  ( 133.7287565553229456, -4.000000000000003553, 0.5000000000000029976 ) ) ;
#1683=DIRECTION ( 'NONE',  ( -2.908569913943826047E-16, 1.000000000000000000, 6.826925868028084813E-18 ) ) ;
#1685=ORIENTED_EDGE ( 'NONE', *, *, #7603, .T. ) ;
#1691=VECTOR ( 'NONE', #10005, 1000.000000000000000 ) ;
#1692=LINE ( 'NONE', #15707, #4010 ) ;
#1694=VECTOR ( 'NONE', #29059, 1000.000000000000000 ) ;
#1696=FACE_OUTER_BOUND ( 'NONE', #24882, .T. ) ;
#1697=ORIENTED_EDGE ( 'NONE', *, *, #3987, .T. ) ;
#1698=DIRECTION ( 'NONE',  ( -2.698458740408365879E-16, 1.000000000000000000, 0.000000000000000000 ) ) ;
#1700=FACE_OUTER_BOUND ( 'NONE', #16788, .T. ) ;
#1701=ORIENTED_EDGE ( 'NONE', *, *, #9372, .F. ) ;
#1702=EDGE_LOOP ( 'NONE', ( #19013, #20985, #21361, #6119 ) ) ;
#1703=LINE ( 'NONE', #9295, #18767 ) ;
#1704=VECTOR ( 'NONE', #23386, 999.9999999999998863 ) ;
#1708=ORIENTED_EDGE ( 'NONE', *, *, #13482, .T. ) ;
#1709=CARTESIAN_POINT ( 'NONE',  ( 154.5152310637605240, -10.00000000000000000, -21.71180489736091346 ) ) ;
#1711=LINE ( 'NONE', #8408, #3955 ) ;
#1712=CARTESIAN_POINT ( 'NONE',  ( 130.7287565553229456, -9.999999999999982236, 3.500000000000003109 ) ) ;
#1713=EDGE_LOOP ( 'NONE', ( #18662, #11561, #14399, #9198 ) ) ;
#1716=ORIENTED_EDGE ( 'NONE', *, *, #30020, .F. ) ;
#1718=ADVANCED_FACE ( 'NONE', ( #17188 ), #24069, .T. ) ;
#1722=ORIENTED_EDGE ( 'NONE', *, *, #27731, .T. ) ;
#1723=EDGE_CURVE ( 'NONE', #26303, #5191, #22214, .T. ) ;
#1724=ORIENTED_EDGE ( 'NONE', *, *, #2251, .F. ) ;
#1725=CARTESIAN_POINT ( 'NONE',  ( 127.7287565553229740, -1.999999999999982681, 0.5000000000000115463 ) ) ;
#1726=CARTESIAN_POINT ( 'NONE',  ( 118.5123031260608286, -4.999999999999985789, -86.10422831294586388 ) ) ;
#1727=CARTESIAN_POINT ( 'NONE',  ( 166.1922820468853672, -1.999999999999971356, -30.91696583120936026 ) ) ;
#1728=ORIENTED_EDGE ( 'NONE', *, *, #12623, .T. ) ;
#1732=VECTOR ( 'NONE', #11918, 1000.000000000000000 ) ;
#1733=ORIENTED_EDGE ( 'NONE', *, *, #15202, .F. ) ;
#1734=LINE ( 'NONE', #20322, #4017 ) ;
#1735=FACE_OUTER_BOUND ( 'NONE', #26670, .T. ) ;
#1737=DIRECTION ( 'NONE',  ( -2.698458740408365879E-16, 1.000000000000000000, 0.000000000000000000 ) ) ;
#1738=LINE ( 'NONE', #20328, #16512 ) ;
#1739=CARTESIAN_POINT ( 'NONE',  ( 84.45309523925811845, -4.999999999999994671, 61.35876531300809944 ) ) ;
#1743=ORIENTED_EDGE ( 'NONE', *, *, #23303, .T. ) ;
#1744=FACE_OUTER_BOUND ( 'NONE', #6476, .T. ) ;
#1746=VERTEX_POINT ( 'NONE', #19762 ) ;
#1748=VECTOR ( 'NONE', #8922, 1000.000000000000000 ) ;
#1749=CARTESIAN_POINT ( 'NONE',  ( 175.7287565553229456, -9.999999999999994671, -22.10610323145030520 ) ) ;
#1750=DIRECTION ( 'NONE',  ( -2.698458740408365879E-16, 1.000000000000000000, 0.000000000000000000 ) ) ;
#1751=CARTESIAN_POINT ( 'NONE',  ( 172.0152310637603819, -1.999999999999970912, -0.06116980274991495881 ) ) ;
#1753=VERTEX_POINT ( 'NONE', #28677 ) ;
#1754=VERTEX_POINT ( 'NONE', #26673 ) ;
#1755=CARTESIAN_POINT ( 'NONE',  ( 174.7287565553228887, -1.999999999999969358, -16.50000000000000355 ) ) ;
#1757=EDGE_CURVE ( 'NONE', #24463, #26115, #12750, .T. ) ;
#1759=CARTESIAN_POINT ( 'NONE',  ( 132.2287565553230024, -4.999999999999982236, -12.16987298107780013 ) ) ;
#1761=EDGE_CURVE ( 'NONE', #1908, #20048, #5901, .T. ) ;
#1765=ADVANCED_FACE ( 'NONE', ( #26366 ), #18502, .T. ) ;
#1767=ORIENTED_EDGE ( 'NONE', *, *, #11879, .T. ) ;
#1768=CARTESIAN_POINT ( 'NONE',  ( 162.0152310637604387, -1.999999999999973577, 1.702185954127501066 ) ) ;
#1769=VECTOR ( 'NONE', #19625, 1000.000000000000000 ) ;
#1773=ORIENTED_EDGE ( 'NONE', *, *, #21581, .T. ) ;
#1774=FACE_OUTER_BOUND ( 'NONE', #29876, .T. ) ;
#1777=CARTESIAN_POINT ( 'NONE',  ( 168.6922820468853956, -4.999999999999971578, -35.24709285013155835 ) ) ;
#1778=LINE ( 'NONE', #1932, #23891 ) ;
#1779=VECTOR ( 'NONE', #26176, 1000.000000000000000 ) ;
#1780=DIRECTION ( 'NONE',  ( 1.110223024625156540E-16, 2.995891024602366092E-32, 1.000000000000000000 ) ) ;
#1781=CARTESIAN_POINT ( 'NONE',  ( 102.9952437281683757, -4.999999999999989342, -74.83042475079173528 ) ) ;
#1786=DIRECTION ( 'NONE',  ( 0.5877852522924731371, 1.586114251531760728E-16, -0.8090169943749474513 ) ) ;
#1788=CARTESIAN_POINT ( 'NONE',  ( 149.7287565553230024, -4.999999999999976907, -16.50000000000000000 ) ) ;
#1789=CARTESIAN_POINT ( 'NONE',  ( 138.6922820468854525, -1.999999999999979572, -35.24709285013155835 ) ) ;
#1793=CARTESIAN_POINT ( 'NONE',  ( 102.3970440912936795, -4.999999999999989342, 74.39580727436489838 ) ) ;
#1795=EDGE_LOOP ( 'NONE', ( #21831, #6319, #22373, #27502 ) ) ;
#1796=VECTOR ( 'NONE', #6285, 1000.000000000000000 ) ;
#1797=CARTESIAN_POINT ( 'NONE',  ( 99.72270124223099685, -4.999999999999990230, -72.45278346005385117 ) ) ;
#1798=DIRECTION ( 'NONE',  ( -2.698458740408365879E-16, 1.000000000000000000, 0.000000000000000000 ) ) ;
#1800=ADVANCED_FACE ( 'NONE', ( #12441 ), #1322, .T. ) ;
#1801=VECTOR ( 'NONE', #14004, 1000.000000000000000 ) ;
#1802=PLANE ( 'NONE',  #16117 ) ;
#1804=EDGE_CURVE ( 'NONE', #8129, #28570, #17479, .T. ) ;
#1805=ORIENTED_EDGE ( 'NONE', *, *, #411, .T. ) ;
#1806=EDGE_CURVE ( 'NONE', #14013, #17474, #10613, .T. ) ;
#1815=VECTOR ( 'NONE', #20958, 1000.000000000000000 ) ;
#1817=CARTESIAN_POINT ( 'NONE',  ( 20.06118759710066968, -5.000000000000012434, -61.74198680378115967 ) ) ;
#1818=CARTESIAN_POINT ( 'NONE',  ( 172.0152310637604387, -9.999999999999994671, -17.38167787843871182 ) ) ;
#1820=VECTOR ( 'NONE', #18891, 1000.000000000000000 ) ;
#1821=CARTESIAN_POINT ( 'NONE',  ( 157.0152310637605524, -9.999999999999998224, -24.27857615940569502 ) ) ;
#1822=AXIS2_PLACEMENT_3D ( 'NONE', #4692, #24755, #24596 ) ;
#1823=CARTESIAN_POINT ( 'NONE',  ( 138.6922820468854525, -1.999999999999979572, -6.413161187712876909 ) ) ;
#1824=DIRECTION ( 'NONE',  ( -2.698458740408365879E-16, 1.000000000000000000, 0.000000000000000000 ) ) ;
#1826=VECTOR ( 'NONE', #28497, 1000.000000000000000 ) ;
#1827=ORIENTED_EDGE ( 'NONE', *, *, #10230, .F. ) ;
#1829=VERTEX_POINT ( 'NONE', #5594 ) ;
#1831=CARTESIAN_POINT ( 'NONE',  ( 172.7287565553229456, -1.999999999999970468, -39.49999999999997158 ) ) ;
#1833=FACE_BOUND ( 'NONE', #13395, .T. ) ;
#1836=CARTESIAN_POINT ( 'NONE',  ( 167.0152310637604955, -1.999999999999971356, -15.61832212156129707 ) ) ;
#1840=CARTESIAN_POINT ( 'NONE',  ( 163.6922820468853672, -9.999999999999998224, -23.73366926340167637 ) ) ;
#1841=ORIENTED_EDGE ( 'NONE', *, *, #2900, .T. ) ;
#1842=ORIENTED_EDGE ( 'NONE', *, *, #27520, .T. ) ;
#1843=VERTEX_POINT ( 'NONE', #5292 ) ;
#1844=ADVANCED_FACE ( 'NONE', ( #18082 ), #13209, .T. ) ;
#1847=EDGE_CURVE ( 'NONE', #1403, #28891, #27443, .T. ) ;
#1849=EDGE_LOOP ( 'NONE', ( #23058, #3665, #6405, #3848 ) ) ;
#1850=VECTOR ( 'NONE', #8309, 1000.000000000000000 ) ;
#1855=DIRECTION ( 'NONE',  ( -2.698458740408365879E-16, 1.000000000000000000, 0.000000000000000000 ) ) ;
#1856=VECTOR ( 'NONE', #11459, 1000.000000000000000 ) ;
#1860=AXIS2_PLACEMENT_3D ( 'NONE', #26887, #14779, #26725 ) ;
#1861=ORIENTED_EDGE ( 'NONE', *, *, #15291, .T. ) ;
#1862=ADVANCED_FACE ( 'NONE', ( #6043 ), #11358, .T. ) ;
#1865=DIRECTION ( 'NONE',  ( 0.5877852522924731371, 0.000000000000000000, 0.8090169943749474513 ) ) ;
#1866=VECTOR ( 'NONE', #5960, 1000.000000000000000 ) ;
#1868=FACE_OUTER_BOUND ( 'NONE', #6254, .T. ) ;
#1872=ORIENTED_EDGE ( 'NONE', *, *, #19852, .F. ) ;
#1873=DIRECTION ( 'NONE',  ( -1.110223024625156540E-16, 0.000000000000000000, -1.000000000000000000 ) ) ;
#1875=LINE ( 'NONE', #13882, #16600 ) ;
#1877=DIRECTION ( 'NONE',  ( -0.8090169943749474513, -2.183098979609982436E-16, 0.5877852522924731371 ) ) ;
#1878=VERTEX_POINT ( 'NONE', #10910 ) ;
#1884=LINE ( 'NONE', #30151, #4283 ) ;
#1885=DIRECTION ( 'NONE',  ( -0.9510565162951536422, -2.566386769018988816E-16, -0.3090169943749472292 ) ) ;
#1890=VERTEX_POINT ( 'NONE', #24976 ) ;
#1891=DIRECTION ( 'NONE',  ( -0.9510565162951536422, -2.566386769018988816E-16, -0.3090169943749472292 ) ) ;
#1892=EDGE_CURVE ( 'NONE', #2137, #10985, #13501, .T. ) ;
#1893=LINE ( 'NONE', #13314, #9588 ) ;
#1895=EDGE_CURVE ( 'NONE', #5625, #4687, #13652, .T. ) ;
#1896=DIRECTION ( 'NONE',  ( -2.698458740408365879E-16, 1.000000000000000000, 0.000000000000000000 ) ) ;
#1897=UNCERTAINTY_MEASURE_WITH_UNIT (LENGTH_MEASURE( 1.000000000000000082E-05 ), #9281, 'distance_accuracy_value', 'NONE');
#1900=EDGE_LOOP ( 'NONE', ( #16044, #14481, #10590, #25713, #21287 ) ) ;
#1901=VECTOR ( 'NONE', #29105, 1000.000000000000000 ) ;
#1902=CARTESIAN_POINT ( 'NONE',  ( 161.1922820468853672, -9.999999999999998224, -22.25671179336496053 ) ) ;
#1903=ORIENTED_EDGE ( 'NONE', *, *, #17786, .F. ) ;
#1906=DIRECTION ( 'NONE',  ( -1.110223024625156540E-16, 0.000000000000000000, -1.000000000000000000 ) ) ;
#1907=CARTESIAN_POINT ( 'NONE',  ( 177.2287565553228603, -1.999999999999968914, -12.16987298107780369 ) ) ;
#1908=VERTEX_POINT ( 'NONE', #1631 ) ;
#1910=ORIENTED_EDGE ( 'NONE', *, *, #374, .F. ) ;
#1911=AXIS2_PLACEMENT_3D ( 'NONE', #5698, #17283, #13004 ) ;
#1913=LINE ( 'NONE', #18061, #14911 ) ;
#1918=DIRECTION ( 'NONE',  ( -0.8090169943749474513, -2.183098979609982436E-16, 0.5877852522924731371 ) ) ;
#1920=ORIENTED_EDGE ( 'NONE', *, *, #3574, .F. ) ;
#1925=EDGE_LOOP ( 'NONE', ( #19693, #19949, #3167, #6636 ) ) ;
#1926=LINE ( 'NONE', #25107, #26864 ) ;
#1927=VECTOR ( 'NONE', #25831, 1000.000000000000000 ) ;
#1930=ADVANCED_FACE ( 'NONE', ( #1478 ), #15938, .T. ) ;
#1931=EDGE_CURVE ( 'NONE', #16946, #18592, #17773, .T. ) ;
#1932=CARTESIAN_POINT ( 'NONE',  ( 154.7287565553230309, -10.00000000000000000, -33.82050807568879947 ) ) ;
#1935=DIRECTION ( 'NONE',  ( -2.698458740408365879E-16, 1.000000000000000000, 0.000000000000000000 ) ) ;
#1944=CARTESIAN_POINT ( 'NONE',  ( 147.0152310637606092, -4.999999999999978684, -32.93883019725009120 ) ) ;
#1946=DIRECTION ( 'NONE',  ( -2.698458740408365879E-16, 1.000000000000000000, 0.000000000000000000 ) ) ;
#1947=ORIENTED_EDGE ( 'NONE', *, *, #27396, .T. ) ;
#1948=LINE ( 'NONE', #22847, #301 ) ;
#1950=ORIENTED_EDGE ( 'NONE', *, *, #16125, .T. ) ;
#1952=LINE ( 'NONE', #1797, #4214 ) ;
#1953=DIRECTION ( 'NONE',  ( -0.9510565162951536422, -2.566386769018988816E-16, -0.3090169943749472292 ) ) ;
#1954=DIRECTION ( 'NONE',  ( -0.5877852522924731371, 0.000000000000000000, 0.8090169943749474513 ) ) ;
#1955=VERTEX_POINT ( 'NONE', #8765 ) ;
#1958=EDGE_LOOP ( 'NONE', ( #9691, #6511, #3022, #19742 ) ) ;
#1961=LINE ( 'NONE', #11243, #13754 ) ;
#1963=VERTEX_POINT ( 'NONE', #15329 ) ;
#1964=LINE ( 'NONE', #4538, #25018 ) ;
#1966=AXIS2_PLACEMENT_3D ( 'NONE', #3469, #17641, #10319 ) ;
#1967=DIRECTION ( 'NONE',  ( -2.698458740408365879E-16, 1.000000000000000000, 0.000000000000000000 ) ) ;
#1969=EDGE_CURVE ( 'NONE', #2119, #17207, #1778, .T. ) ;
#1970=DIRECTION ( 'NONE',  ( -0.9510565162951536422, 0.000000000000000000, -0.3090169943749472292 ) ) ;
#1971=EDGE_CURVE ( 'NONE', #1843, #11751, #20218, .T. ) ;
#1973=AXIS2_PLACEMENT_3D ( 'NONE', #5298, #14430, #4989 ) ;
#1974=VECTOR ( 'NONE', #15489, 1000.000000000000000 ) ;
#1975=EDGE_CURVE ( 'NONE', #22500, #6950, #4205, .T. ) ;
#1976=LINE ( 'NONE', #8950, #16082 ) ;
#1978=ORIENTED_EDGE ( 'NONE', *, *, #5256, .T. ) ;
#1980=ORIENTED_EDGE ( 'NONE', *, *, #3782, .F. ) ;
#1984=LINE ( 'NONE', #11265, #20453 ) ;
#1986=VECTOR ( 'NONE', #25170, 1000.000000000000000 ) ;
#1987=VERTEX_POINT ( 'NONE', #29604 ) ;
#1990=FACE_OUTER_BOUND ( 'NONE', #824, .T. ) ;
#1991=ORIENTED_EDGE ( 'NONE', *, *, #23209, .F. ) ;
#1992=CARTESIAN_POINT ( 'NONE',  ( 131.1922820468854241, -1.999999999999982236, -22.25671179336495697 ) ) ;
#1993=ORIENTED_EDGE ( 'NONE', *, *, #1723, .F. ) ;
#1995=VECTOR ( 'NONE', #18610, 999.9999999999998863 ) ;
#1999=CARTESIAN_POINT ( 'NONE',  ( 20.69654234312579533, -5.000000000000012434, -63.69740764588885185 ) ) ;
#2000=LINE ( 'NONE', #27804, #20081 ) ;
#2002=EDGE_LOOP ( 'NONE', ( #27202, #19220, #18719, #5417 ) ) ;
#2004=VECTOR ( 'NONE', #19632, 1000.000000000000000 ) ;
#2006=AXIS2_PLACEMENT_3D ( 'NONE', #8999, #16029, #4889 ) ;
#2007=EDGE_CURVE ( 'NONE', #26011, #21590, #27297, .T. ) ;
#2008=EDGE_CURVE ( 'NONE', #20426, #28522, #15644, .T. ) ;
#2009=EDGE_CURVE ( 'NONE', #17052, #16407, #4953, .T. ) ;
#2012=LINE ( 'NONE', #16170, #2927 ) ;
#2013=ORIENTED_EDGE ( 'NONE', *, *, #28246, .T. ) ;
#2014=ORIENTED_EDGE ( 'NONE', *, *, #6086, .T. ) ;
#2015=LINE ( 'NONE', #6578, #23655 ) ;
#2019=ORIENTED_EDGE ( 'NONE', *, *, #9336, .F. ) ;
#2023=LINE ( 'NONE', #1567, #14475 ) ;
#2024=ORIENTED_EDGE ( 'NONE', *, *, #20166, .T. ) ;
#2025=VERTEX_POINT ( 'NONE', #2227 ) ;
#2026=LINE ( 'NONE', #18321, #3254 ) ;
#2027=EDGE_LOOP ( 'NONE', ( #13919, #4831, #22546, #26614 ) ) ;
#2029=AXIS2_PLACEMENT_3D ( 'NONE', #4808, #7102, #6807 ) ;
#2031=VECTOR ( 'NONE', #25433, 1000.000000000000000 ) ;
#2034=FACE_OUTER_BOUND ( 'NONE', #1925, .T. ) ;
#2036=ORIENTED_EDGE ( 'NONE', *, *, #28323, .T. ) ;
#2040=VERTEX_POINT ( 'NONE', #16241 ) ;
#2041=DIRECTION ( 'NONE',  ( -0.8090169943749474513, -2.183098979609982436E-16, 0.5877852522924731371 ) ) ;
#2042=EDGE_CURVE ( 'NONE', #26513, #16825, #11500, .T. ) ;
#2044=LINE ( 'NONE', #30010, #16034 ) ;
#2046=DIRECTION ( 'NONE',  ( -0.8090169943749474513, -2.183098979609982436E-16, 0.5877852522924731371 ) ) ;
#2049=ORIENTED_EDGE ( 'NONE', *, *, #7802, .T. ) ;
#2050=DIRECTION ( 'NONE',  ( 0.5877852522924731371, 1.586114251531760728E-16, 0.8090169943749474513 ) ) ;
#2056=ORIENTED_EDGE ( 'NONE', *, *, #7085, .T. ) ;
#2058=ORIENTED_EDGE ( 'NONE', *, *, #23632, .T. ) ;
#2060=LINE ( 'NONE', #30028, #23231 ) ;
#2063=PLANE ( 'NONE',  #16133 ) ;
#2064=ORIENTED_EDGE ( 'NONE', *, *, #21308, .F. ) ;
#2066=CARTESIAN_POINT ( 'NONE',  ( 130.7287565553229172, -10.00000000000000888, -30.76635726929466585 ) ) ;
#2067=VECTOR ( 'NONE', #18751, 1000.000000000000000 ) ;
#2069=ORIENTED_EDGE ( 'NONE', *, *, #4771, .F. ) ;
#2070=DIRECTION ( 'NONE',  ( 0.5877852522924731371, 0.000000000000000000, 0.8090169943749474513 ) ) ;
#2071=EDGE_CURVE ( 'NONE', #23292, #10473, #9039, .T. ) ;
#2072=VECTOR ( 'NONE', #6617, 1000.000000000000000 ) ;
#2076=ORIENTED_EDGE ( 'NONE', *, *, #7497, .T. ) ;
#2077=DIRECTION ( 'NONE',  ( 1.110223024625156540E-16, 2.995891024602366092E-32, 1.000000000000000000 ) ) ;
#2078=AXIS2_PLACEMENT_3D ( 'NONE', #825, #9667, #12260 ) ;
#2079=CARTESIAN_POINT ( 'NONE',  ( 168.6922820468853388, -9.999999999999996447, -17.92658477444275889 ) ) ;
#2080=VERTEX_POINT ( 'NONE', #23574 ) ;
#2082=CARTESIAN_POINT ( 'NONE',  ( 174.5152310637604671, -9.999999999999994671, -19.94844914048349693 ) ) ;
#2083=CARTESIAN_POINT ( 'NONE',  ( 136.1922820468854241, -4.999999999999980460, -10.74328820663507322 ) ) ;
#2084=AXIS2_PLACEMENT_3D ( 'NONE', #2149, #27649, #13273 ) ;
#2085=DIRECTION ( 'NONE',  ( -0.9510565162951536422, -2.566386769018988323E-16, 0.3090169943749475623 ) ) ;
#2089=ORIENTED_EDGE ( 'NONE', *, *, #28976, .F. ) ;
#2092=DIRECTION ( 'NONE',  ( -2.698458740408365879E-16, 1.000000000000000000, 0.000000000000000000 ) ) ;
#2093=LINE ( 'NONE', #22688, #27122 ) ;
#2099=ORIENTED_EDGE ( 'NONE', *, *, #6954, .T. ) ;
#2100=DIRECTION ( 'NONE',  ( -0.9510565162951536422, -2.566386769018988816E-16, -0.3090169943749472292 ) ) ;
#2101=DIRECTION ( 'NONE',  ( -0.5877852522924731371, -1.586114251531760235E-16, 0.8090169943749474513 ) ) ;
#2104=PLANE ( 'NONE',  #4427 ) ;
#2105=ORIENTED_EDGE ( 'NONE', *, *, #1590, .F. ) ;
#2108=EDGE_CURVE ( 'NONE', #28209, #22503, #9210, .T. ) ;
#2113=VECTOR ( 'NONE', #12320, 1000.000000000000000 ) ;
#2114=EDGE_CURVE ( 'NONE', #21937, #14836, #2670, .T. ) ;
#2117=ORIENTED_EDGE ( 'NONE', *, *, #11471, .F. ) ;
#2118=PLANE ( 'NONE',  #24039 ) ;
#2119=VERTEX_POINT ( 'NONE', #16393 ) ;
#2120=CARTESIAN_POINT ( 'NONE',  ( 154.5152310637605524, -1.999999999999974465, -19.94844914048349693 ) ) ;
#2121=VERTEX_POINT ( 'NONE', #13940 ) ;
#2127=ORIENTED_EDGE ( 'NONE', *, *, #24104, .T. ) ;
#2128=AXIS2_PLACEMENT_3D ( 'NONE', #6346, #1174, #15641 ) ;
#2132=DIRECTION ( 'NONE',  ( 0.000000000000000000, 0.000000000000000000, -1.000000000000000000 ) ) ;
#2133=DIRECTION ( 'NONE',  ( -2.698458740408365879E-16, 1.000000000000000000, 0.000000000000000000 ) ) ;
#2134=ORIENTED_EDGE ( 'NONE', *, *, #23845, .F. ) ;
#2135=CARTESIAN_POINT ( 'NONE',  ( 164.7287565553229740, -1.999999999999970912, -33.82050807568879947 ) ) ;
#2137=VERTEX_POINT ( 'NONE', #9056 ) ;
#2139=ORIENTED_EDGE ( 'NONE', *, *, #18688, .T. ) ;
#2141=ADVANCED_FACE ( 'NONE', ( #16705 ), #28194, .T. ) ;
#2148=ADVANCED_FACE ( 'NONE', ( #4647 ), #14089, .T. ) ;
#2149=CARTESIAN_POINT ( 'NONE',  ( 162.2287565553229172, -9.999999999999998224, -12.16987298107780369 ) ) ;
#2152=CARTESIAN_POINT ( 'NONE',  ( 144.7287565553230024, -4.999999999999978684, -7.839745962155614478 ) ) ;
#2153=DIRECTION ( 'NONE',  ( 2.908569913943825554E-16, -1.000000000000000000, 0.000000000000000000 ) ) ;
#2155=CARTESIAN_POINT ( 'NONE',  ( 147.0152310637605240, -4.999999999999977796, 1.702185954127501066 ) ) ;
#2157=ORIENTED_EDGE ( 'NONE', *, *, #18939, .F. ) ;
#2158=ORIENTED_EDGE ( 'NONE', *, *, #5327, .F. ) ;
#2159=DIRECTION ( 'NONE',  ( 1.000000000000000000, 2.891205793294675861E-16, 0.000000000000000000 ) ) ;
#2164=ORIENTED_EDGE ( 'NONE', *, *, #27058, .T. ) ;
#2166=VECTOR ( 'NONE', #19653, 1000.000000000000000 ) ;
#2168=DIRECTION ( 'NONE',  ( -0.9510565162951536422, -2.566386769018988816E-16, -0.3090169943749472292 ) ) ;
#2170=ORIENTED_EDGE ( 'NONE', *, *, #5331, .F. ) ;
#2171=DIRECTION ( 'NONE',  ( -0.9510565162951536422, -2.566386769018988816E-16, -0.3090169943749472292 ) ) ;
#2172=VERTEX_POINT ( 'NONE', #7092 ) ;
#2176=VERTEX_POINT ( 'NONE', #11951 ) ;
#2177=EDGE_CURVE ( 'NONE', #29408, #24657, #2538, .T. ) ;
#2178=EDGE_LOOP ( 'NONE', ( #378, #21895, #3651, #22795, #9995 ) ) ;
#2179=EDGE_CURVE ( 'NONE', #29391, #30115, #11806, .T. ) ;
#2181=ORIENTED_EDGE ( 'NONE', *, *, #3371, .T. ) ;
#2183=ADVANCED_FACE ( 'NONE', ( #18383 ), #27737, .T. ) ;
#2184=CARTESIAN_POINT ( 'NONE',  ( 106.5152396090253148, -4.999999999999988454, 77.38785145663800336 ) ) ;
#2188=ORIENTED_EDGE ( 'NONE', *, *, #2274, .T. ) ;
#2189=PLANE ( 'NONE',  #18642 ) ;
#2190=VECTOR ( 'NONE', #14427, 1000.000000000000000 ) ;
#2191=CARTESIAN_POINT ( 'NONE',  ( 176.1922820468852819, -9.999999999999994671, -13.59645775552055902 ) ) ;
#2192=LINE ( 'NONE', #20772, #16546 ) ;
#2197=ORIENTED_EDGE ( 'NONE', *, *, #18377, .T. ) ;
#2198=DIRECTION ( 'NONE',  ( -1.110223024625156540E-16, 0.000000000000000000, -1.000000000000000000 ) ) ;
#2199=ORIENTED_EDGE ( 'NONE', *, *, #26218, .F. ) ;
#2202=DIRECTION ( 'NONE',  ( -0.9510565162951536422, -2.566386769018988323E-16, 0.3090169943749475623 ) ) ;
#2203=DIRECTION ( 'NONE',  ( -2.698458740408365879E-16, 1.000000000000000000, 0.000000000000000000 ) ) ;
#2205=EDGE_LOOP ( 'NONE', ( #16150, #2209, #7218, #11627 ) ) ;
#2206=VERTEX_POINT ( 'NONE', #14993 ) ;
#2207=DIRECTION ( 'NONE',  ( 6.938893903907227392E-16, -0.000000000000000000, 1.000000000000000000 ) ) ;
#2209=ORIENTED_EDGE ( 'NONE', *, *, #3675, .F. ) ;
#2211=CARTESIAN_POINT ( 'NONE',  ( 132.2287565553230024, -10.00000000000000888, -3.509618943233403510 ) ) ;
#2212=VERTEX_POINT ( 'NONE', #21875 ) ;
#2213=ADVANCED_FACE ( 'NONE', ( #7841 ), #23892, .T. ) ;
#2215=LINE ( 'NONE', #4189, #12522 ) ;
#2217=ORIENTED_EDGE ( 'NONE', *, *, #9890, .T. ) ;
#2220=ORIENTED_EDGE ( 'NONE', *, *, #2042, .T. ) ;
#2224=EDGE_LOOP ( 'NONE', ( #22672, #8764, #8225, #13266 ) ) ;
#2225=CARTESIAN_POINT ( 'NONE',  ( 151.1922820468853672, -1.999999999999976685, -4.936203717676158398 ) ) ;
#2226=DIRECTION ( 'NONE',  ( 0.9510565162951536422, 0.000000000000000000, -0.3090169943749475623 ) ) ;
#2227=CARTESIAN_POINT ( 'NONE',  ( 141.1922820468854525, -1.999999999999979128, -19.40354224447947473 ) ) ;
#2228=DIRECTION ( 'NONE',  ( -0.9510565162951536422, -2.566386769018988323E-16, 0.3090169943749475623 ) ) ;
#2229=DIRECTION ( 'NONE',  ( -0.9510565162951536422, 0.000000000000000000, -0.3090169943749472292 ) ) ;
#2234=EDGE_CURVE ( 'NONE', #26570, #10404, #12407, .T. ) ;
#2235=EDGE_CURVE ( 'NONE', #7797, #18644, #10269, .T. ) ;
#2239=DIRECTION ( 'NONE',  ( 0.9510565162951536422, 0.000000000000000000, -0.3090169943749475623 ) ) ;
#2240=CARTESIAN_POINT ( 'NONE',  ( 141.1922820468854525, -1.999999999999978684, -28.06379628232387446 ) ) ;
#2243=DIRECTION ( 'NONE',  ( -1.000000000000000000, -2.698458740408365879E-16, -0.000000000000000000 ) ) ;
#2245=VECTOR ( 'NONE', #13063, 1000.000000000000000 ) ;
#2246=EDGE_LOOP ( 'NONE', ( #6110, #5836, #1827, #7710 ) ) ;
#2247=CARTESIAN_POINT ( 'NONE',  ( 134.5152310637605808, -4.999999999999981348, -11.28819510263909187 ) ) ;
#2248=CARTESIAN_POINT ( 'NONE',  ( 152.2287565553230309, -1.999999999999974465, -29.49038105676660493 ) ) ;
#2249=AXIS2_PLACEMENT_3D ( 'NONE', #24723, #22430, #8220 ) ;
#2251=EDGE_CURVE ( 'NONE', #17576, #26769, #12711, .T. ) ;
#2252=ORIENTED_EDGE ( 'NONE', *, *, #18555, .T. ) ;
#2259=CARTESIAN_POINT ( 'NONE',  ( 149.5152310637605808, -10.00000000000000178, -30.37205893520531319 ) ) ;
#2261=VECTOR ( 'NONE', #232, 1000.000000000000000 ) ;
#2262=ORIENTED_EDGE ( 'NONE', *, *, #20668, .T. ) ;
#2263=PLANE ( 'NONE',  #1141 ) ;
#2264=DIRECTION ( 'NONE',  ( 0.5877852522924731371, 1.586114251531760728E-16, 0.8090169943749474513 ) ) ;
#2265=ORIENTED_EDGE ( 'NONE', *, *, #24913, .F. ) ;
#2267=CARTESIAN_POINT ( 'NONE',  ( 151.1922820468854525, -10.00000000000000178, -28.06379628232387802 ) ) ;
#2269=CARTESIAN_POINT ( 'NONE',  ( 149.7287565553229456, -10.00000000000000355, 0.8205080756887930260 ) ) ;
#2270=EDGE_CURVE ( 'NONE', #15678, #12642, #26790, .T. ) ;
#2272=VECTOR ( 'NONE', #6813, 1000.000000000000000 ) ;
#2274=EDGE_CURVE ( 'NONE', #16222, #18174, #5710, .T. ) ;
#2275=EDGE_LOOP ( 'NONE', ( #4680, #12647, #21018, #23137 ) ) ;
#2277=PLANE ( 'NONE',  #3934 ) ;
#2278=FACE_OUTER_BOUND ( 'NONE', #25468, .T. ) ;
#2280=CARTESIAN_POINT ( 'NONE',  ( 149.7287565553230309, -10.00000000000000178, -25.16025403784440329 ) ) ;
#2281=DIRECTION ( 'NONE',  ( -0.9510565162951536422, -2.566386769018988816E-16, -0.3090169943749472292 ) ) ;
#2283=CARTESIAN_POINT ( 'NONE',  ( 156.1922820468853956, -1.999999999999975353, -19.40354224447947828 ) ) ;
#2284=DIRECTION ( 'NONE',  ( -1.110223024625156540E-16, 0.000000000000000000, -1.000000000000000000 ) ) ;
#2285=DIRECTION ( 'NONE',  ( -2.908569913943826047E-16, 1.000000000000000000, 6.826925868028084813E-18 ) ) ;
#2286=VERTEX_POINT ( 'NONE', #22033 ) ;
#2291=VECTOR ( 'NONE', #13931, 999.9999999999998863 ) ;
#2292=DIRECTION ( 'NONE',  ( 0.9510565162951536422, 2.566386769018988816E-16, 0.3090169943749472292 ) ) ;
#2293=FACE_OUTER_BOUND ( 'NONE', #25182, .T. ) ;
#2294=PLANE ( 'NONE',  #2084 ) ;
#2295=VECTOR ( 'NONE', #18970, 1000.000000000000000 ) ;
#2298=VERTEX_POINT ( 'NONE', #5254 ) ;
#2299=PRESENTATION_STYLE_ASSIGNMENT (( #2742 ) ) ;
#2301=CARTESIAN_POINT ( 'NONE',  ( 148.6922820468854241, -10.00000000000000178, -17.92658477444275889 ) ) ;
#2303=DIRECTION ( 'NONE',  ( 0.000000000000000000, -0.7071067811865455743, 0.7071067811865495711 ) ) ;
#2306=PLANE ( 'NONE',  #25775 ) ;
#2307=CARTESIAN_POINT ( 'NONE',  ( 154.5152310637604955, -4.999999999999976019, -1.715463671822631215E-14 ) ) ;
#2308=ORIENTED_EDGE ( 'NONE', *, *, #19397, .F. ) ;
#2313=VECTOR ( 'NONE', #10243, 1000.000000000000000 ) ;
#2318=VERTEX_POINT ( 'NONE', #17438 ) ;
#2319=EDGE_LOOP ( 'NONE', ( #16188, #11098, #11207, #23126, #15990 ) ) ;
#2320=AXIS2_PLACEMENT_3D ( 'NONE', #7927, #26569, #26727 ) ;
#2322=DIRECTION ( 'NONE',  ( -0.5877852522924731371, 0.000000000000000000, 0.8090169943749474513 ) ) ;
#2324=CARTESIAN_POINT ( 'NONE',  ( 132.0152310637605808, -1.999999999999981348, -24.27857615940569147 ) ) ;
#2326=ORIENTED_EDGE ( 'NONE', *, *, #27824, .F. ) ;
#2327=EDGE_LOOP ( 'NONE', ( #6846, #6618, #28633, #9427 ) ) ;
#2333=ORIENTED_EDGE ( 'NONE', *, *, #24528, .F. ) ;
#2334=DIRECTION ( 'NONE',  ( -2.698458740408365879E-16, 1.000000000000000000, 0.000000000000000000 ) ) ;
#2339=VECTOR ( 'NONE', #1378, 1000.000000000000000 ) ;
#2340=ORIENTED_EDGE ( 'NONE', *, *, #1847, .T. ) ;
#2343=VERTEX_POINT ( 'NONE', #5409 ) ;
#2344=LINE ( 'NONE', #9016, #6234 ) ;
#2345=CARTESIAN_POINT ( 'NONE',  ( 162.0152310637604671, -4.999999999999974243, -17.38167787843871182 ) ) ;
#2346=EDGE_CURVE ( 'NONE', #22282, #18177, #5862, .T. ) ;
#2347=DIRECTION ( 'NONE',  ( -2.698458740408365879E-16, 1.000000000000000000, 0.000000000000000000 ) ) ;
#2348=EDGE_CURVE ( 'NONE', #28792, #14970, #24475, .T. ) ;
#2349=EDGE_CURVE ( 'NONE', #29672, #2431, #21431, .T. ) ;
#2351=EDGE_CURVE ( 'NONE', #11550, #15239, #24036, .T. ) ;
#2352=CARTESIAN_POINT ( 'NONE',  ( 137.0152310637606092, -1.999999999999979572, -24.27857615940569147 ) ) ;
#2353=ORIENTED_EDGE ( 'NONE', *, *, #483, .F. ) ;
#2354=CARTESIAN_POINT ( 'NONE',  ( 159.5152310637604955, -4.999999999999974243, -21.71180489736091346 ) ) ;
#2355=ORIENTED_EDGE ( 'NONE', *, *, #17783, .T. ) ;
#2357=VECTOR ( 'NONE', #11359, 1000.000000000000000 ) ;
#2359=CARTESIAN_POINT ( 'NONE',  ( 164.5152310637605240, -4.999999999999972466, -28.60870317832789667 ) ) ;
#2362=ORIENTED_EDGE ( 'NONE', *, *, #9665, .T. ) ;
#2363=VERTEX_POINT ( 'NONE', #19429 ) ;
#2366=EDGE_LOOP ( 'NONE', ( #17895, #10638, #12091, #6441 ) ) ;
#2367=VECTOR ( 'NONE', #30002, 1000.000000000000000 ) ;
#2369=DIRECTION ( 'NONE',  ( -0.8090169943749474513, -2.183098979609982436E-16, 0.5877852522924731371 ) ) ;
#2371=VERTEX_POINT ( 'NONE', #28802 ) ;
#2372=FACE_OUTER_BOUND ( 'NONE', #25370, .T. ) ;
#2375=VERTEX_POINT ( 'NONE', #18040 ) ;
#2376=CARTESIAN_POINT ( 'NONE',  ( 8.373952262043122374, -5.000000000000015099, 25.77237501798157737 ) ) ;
#2377=AXIS2_PLACEMENT_3D ( 'NONE', #19077, #24266, #16932 ) ;
#2379=DIRECTION ( 'NONE',  ( 0.3090169943749475623, 8.338696094058001131E-17, 0.9510565162951536422 ) ) ;
#2381=CARTESIAN_POINT ( 'NONE',  ( 2.885073759410454741, -5.000000000000016875, 8.879344012873866987 ) ) ;
#2382=EDGE_CURVE ( 'NONE', #14798, #28792, #12863, .T. ) ;
#2384=EDGE_CURVE ( 'NONE', #18677, #7083, #18191, .T. ) ;
#2386=VECTOR ( 'NONE', #10186, 1000.000000000000000 ) ;
#2392=DIRECTION ( 'NONE',  ( -2.698458740408365879E-16, 1.000000000000000000, 0.000000000000000000 ) ) ;
#2393=DIRECTION ( 'NONE',  ( -0.5877852522924731371, -1.586114251531760235E-16, 0.8090169943749474513 ) ) ;
#2397=DIRECTION ( 'NONE',  ( -2.698458740408365879E-16, 1.000000000000000000, 0.000000000000000000 ) ) ;
#2399=ORIENTED_EDGE ( 'NONE', *, *, #29176, .T. ) ;
#2400=CARTESIAN_POINT ( 'NONE',  ( 168.6922820468852819, -1.999999999999972244, -0.6060766987539614181 ) ) ;
#2403=ORIENTED_EDGE ( 'NONE', *, *, #29649, .F. ) ;
#2405=EDGE_LOOP ( 'NONE', ( #18466, #28383, #2939, #24172 ) ) ;
#2407=VECTOR ( 'NONE', #8647, 1000.000000000000000 ) ;
#2409=EDGE_LOOP ( 'NONE', ( #449, #9178, #16543, #29505 ) ) ;
#2413=EDGE_CURVE ( 'NONE', #28897, #6950, #1436, .T. ) ;
#2414=VECTOR ( 'NONE', #22022, 1000.000000000000000 ) ;
#2415=ORIENTED_EDGE ( 'NONE', *, *, #16103, .T. ) ;
#2416=FACE_OUTER_BOUND ( 'NONE', #535, .T. ) ;
#2418=ORIENTED_EDGE ( 'NONE', *, *, #16387, .T. ) ;
#2419=LINE ( 'NONE', #7283, #13858 ) ;
#2420=EDGE_CURVE ( 'NONE', #4823, #2890, #25228, .T. ) ;
#2421=FACE_OUTER_BOUND ( 'NONE', #19990, .T. ) ;
#2423=VECTOR ( 'NONE', #22294, 1000.000000000000000 ) ;
#2425=FACE_OUTER_BOUND ( 'NONE', #8742, .T. ) ;
#2426=DIRECTION ( 'NONE',  ( -2.698458740408365879E-16, 1.000000000000000000, 0.000000000000000000 ) ) ;
#2430=PLANE ( 'NONE',  #9028 ) ;
#2431=VERTEX_POINT ( 'NONE', #27406 ) ;
#2432=CARTESIAN_POINT ( 'NONE',  ( 153.6922820468853672, -4.999999999999976907, -6.413161187712876909 ) ) ;
#2434=LINE ( 'NONE', #19043, #19038 ) ;
#2435=ORIENTED_EDGE ( 'NONE', *, *, #26498, .T. ) ;
#2436=DIRECTION ( 'NONE',  ( 0.3090169943749472292, 8.338696094057992503E-17, -0.9510565162951536422 ) ) ;
#2437=ORIENTED_EDGE ( 'NONE', *, *, #21004, .T. ) ;
#2441=ORIENTED_EDGE ( 'NONE', *, *, #6056, .T. ) ;
#2443=CARTESIAN_POINT ( 'NONE',  ( 12.35150960650664942, -5.000000000000014211, 38.01403777520749117 ) ) ;
#2444=LINE ( 'NONE', #11721, #17476 ) ;
#2447=EDGE_CURVE ( 'NONE', #11751, #2343, #1893, .T. ) ;
#2452=VECTOR ( 'NONE', #1485, 1000.000000000000000 ) ;
#2456=CARTESIAN_POINT ( 'NONE',  ( 109.1175021841459056, -4.999999999999987566, -79.27850588649985752 ) ) ;
#2457=DIRECTION ( 'NONE',  ( 0.9510565162951536422, 2.566386769018988816E-16, 0.3090169943749472292 ) ) ;
#2461=VERTEX_POINT ( 'NONE', #11174 ) ;
#2463=ORIENTED_EDGE ( 'NONE', *, *, #18246, .F. ) ;
#2464=DIRECTION ( 'NONE',  ( -2.698458740408365879E-16, 1.000000000000000000, 0.000000000000000000 ) ) ;
#2469=ORIENTED_EDGE ( 'NONE', *, *, #17041, .T. ) ;
#2470=ORIENTED_EDGE ( 'NONE', *, *, #3402, .F. ) ;
#2473=CARTESIAN_POINT ( 'NONE',  ( 180.7287565553229456, -9.999999999999968026, -33.50000000000000000 ) ) ;
#2474=VECTOR ( 'NONE', #28033, 1000.000000000000000 ) ;
#2476=FACE_OUTER_BOUND ( 'NONE', #15120, .T. ) ;
#2477=CARTESIAN_POINT ( 'NONE',  ( 17.59495141080627789, -5.000000000000013323, -54.15169229443701937 ) ) ;
#2478=ORIENTED_EDGE ( 'NONE', *, *, #4864, .F. ) ;
#2482=EDGE_LOOP ( 'NONE', ( #907, #19784, #9447, #8535, #27642 ) ) ;
#2485=ORIENTED_EDGE ( 'NONE', *, *, #29448, .F. ) ;
#2486=CARTESIAN_POINT ( 'NONE',  ( 129.5152310637605808, -10.00000000000000888, -28.60870317832789311 ) ) ;
#2487=ORIENTED_EDGE ( 'NONE', *, *, #13895, .T. ) ;
#2489=VECTOR ( 'NONE', #1192, 1000.000000000000000 ) ;
#2491=EDGE_CURVE ( 'NONE', #25406, #23532, #15746, .T. ) ;
#2492=ADVANCED_FACE ( 'NONE', ( #22176 ), #11021, .T. ) ;
#2498=VERTEX_POINT ( 'NONE', #8285 ) ;
#2499=FACE_BOUND ( 'NONE', #5350, .T. ) ;
#2500=VECTOR ( 'NONE', #10038, 1000.000000000000000 ) ;
#2501=LINE ( 'NONE', #23088, #18403 ) ;
#2502=CARTESIAN_POINT ( 'NONE',  ( 164.5152310637604671, -1.999999999999971800, -21.71180489736091346 ) ) ;
#2503=LINE ( 'NONE', #4471, #13383 ) ;
#2506=CARTESIAN_POINT ( 'NONE',  ( 148.6922820468853956, -1.999999999999977129, -6.413161187712876909 ) ) ;
#2508=LINE ( 'NONE', #16812, #28637 ) ;
#2510=AXIS2_PLACEMENT_3D ( 'NONE', #5383, #24154, #3258 ) ;
#2512=ORIENTED_EDGE ( 'NONE', *, *, #3444, .F. ) ;
#2514=LINE ( 'NONE', #18355, #27847 ) ;
#2515=CARTESIAN_POINT ( 'NONE',  ( 132.2287565553230024, -1.999999999999981348, -29.49038105676660138 ) ) ;
#2517=EDGE_LOOP ( 'NONE', ( #10511, #28396, #2117, #6335 ) ) ;
#2520=ORIENTED_EDGE ( 'NONE', *, *, #15928, .F. ) ;
#2523=VERTEX_POINT ( 'NONE', #29715 ) ;
#2524=DIRECTION ( 'NONE',  ( 2.698458740408365879E-16, -1.000000000000000000, 0.000000000000000000 ) ) ;
#2526=EDGE_LOOP ( 'NONE', ( #15705, #23448, #8859, #2157 ) ) ;
#2530=EDGE_CURVE ( 'NONE', #14970, #1987, #4164, .T. ) ;
#2531=ADVANCED_FACE ( 'NONE', ( #22786 ), #24936, .T. ) ;
#2532=ORIENTED_EDGE ( 'NONE', *, *, #12787, .T. ) ;
#2533=ORIENTED_EDGE ( 'NONE', *, *, #4361, .T. ) ;
#2534=VECTOR ( 'NONE', #21135, 1000.000000000000000 ) ;
#2535=DIRECTION ( 'NONE',  ( 1.110223024625156540E-16, 2.995891024602366092E-32, 1.000000000000000000 ) ) ;
#2536=VECTOR ( 'NONE', #26811, 1000.000000000000000 ) ;
#2537=LINE ( 'NONE', #22978, #3109 ) ;
#2538=LINE ( 'NONE', #9669, #15388 ) ;
#2539=LINE ( 'NONE', #26328, #5787 ) ;
#2545=EDGE_LOOP ( 'NONE', ( #28044, #17103, #25529, #13775 ) ) ;
#2546=DIRECTION ( 'NONE',  ( -0.5877852522924731371, -1.586114251531760728E-16, -0.8090169943749474513 ) ) ;
#2548=DIRECTION ( 'NONE',  ( 0.9510565162951536422, 2.566386769018988816E-16, 0.3090169943749472292 ) ) ;
#2549=CARTESIAN_POINT ( 'NONE',  ( 142.0152310637606092, -10.00000000000000355, -15.61832212156129707 ) ) ;
#2552=DIRECTION ( 'NONE',  ( 0.5877852522924731371, 1.586114251531760728E-16, -0.8090169943749474513 ) ) ;
#2555=FACE_OUTER_BOUND ( 'NONE', #11801, .T. ) ;
#2556=DIRECTION ( 'NONE',  ( 0.3090169943749475623, 8.338696094058001131E-17, 0.9510565162951536422 ) ) ;
#2557=EDGE_CURVE ( 'NONE', #4895, #24305, #17735, .T. ) ;
#2560=VERTEX_POINT ( 'NONE', #19881 ) ;
#2564=ADVANCED_FACE ( 'NONE', ( #29245 ), #13018, .T. ) ;
#2565=EDGE_CURVE ( 'NONE', #26900, #9877, #22333, .T. ) ;
#2566=EDGE_CURVE ( 'NONE', #17684, #10350, #6157, .T. ) ;
#2568=VECTOR ( 'NONE', #22284, 1000.000000000000000 ) ;
#2569=VERTEX_POINT ( 'NONE', #9635 ) ;
#2570=CARTESIAN_POINT ( 'NONE',  ( 154.5152310637604955, -1.999999999999975353, -2.627941064794695691 ) ) ;
#2572=LINE ( 'NONE', #118, #27065 ) ;
#2573=LINE ( 'NONE', #14280, #6842 ) ;
#2577=VECTOR ( 'NONE', #41, 1000.000000000000000 ) ;
#2578=CARTESIAN_POINT ( 'NONE',  ( 137.2287565553230309, -1.999999999999979572, -29.49038105676660138 ) ) ;
#2581=CARTESIAN_POINT ( 'NONE',  ( 94.27072269707019814, -4.999999999999992006, 68.49168918522173044 ) ) ;
#2582=LINE ( 'NONE', #7142, #9582 ) ;
#2583=ORIENTED_EDGE ( 'NONE', *, *, #22381, .F. ) ;
#2585=DIRECTION ( 'NONE',  ( 0.5877852522924731371, 0.000000000000000000, 0.8090169943749474513 ) ) ;
#2587=LINE ( 'NONE', #30105, #14938 ) ;
#2588=EDGE_LOOP ( 'NONE', ( #26292, #8509, #22302, #16171, #6464 ) ) ;
#2592=DIRECTION ( 'NONE',  ( 1.000000000000000000, 2.698458740408365879E-16, -1.110223024625156540E-16 ) ) ;
#2593=FACE_OUTER_BOUND ( 'NONE', #19222, .T. ) ;
#2594=EDGE_CURVE ( 'NONE', #15731, #14637, #16047, .T. ) ;
#2595=LINE ( 'NONE', #16612, #21057 ) ;
#2596=EDGE_CURVE ( 'NONE', #2498, #5840, #13904, .T. ) ;
#2598=DIRECTION ( 'NONE',  ( 1.000000000000000000, 2.908569913943825554E-16, -6.938893903907227392E-16 ) ) ;
#2599=DIRECTION ( 'NONE',  ( -2.698458740408365879E-16, 1.000000000000000000, 0.000000000000000000 ) ) ;
#2600=CARTESIAN_POINT ( 'NONE',  ( 175.7287565553229456, -4.999999999999970690, 3.500000000000003109 ) ) ;
#2602=CARTESIAN_POINT ( 'NONE',  ( 159.7287565553230309, -4.999999999999974243, -33.82050807568879947 ) ) ;
#2605=CARTESIAN_POINT ( 'NONE',  ( 151.1922820468854525, -4.999999999999976907, -28.06379628232387802 ) ) ;
#2607=ORIENTED_EDGE ( 'NONE', *, *, #5320, .T. ) ;
#2610=CARTESIAN_POINT ( 'NONE',  ( 148.6922820468853672, -1.999999999999977129, 2.247092850131519715 ) ) ;
#2613=FACE_BOUND ( 'NONE', #4391, .T. ) ;
#2614=ORIENTED_EDGE ( 'NONE', *, *, #4600, .F. ) ;
#2616=ORIENTED_EDGE ( 'NONE', *, *, #27322, .F. ) ;
#2618=CARTESIAN_POINT ( 'NONE',  ( 174.5152310637604671, -9.999999999999994671, -30.37205893520531319 ) ) ;
#2620=LINE ( 'NONE', #29311, #4429 ) ;
#2622=ORIENTED_EDGE ( 'NONE', *, *, #6057, .T. ) ;
#2623=DIRECTION ( 'NONE',  ( -2.698458740408365879E-16, 1.000000000000000000, 0.000000000000000000 ) ) ;
#2626=VERTEX_POINT ( 'NONE', #28305 ) ;
#2631=VECTOR ( 'NONE', #18990, 1000.000000000000000 ) ;
#2632=DIRECTION ( 'NONE',  ( -2.698458740408365879E-16, 1.000000000000000000, 0.000000000000000000 ) ) ;
#2635=VERTEX_POINT ( 'NONE', #2191 ) ;
#2636=FACE_BOUND ( 'NONE', #7512, .T. ) ;
#2637=EDGE_LOOP ( 'NONE', ( #6521, #20563, #29066, #15430, #7898, #13260 ) ) ;
#2639=LINE ( 'NONE', #14509, #17992 ) ;
#2643=DIRECTION ( 'NONE',  ( 0.9510565162951536422, 2.566386769018988816E-16, 0.3090169943749472292 ) ) ;
#2644=EDGE_CURVE ( 'NONE', #4011, #6733, #9617, .T. ) ;
#2647=ORIENTED_EDGE ( 'NONE', *, *, #442, .F. ) ;
#2652=DIRECTION ( 'NONE',  ( 0.5877852522924731371, 1.586114251531760728E-16, -0.8090169943749474513 ) ) ;
#2653=FACE_OUTER_BOUND ( 'NONE', #5134, .T. ) ;
#2655=PLANE ( 'NONE',  #28635 ) ;
#2657=ORIENTED_EDGE ( 'NONE', *, *, #6571, .F. ) ;
#2659=CARTESIAN_POINT ( 'NONE',  ( 154.7287565553229172, -1.999999999999975353, -16.50000000000000000 ) ) ;
#2660=LINE ( 'NONE', #11793, #27223 ) ;
#2663=DIRECTION ( 'NONE',  ( 0.5877852522924731371, 1.586114251531760728E-16, -0.8090169943749474513 ) ) ;
#2666=VECTOR ( 'NONE', #11845, 1000.000000000000000 ) ;
#2667=ORIENTED_EDGE ( 'NONE', *, *, #11288, .T. ) ;
#2668=DIRECTION ( 'NONE',  ( -0.9510565162951536422, -2.566386769018988816E-16, -0.3090169943749472292 ) ) ;
#2669=LINE ( 'NONE', #21271, #24065 ) ;
#2670=LINE ( 'NONE', #25714, #12468 ) ;
#2671=CARTESIAN_POINT ( 'NONE',  ( 164.7287565553228887, -1.999999999999972689, 0.8205080756887930260 ) ) ;
#2678=ORIENTED_EDGE ( 'NONE', *, *, #23481, .T. ) ;
#2681=EDGE_CURVE ( 'NONE', #10405, #10807, #2501, .T. ) ;
#2683=DIRECTION ( 'NONE',  ( -0.9510565162951536422, -2.566386769018988323E-16, 0.3090169943749475623 ) ) ;
#2684=CARTESIAN_POINT ( 'NONE',  ( 151.1922820468854241, -1.999999999999975797, -22.25671179336496053 ) ) ;
#2686=CARTESIAN_POINT ( 'NONE',  ( 149.5152310637605524, -1.999999999999975797, -21.71180489736091346 ) ) ;
#2687=ORIENTED_EDGE ( 'NONE', *, *, #16523, .T. ) ;
#2688=DIRECTION ( 'NONE',  ( -0.5877852522924731371, -1.586114251531760235E-16, 0.8090169943749474513 ) ) ;
#2690=ORIENTED_EDGE ( 'NONE', *, *, #19611, .F. ) ;
#2692=LINE ( 'NONE', #2848, #19554 ) ;
#2694=VERTEX_POINT ( 'NONE', #23383 ) ;
#2696=EDGE_LOOP ( 'NONE', ( #19357, #4464, #18008, #2308 ) ) ;
#2700=ORIENTED_EDGE ( 'NONE', *, *, #23049, .F. ) ;
#2702=VECTOR ( 'NONE', #24441, 1000.000000000000000 ) ;
#2703=ORIENTED_EDGE ( 'NONE', *, *, #27450, .T. ) ;
#2704=DIRECTION ( 'NONE',  ( 1.110223024625156540E-16, 2.995891024602366092E-32, 1.000000000000000000 ) ) ;
#2705=CARTESIAN_POINT ( 'NONE',  ( 164.5152310637604671, -9.999999999999998224, -2.627941064794695691 ) ) ;
#2707=LINE ( 'NONE', #16587, #24077 ) ;
#2712=VERTEX_POINT ( 'NONE', #11321 ) ;
#2713=EDGE_CURVE ( 'NONE', #11968, #18587, #27852, .T. ) ;
#2715=CARTESIAN_POINT ( 'NONE',  ( 153.6922820468854241, -1.999999999999975797, -23.73366926340167282 ) ) ;
#2717=EDGE_CURVE ( 'NONE', #968, #26624, #2344, .T. ) ;
#2719=LINE ( 'NONE', #2581, #19985 ) ;
#2720=ADVANCED_FACE ( 'NONE', ( #16505 ), #28155, .T. ) ;
#2721=EDGE_LOOP ( 'NONE', ( #26013, #24206, #27600, #14580 ) ) ;
#2722=FACE_OUTER_BOUND ( 'NONE', #25105, .T. ) ;
#2723=VERTEX_POINT ( 'NONE', #23535 ) ;
#2725=CARTESIAN_POINT ( 'NONE',  ( 142.2287565553230024, -10.00000000000000533, -3.509618943233403510 ) ) ;
#2726=CARTESIAN_POINT ( 'NONE',  ( 14.02072799663827141, -5.000000000000014211, 43.15136373446576101 ) ) ;
#2730=ORIENTED_EDGE ( 'NONE', *, *, #21680, .T. ) ;
#2735=LINE ( 'NONE', #4709, #20367 ) ;
#2736=DIRECTION ( 'NONE',  ( 1.000000000000000000, 2.698458740408365879E-16, -1.110223024625156540E-16 ) ) ;
#2737=CARTESIAN_POINT ( 'NONE',  ( 143.6922820468854525, -1.999999999999978018, -26.58683881228715506 ) ) ;
#2742=SURFACE_STYLE_USAGE ( .BOTH. , #27809 ) ;
#2744=DIRECTION ( 'NONE',  ( -2.698458740408365879E-16, 1.000000000000000000, 0.000000000000000000 ) ) ;
#2746=LINE ( 'NONE', #20889, #499 ) ;
#2747=VECTOR ( 'NONE', #6423, 1000.000000000000000 ) ;
#2748=LINE ( 'NONE', #306, #11872 ) ;
#2750=CARTESIAN_POINT ( 'NONE',  ( 125.7287565553229456, -84.33034373659255323, -33.50000000000000000 ) ) ;
#2752=ORIENTED_EDGE ( 'NONE', *, *, #13723, .T. ) ;
#2754=VERTEX_POINT ( 'NONE', #7060 ) ;
#2755=EDGE_CURVE ( 'NONE', #14083, #2431, #16352, .T. ) ;
#2758=ADVANCED_FACE ( 'NONE', ( #196 ), #9476, .T. ) ;
#2761=ADVANCED_FACE ( 'NONE', ( #11915 ), #348, .T. ) ;
#2762=ORIENTED_EDGE ( 'NONE', *, *, #15166, .F. ) ;
#2763=ORIENTED_EDGE ( 'NONE', *, *, #13385, .F. ) ;
#2764=ORIENTED_EDGE ( 'NONE', *, *, #5295, .F. ) ;
#2766=PLANE ( 'NONE',  #14007 ) ;
#2767=VECTOR ( 'NONE', #26977, 1000.000000000000000 ) ;
#2769=LINE ( 'NONE', #12052, #865 ) ;
#2770=VERTEX_POINT ( 'NONE', #1105 ) ;
#2771=CARTESIAN_POINT ( 'NONE',  ( 149.5152310637605524, -4.999999999999976907, -11.28819510263909542 ) ) ;
#2772=VERTEX_POINT ( 'NONE', #7505 ) ;
#2774=VERTEX_POINT ( 'NONE', #14801 ) ;
#2775=VECTOR ( 'NONE', #28779, 1000.000000000000000 ) ;
#2779=VECTOR ( 'NONE', #18607, 1000.000000000000000 ) ;
#2780=CARTESIAN_POINT ( 'NONE',  ( 148.6922820468853672, -1.999999999999977573, -0.6060766987539614181 ) ) ;
#2786=EDGE_CURVE ( 'NONE', #26001, #27081, #5060, .T. ) ;
#2787=CARTESIAN_POINT ( 'NONE',  ( 169.7287565553229172, -9.999999999999996447, -16.50000000000000355 ) ) ;
#2790=CARTESIAN_POINT ( 'NONE',  ( 139.7287565553230309, -10.00000000000000533, -25.16025403784439973 ) ) ;
#2792=VECTOR ( 'NONE', #29034, 1000.000000000000000 ) ;
#2798=CARTESIAN_POINT ( 'NONE',  ( 154.5152310637605808, -1.999999999999974021, -28.60870317832789667 ) ) ;
#2799=ORIENTED_EDGE ( 'NONE', *, *, #16998, .F. ) ;
#2800=CARTESIAN_POINT ( 'NONE',  ( 172.0152310637604387, -1.999999999999970024, -17.38167787843871182 ) ) ;
#2801=ORIENTED_EDGE ( 'NONE', *, *, #647, .T. ) ;
#2803=ORIENTED_EDGE ( 'NONE', *, *, #2420, .T. ) ;
#2806=DIRECTION ( 'NONE',  ( 0.5877852522924731371, 0.000000000000000000, 0.8090169943749474513 ) ) ;
#2809=CARTESIAN_POINT ( 'NONE',  ( 133.6922820468854241, -10.00000000000000711, -6.413161187712875133 ) ) ;
#2811=ORIENTED_EDGE ( 'NONE', *, *, #7531, .T. ) ;
#2814=VECTOR ( 'NONE', #27532, 1000.000000000000000 ) ;
#2815=CARTESIAN_POINT ( 'NONE',  ( 133.6922820468854241, -4.999999999999981348, -26.58683881228715506 ) ) ;
#2818=VERTEX_POINT ( 'NONE', #28455 ) ;
#2823=DIRECTION ( 'NONE',  ( -0.5877852522924731371, 0.000000000000000000, 0.8090169943749474513 ) ) ;
#2824=EDGE_LOOP ( 'NONE', ( #1513, #5546, #4035, #7617, #25091 ) ) ;
#2826=EDGE_CURVE ( 'NONE', #4536, #3628, #9783, .T. ) ;
#2827=PLANE ( 'NONE',  #27440 ) ;
#2828=DIRECTION ( 'NONE',  ( 0.9510565162951536422, 0.000000000000000000, -0.3090169943749475623 ) ) ;
#2830=DIRECTION ( 'NONE',  ( 1.000000000000000000, 2.168404344971006896E-16, 0.000000000000000000 ) ) ;
#2831=FACE_OUTER_BOUND ( 'NONE', #8191, .T. ) ;
#2837=ORIENTED_EDGE ( 'NONE', *, *, #10306, .F. ) ;
#2839=AXIS2_PLACEMENT_3D ( 'NONE', #16651, #28295, #11604 ) ;
#2840=DIRECTION ( 'NONE',  ( 0.3090169943749475623, 8.338696094058001131E-17, 0.9510565162951536422 ) ) ;
#2841=CARTESIAN_POINT ( 'NONE',  ( 169.7287565553229172, -9.999999999999996447, -16.50000000000000355 ) ) ;
#2842=DIRECTION ( 'NONE',  ( -2.698458740408365879E-16, 1.000000000000000000, 0.000000000000000000 ) ) ;
#2844=EDGE_LOOP ( 'NONE', ( #9643, #26462, #23724, #7699 ) ) ;
#2845=DIRECTION ( 'NONE',  ( 0.000000000000000000, 0.7071067811865462405, -0.7071067811865489050 ) ) ;
#2847=CARTESIAN_POINT ( 'NONE',  ( 153.6922820468853388, -1.999999999999976241, -0.6060766987539614181 ) ) ;
#2848=CARTESIAN_POINT ( 'NONE',  ( 129.5152310637605524, -10.00000000000000888, -30.37205893520530964 ) ) ;
#2849=VERTEX_POINT ( 'NONE', #8092 ) ;
#2852=ORIENTED_EDGE ( 'NONE', *, *, #20783, .T. ) ;
#2858=ADVANCED_FACE ( 'NONE', ( #19098 ), #25984, .T. ) ;
#2859=EDGE_CURVE ( 'NONE', #7377, #1843, #14351, .T. ) ;
#2860=VECTOR ( 'NONE', #24545, 1000.000000000000000 ) ;
#2861=EDGE_CURVE ( 'NONE', #14702, #25081, #21996, .T. ) ;
#2863=EDGE_CURVE ( 'NONE', #7345, #8301, #5214, .T. ) ;
#2864=DIRECTION ( 'NONE',  ( -0.5877852522924731371, -1.586114251531760235E-16, 0.8090169943749474513 ) ) ;
#2866=PLANE ( 'NONE',  #29779 ) ;
#2868=LINE ( 'NONE', #23771, #19216 ) ;
#2869=DIRECTION ( 'NONE',  ( 0.3090169943749475623, 8.338696094058001131E-17, 0.9510565162951536422 ) ) ;
#2873=LINE ( 'NONE', #10012, #5127 ) ;
#2875=DIRECTION ( 'NONE',  ( -2.698458740408365879E-16, 1.000000000000000000, 0.000000000000000000 ) ) ;
#2879=VECTOR ( 'NONE', #21888, 1000.000000000000000 ) ;
#2880=LINE ( 'NONE', #14290, #25154 ) ;
#2882=ORIENTED_EDGE ( 'NONE', *, *, #11285, .T. ) ;
#2883=CARTESIAN_POINT ( 'NONE',  ( 147.2287565553230309, -4.999999999999977796, -20.83012701892220164 ) ) ;
#2884=AXIS2_PLACEMENT_3D ( 'NONE', #12421, #15005, #22044 ) ;
#2885=ORIENTED_EDGE ( 'NONE', *, *, #5510, .T. ) ;
#2890=VERTEX_POINT ( 'NONE', #5372 ) ;
#2893=LINE ( 'NONE', #1058, #28725 ) ;
#2896=EDGE_CURVE ( 'NONE', #11499, #983, #12520, .T. ) ;
#2898=VERTEX_POINT ( 'NONE', #19392 ) ;
#2899=LINE ( 'NONE', #14758, #1605 ) ;
#2900=EDGE_CURVE ( 'NONE', #17052, #16411, #21840, .T. ) ;
#2901=CARTESIAN_POINT ( 'NONE',  ( 134.5152310637605808, -4.999999999999980460, -28.60870317832789311 ) ) ;
#2903=DIRECTION ( 'NONE',  ( -0.9510565162951536422, -2.566386769018988323E-16, 0.3090169943749475623 ) ) ;
#2905=CARTESIAN_POINT ( 'NONE',  ( 134.5152310637605524, -4.999999999999981348, -1.493419066897600538E-14 ) ) ;
#2908=DIRECTION ( 'NONE',  ( 0.5877852522924731371, 1.586114251531760728E-16, -0.8090169943749474513 ) ) ;
#2910=VERTEX_POINT ( 'NONE', #10232 ) ;
#2915=FACE_BOUND ( 'NONE', #5984, .T. ) ;
#2921=VERTEX_POINT ( 'NONE', #19243 ) ;
#2922=DIRECTION ( 'NONE',  ( -1.110223024625156540E-16, 0.000000000000000000, -1.000000000000000000 ) ) ;
#2923=ORIENTED_EDGE ( 'NONE', *, *, #6603, .F. ) ;
#2925=EDGE_CURVE ( 'NONE', #11270, #756, #24289, .T. ) ;
#2926=VERTEX_POINT ( 'NONE', #3099 ) ;
#2927=VECTOR ( 'NONE', #11292, 1000.000000000000000 ) ;
#2931=ORIENTED_EDGE ( 'NONE', *, *, #17744, .F. ) ;
#2932=CARTESIAN_POINT ( 'NONE',  ( 133.6922820468854241, -10.00000000000000711, -23.73366926340167282 ) ) ;
#2933=LINE ( 'NONE', #28591, #25948 ) ;
#2938=EDGE_CURVE ( 'NONE', #8559, #25751, #14657, .T. ) ;
#2939=ORIENTED_EDGE ( 'NONE', *, *, #23417, .F. ) ;
#2940=ADVANCED_FACE ( 'NONE', ( #17112 ), #12676, .T. ) ;
#2941=LINE ( 'NONE', #14503, #22725 ) ;
#2942=EDGE_CURVE ( 'NONE', #7113, #24158, #19840, .T. ) ;
#2943=FACE_BOUND ( 'NONE', #14033, .T. ) ;
#2944=AXIS2_PLACEMENT_3D ( 'NONE', #1006, #17307, #17456 ) ;
#2945=VERTEX_POINT ( 'NONE', #15716 ) ;
#2947=PLANE ( 'NONE',  #20859 ) ;
#2948=DIRECTION ( 'NONE',  ( 1.110223024625156540E-16, 2.995891024602366092E-32, 1.000000000000000000 ) ) ;
#2949=VECTOR ( 'NONE', #9870, 1000.000000000000000 ) ;
#2950=CARTESIAN_POINT ( 'NONE',  ( 153.6922820468853388, -4.999999999999975131, 2.247092850131519715 ) ) ;
#2951=DIRECTION ( 'NONE',  ( -0.5877852522924731371, -1.586114251531760235E-16, 0.8090169943749474513 ) ) ;
#2952=AXIS2_PLACEMENT_3D ( 'NONE', #6492, #20660, #25551 ) ;
#2954=CARTESIAN_POINT ( 'NONE',  ( 25.07260858567070372, -5.000000000000010658, -77.16555467815769020 ) ) ;
#2955=CARTESIAN_POINT ( 'NONE',  ( 143.6922820468854241, -1.999999999999978462, -6.413161187712876909 ) ) ;
#2956=ORIENTED_EDGE ( 'NONE', *, *, #11250, .F. ) ;
#2958=ORIENTED_EDGE ( 'NONE', *, *, #29135, .F. ) ;
#2961=DIRECTION ( 'NONE',  ( 0.5877852522924731371, 1.586114251531760728E-16, -0.8090169943749474513 ) ) ;
#2963=PLANE ( 'NONE',  #22438 ) ;
#2964=ORIENTED_EDGE ( 'NONE', *, *, #15363, .T. ) ;
#2965=PLANE ( 'NONE',  #24708 ) ;
#2967=VECTOR ( 'NONE', #3993, 1000.000000000000000 ) ;
#2968=VERTEX_POINT ( 'NONE', #29839 ) ;
#2972=PLANE ( 'NONE',  #16930 ) ;
#2975=VERTEX_POINT ( 'NONE', #22602 ) ;
#2981=ORIENTED_EDGE ( 'NONE', *, *, #5896, .F. ) ;
#2984=ORIENTED_EDGE ( 'NONE', *, *, #12627, .F. ) ;
#2986=DIRECTION ( 'NONE',  ( -2.698458740408365879E-16, 1.000000000000000000, 0.000000000000000000 ) ) ;
#2987=AXIS2_PLACEMENT_3D ( 'NONE', #17203, #10327, #10020 ) ;
#2989=DIRECTION ( 'NONE',  ( -2.698458740408365879E-16, 1.000000000000000000, 0.000000000000000000 ) ) ;
#2990=VECTOR ( 'NONE', #5459, 1000.000000000000000 ) ;
#2991=DIRECTION ( 'NONE',  ( 1.110223024625156540E-16, 2.995891024602366092E-32, 1.000000000000000000 ) ) ;
#2996=EDGE_LOOP ( 'NONE', ( #24377, #11855, #13712, #737 ) ) ;
#2998=DIRECTION ( 'NONE',  ( -1.110223024625156540E-16, 0.000000000000000000, -1.000000000000000000 ) ) ;
#3001=CARTESIAN_POINT ( 'NONE',  ( 138.6922820468854241, -1.999999999999979572, 2.247092850131519715 ) ) ;
#3003=LINE ( 'NONE', #9526, #12458 ) ;
#3006=LINE ( 'NONE', #21142, #14428 ) ;
#3007=PLANE ( 'NONE',  #13229 ) ;
#3010=VERTEX_POINT ( 'NONE', #2605 ) ;
#3017=EDGE_LOOP ( 'NONE', ( #10896, #20345, #23474, #22065, #2703 ) ) ;
#3019=LINE ( 'NONE', #12597, #23079 ) ;
#3020=VERTEX_POINT ( 'NONE', #11291 ) ;
#3022=ORIENTED_EDGE ( 'NONE', *, *, #11914, .F. ) ;
#3023=LINE ( 'NONE', #10310, #13362 ) ;
#3028=CARTESIAN_POINT ( 'NONE',  ( 133.7287565553229456, -9.999999999999980460, 8.500000000000007105 ) ) ;
#3030=CARTESIAN_POINT ( 'NONE',  ( 132.0152310637605524, -10.00000000000000711, -26.04193191628310800 ) ) ;
#3032=EDGE_CURVE ( 'NONE', #18212, #9897, #11880, .T. ) ;
#3033=EDGE_CURVE ( 'NONE', #23017, #18285, #27660, .T. ) ;
#3034=ORIENTED_EDGE ( 'NONE', *, *, #5777, .T. ) ;
#3035=CARTESIAN_POINT ( 'NONE',  ( 142.2287565553230309, -4.999999999999978684, -29.49038105676659427 ) ) ;
#3036=EDGE_CURVE ( 'NONE', #475, #10764, #14012, .T. ) ;
#3037=VECTOR ( 'NONE', #25520, 1000.000000000000000 ) ;
#3038=FACE_OUTER_BOUND ( 'NONE', #4714, .T. ) ;
#3039=ORIENTED_EDGE ( 'NONE', *, *, #13566, .F. ) ;
#3041=EDGE_LOOP ( 'NONE', ( #10760, #4891, #29811, #26534 ) ) ;
#3048=VECTOR ( 'NONE', #3377, 1000.000000000000000 ) ;
#3049=DIRECTION ( 'NONE',  ( -2.698458740408365879E-16, 1.000000000000000000, 0.000000000000000000 ) ) ;
#3051=DIRECTION ( 'NONE',  ( -2.698458740408365879E-16, 1.000000000000000000, 0.000000000000000000 ) ) ;
#3054=FACE_OUTER_BOUND ( 'NONE', #22028, .T. ) ;
#3055=LINE ( 'NONE', #21502, #22611 ) ;
#3057=LINE ( 'NONE', #5177, #30207 ) ;
#3059=ORIENTED_EDGE ( 'NONE', *, *, #23172, .F. ) ;
#3061=LINE ( 'NONE', #2610, #21729 ) ;
#3062=VECTOR ( 'NONE', #21797, 1000.000000000000000 ) ;
#3066=ORIENTED_EDGE ( 'NONE', *, *, #3952, .F. ) ;
#3067=VERTEX_POINT ( 'NONE', #2155 ) ;
#3068=EDGE_CURVE ( 'NONE', #16190, #15401, #23344, .T. ) ;
#3071=FACE_OUTER_BOUND ( 'NONE', #14781, .T. ) ;
#3076=DIRECTION ( 'NONE',  ( -1.110223024625156540E-16, 0.000000000000000000, -1.000000000000000000 ) ) ;
#3080=CARTESIAN_POINT ( 'NONE',  ( 174.5152310637604671, -1.999999999999969358, -19.94844914048349693 ) ) ;
#3083=ORIENTED_EDGE ( 'NONE', *, *, #20735, .F. ) ;
#3087=AXIS2_PLACEMENT_3D ( 'NONE', #22904, #13420, #25338 ) ;
#3088=CARTESIAN_POINT ( 'NONE',  ( 157.0152310637604671, -4.999999999999975131, 1.702185954127501066 ) ) ;
#3089=ORIENTED_EDGE ( 'NONE', *, *, #12760, .T. ) ;
#3095=VECTOR ( 'NONE', #1629, 1000.000000000000000 ) ;
#3097=FACE_BOUND ( 'NONE', #21375, .T. ) ;
#3098=CARTESIAN_POINT ( 'NONE',  ( 173.6922820468852819, -9.999999999999996447, -6.413161187712876909 ) ) ;
#3099=CARTESIAN_POINT ( 'NONE',  ( 152.0152310637605240, -4.999999999999976907, -6.958068083716895558 ) ) ;
#3100=DIRECTION ( 'NONE',  ( -2.698458740408365879E-16, 1.000000000000000000, 0.000000000000000000 ) ) ;
#3101=CARTESIAN_POINT ( 'NONE',  ( 152.0152310637606092, -10.00000000000000000, -32.93883019725009120 ) ) ;
#3103=CARTESIAN_POINT ( 'NONE',  ( 157.0152310637605240, -10.00000000000000000, -15.61832212156129707 ) ) ;
#3104=DIRECTION ( 'NONE',  ( -0.8090169943749474513, -2.183098979609982436E-16, -0.5877852522924731371 ) ) ;
#3105=ORIENTED_EDGE ( 'NONE', *, *, #10861, .T. ) ;
#3107=ADVANCED_FACE ( 'NONE', ( #16314 ), #2306, .T. ) ;
#3108=EDGE_CURVE ( 'NONE', #20929, #24158, #5023, .T. ) ;
#3109=VECTOR ( 'NONE', #30197, 1000.000000000000000 ) ;
#3112=DIRECTION ( 'NONE',  ( -0.8090169943749474513, -2.183098979609982436E-16, 0.5877852522924731371 ) ) ;
#3113=EDGE_CURVE ( 'NONE', #28338, #23116, #14619, .T. ) ;
#3114=CARTESIAN_POINT ( 'NONE',  ( 153.6922820468853388, -1.999999999999976241, -17.92658477444275533 ) ) ;
#3115=EDGE_LOOP ( 'NONE', ( #14230, #7190, #14496, #28854 ) ) ;
#3116=CARTESIAN_POINT ( 'NONE',  ( 156.1922820468853672, -1.999999999999974909, -13.59645775552055902 ) ) ;
#3124=ORIENTED_EDGE ( 'NONE', *, *, #23242, .T. ) ;
#3125=CARTESIAN_POINT ( 'NONE',  ( 133.6922820468854241, -1.999999999999980904, 2.247092850131519715 ) ) ;
#3128=ORIENTED_EDGE ( 'NONE', *, *, #27009, .T. ) ;
#3129=CARTESIAN_POINT ( 'NONE',  ( 172.0152310637604103, -9.999999999999996447, 1.702185954127501066 ) ) ;
#3130=ORIENTED_EDGE ( 'NONE', *, *, #8422, .F. ) ;
#3131=VERTEX_POINT ( 'NONE', #3611 ) ;
#3132=LINE ( 'NONE', #14085, #24889 ) ;
#3133=VECTOR ( 'NONE', #15221, 1000.000000000000000 ) ;
#3134=DIRECTION ( 'NONE',  ( -2.698458740408365879E-16, 1.000000000000000000, 0.000000000000000000 ) ) ;
#3135=EDGE_CURVE ( 'NONE', #25090, #26900, #16774, .T. ) ;
#3136=DIRECTION ( 'NONE',  ( -2.698458740408365879E-16, 1.000000000000000000, 0.000000000000000000 ) ) ;
#3137=CARTESIAN_POINT ( 'NONE',  ( 131.1922820468854241, -10.00000000000000888, -4.936203717676158398 ) ) ;
#3138=CARTESIAN_POINT ( 'NONE',  ( 86.87998469340118390, -4.999999999999993783, 63.12200371221075557 ) ) ;
#3143=ORIENTED_EDGE ( 'NONE', *, *, #24560, .F. ) ;
#3144=LINE ( 'NONE', #690, #11009 ) ;
#3145=LINE ( 'NONE', #10281, #4824 ) ;
#3147=LINE ( 'NONE', #17454, #12744 ) ;
#3148=EDGE_CURVE ( 'NONE', #7135, #10866, #3057, .T. ) ;
#3149=DIRECTION ( 'NONE',  ( -0.5877852522924731371, 0.000000000000000000, 0.8090169943749474513 ) ) ;
#3151=EDGE_CURVE ( 'NONE', #24767, #29985, #9743, .T. ) ;
#3153=DIRECTION ( 'NONE',  ( -0.5877852522924731371, 0.000000000000000000, 0.8090169943749474513 ) ) ;
#3154=ADVANCED_FACE ( 'NONE', ( #14469 ), #608, .T. ) ;
#3156=CARTESIAN_POINT ( 'NONE',  ( 139.7287565553230309, -10.00000000000000533, -33.82050807568879947 ) ) ;
#3159=AXIS2_PLACEMENT_3D ( 'NONE', #4835, #14133, #23462 ) ;
#3166=EDGE_LOOP ( 'NONE', ( #2099, #5032, #27069, #28833 ) ) ;
#3167=ORIENTED_EDGE ( 'NONE', *, *, #2900, .F. ) ;
#3168=DIRECTION ( 'NONE',  ( -0.5877852522924731371, -1.586114251531760235E-16, 0.8090169943749474513 ) ) ;
#3170=ORIENTED_EDGE ( 'NONE', *, *, #28913, .F. ) ;
#3171=EDGE_CURVE ( 'NONE', #1746, #20723, #21351, .T. ) ;
#3173=LINE ( 'NONE', #12442, #22318 ) ;
#3174=FACE_OUTER_BOUND ( 'NONE', #2526, .T. ) ;
#3179=PLANE ( 'NONE',  #9788 ) ;
#3180=CARTESIAN_POINT ( 'NONE',  ( 152.0152310637604955, -1.999999999999976241, -15.61832212156129351 ) ) ;
#3182=LINE ( 'NONE', #26525, #9732 ) ;
#3183=DIRECTION ( 'NONE',  ( 0.3090169943749475623, 8.338696094058001131E-17, 0.9510565162951536422 ) ) ;
#3184=ORIENTED_EDGE ( 'NONE', *, *, #2942, .T. ) ;
#3185=CARTESIAN_POINT ( 'NONE',  ( 168.6922820468852819, -1.999999999999971800, 2.247092850131519715 ) ) ;
#3186=PLANE ( 'NONE',  #26876 ) ;
#3187=CARTESIAN_POINT ( 'NONE',  ( 129.5152310637605524, -10.00000000000000888, -4.391296821672111328 ) ) ;
#3188=ORIENTED_EDGE ( 'NONE', *, *, #7623, .F. ) ;
#3189=ORIENTED_EDGE ( 'NONE', *, *, #14200, .F. ) ;
#3191=ORIENTED_EDGE ( 'NONE', *, *, #2786, .T. ) ;
#3194=LINE ( 'NONE', #12318, #12114 ) ;
#3195=CARTESIAN_POINT ( 'NONE',  ( 9.407815906149622265, -5.000000000000015099, 28.95428013513216925 ) ) ;
#3196=CIRCLE ( 'NONE', #27587, 3.000000000000002665 ) ;
#3197=DIRECTION ( 'NONE',  ( 0.5877852522924731371, 0.000000000000000000, 0.8090169943749474513 ) ) ;
#3198=FACE_OUTER_BOUND ( 'NONE', #21569, .T. ) ;
#3199=ADVANCED_FACE ( 'NONE', ( #12903 ), #12332, .T. ) ;
#3200=LINE ( 'NONE', #12632, #19158 ) ;
#3201=LINE ( 'NONE', #2120, #21910 ) ;
#3203=DIRECTION ( 'NONE',  ( 0.3090169943749472292, 8.338696094057992503E-17, -0.9510565162951536422 ) ) ;
#3204=CARTESIAN_POINT ( 'NONE',  ( 137.0152310637605808, -4.999999999999980460, -26.04193191628310800 ) ) ;
#3207=VERTEX_POINT ( 'NONE', #7471 ) ;
#3212=FACE_BOUND ( 'NONE', #24, .T. ) ;
#3213=VERTEX_POINT ( 'NONE', #28561 ) ;
#3215=LINE ( 'NONE', #14484, #16494 ) ;
#3217=PLANE ( 'NONE',  #13049 ) ;
#3218=VERTEX_POINT ( 'NONE', #28417 ) ;
#3219=CARTESIAN_POINT ( 'NONE',  ( 133.7287565553229172, -1.999999999999980904, -33.50000000000000000 ) ) ;
#3220=ORIENTED_EDGE ( 'NONE', *, *, #22422, .T. ) ;
#3227=VECTOR ( 'NONE', #11407, 1000.000000000000000 ) ;
#3228=DIRECTION ( 'NONE',  ( -0.9510565162951536422, -2.566386769018988323E-16, 0.3090169943749475623 ) ) ;
#3229=EDGE_LOOP ( 'NONE', ( #13560, #4298, #26514, #13626 ) ) ;
#3238=CARTESIAN_POINT ( 'NONE',  ( 144.5152310637605808, -1.999999999999977129, -21.71180489736091346 ) ) ;
#3239=FACE_BOUND ( 'NONE', #18051, .T. ) ;
#3240=ADVANCED_FACE ( 'NONE', ( #5335 ), #16919, .T. ) ;
#3245=FACE_OUTER_BOUND ( 'NONE', #24557, .T. ) ;
#3246=ORIENTED_EDGE ( 'NONE', *, *, #1450, .T. ) ;
#3247=FACE_OUTER_BOUND ( 'NONE', #25710, .T. ) ;
#3248=VECTOR ( 'NONE', #27756, 1000.000000000000000 ) ;
#3250=LINE ( 'NONE', #17409, #27020 ) ;
#3252=DIRECTION ( 'NONE',  ( -2.698458740408365879E-16, 1.000000000000000000, 0.000000000000000000 ) ) ;
#3253=ORIENTED_EDGE ( 'NONE', *, *, #7874, .T. ) ;
#3254=VECTOR ( 'NONE', #27076, 1000.000000000000000 ) ;
#3258=DIRECTION ( 'NONE',  ( -2.698458740408365879E-16, 1.000000000000000000, 0.000000000000000000 ) ) ;
#3260=ORIENTED_EDGE ( 'NONE', *, *, #23380, .F. ) ;
#3261=PLANE ( 'NONE',  #21758 ) ;
#3262=ORIENTED_EDGE ( 'NONE', *, *, #685, .F. ) ;
#3264=EDGE_LOOP ( 'NONE', ( #9545, #14785, #26529, #1094 ) ) ;
#3267=ORIENTED_EDGE ( 'NONE', *, *, #9277, .T. ) ;
#3271=LINE ( 'NONE', #29551, #29637 ) ;
#3275=VERTEX_POINT ( 'NONE', #744 ) ;
#3276=DIRECTION ( 'NONE',  ( -0.8090169943749474513, -2.183098979609982436E-16, -0.5877852522924731371 ) ) ;
#3278=EDGE_CURVE ( 'NONE', #4517, #3213, #28268, .T. ) ;
#3279=AXIS2_PLACEMENT_3D ( 'NONE', #8884, #9026, #6167 ) ;
#3280=ADVANCED_FACE ( 'NONE', ( #7322 ), #16623, .T. ) ;
#3281=EDGE_CURVE ( 'NONE', #25944, #7041, #29909, .T. ) ;
#3282=CARTESIAN_POINT ( 'NONE',  ( 151.1922820468854241, -10.00000000000000178, -22.25671179336496053 ) ) ;
#3283=EDGE_CURVE ( 'NONE', #17861, #5150, #11219, .T. ) ;
#3284=CARTESIAN_POINT ( 'NONE',  ( 169.5152310637604671, -9.999999999999996447, -21.71180489736091346 ) ) ;
#3293=DIRECTION ( 'NONE',  ( -2.698458740408365879E-16, 1.000000000000000000, 0.000000000000000000 ) ) ;
#3297=DIRECTION ( 'NONE',  ( -2.698458740408365879E-16, 1.000000000000000000, 0.000000000000000000 ) ) ;
#3300=ORIENTED_EDGE ( 'NONE', *, *, #28102, .T. ) ;
#3301=LINE ( 'NONE', #10289, #19309 ) ;
#3303=VECTOR ( 'NONE', #287, 1000.000000000000000 ) ;
#3305=LINE ( 'NONE', #1158, #21016 ) ;
#3306=VERTEX_POINT ( 'NONE', #30052 ) ;
#3309=EDGE_LOOP ( 'NONE', ( #19974, #23855, #29841, #13234 ) ) ;
#3315=AXIS2_PLACEMENT_3D ( 'NONE', #6044, #15034, #24220 ) ;
#3316=ADVANCED_FACE ( 'NONE', ( #8769 ), #20222, .T. ) ;
#3317=DIRECTION ( 'NONE',  ( -0.9510565162951536422, -2.566386769018988323E-16, 0.3090169943749475623 ) ) ;
#3318=ADVANCED_FACE ( 'NONE', ( #24980 ), #27300, .T. ) ;
#3319=EDGE_LOOP ( 'NONE', ( #2678, #3367, #5310, #25559, #28021 ) ) ;
#3320=DIRECTION ( 'NONE',  ( 1.110223024625156540E-16, 2.995891024602366092E-32, 1.000000000000000000 ) ) ;
#3321=VECTOR ( 'NONE', #21531, 1000.000000000000000 ) ;
#3322=FACE_OUTER_BOUND ( 'NONE', #6386, .T. ) ;
#3323=PLANE ( 'NONE',  #12883 ) ;
#3327=LINE ( 'NONE', #3466, #5433 ) ;
#3328=CARTESIAN_POINT ( 'NONE',  ( 147.0152310637605808, -1.999999999999976241, -34.70218595412750773 ) ) ;
#3332=ORIENTED_EDGE ( 'NONE', *, *, #17624, .F. ) ;
#3333=CARTESIAN_POINT ( 'NONE',  ( 172.0152310637604103, -4.999999999999970690, -1.909752701132032663E-14 ) ) ;
#3334=CARTESIAN_POINT ( 'NONE',  ( 172.0152310637604671, -1.999999999999970024, -15.61832212156129707 ) ) ;
#3335=VECTOR ( 'NONE', #7361, 1000.000000000000000 ) ;
#3336=LINE ( 'NONE', #19334, #25381 ) ;
#3337=ORIENTED_EDGE ( 'NONE', *, *, #4358, .F. ) ;
#3340=VECTOR ( 'NONE', #23794, 1000.000000000000000 ) ;
#3343=LINE ( 'NONE', #14901, #11625 ) ;
#3344=DIRECTION ( 'NONE',  ( 1.110223024625156540E-16, 2.995891024602366092E-32, 1.000000000000000000 ) ) ;
#3346=ORIENTED_EDGE ( 'NONE', *, *, #20329, .T. ) ;
#3347=LINE ( 'NONE', #7463, #25488 ) ;
#3351=CARTESIAN_POINT ( 'NONE',  ( 162.0152310637604955, -1.999999999999972244, -26.04193191628311155 ) ) ;
#3352=LINE ( 'NONE', #29018, #10902 ) ;
#3355=AXIS2_PLACEMENT_3D ( 'NONE', #18834, #25871, #2830 ) ;
#3356=ORIENTED_EDGE ( 'NONE', *, *, #16529, .T. ) ;
#3360=FACE_BOUND ( 'NONE', #11696, .T. ) ;
#3361=ORIENTED_EDGE ( 'NONE', *, *, #18637, .F. ) ;
#3363=EDGE_LOOP ( 'NONE', ( #29885, #23813, #6486, #12961 ) ) ;
#3364=DIRECTION ( 'NONE',  ( 0.9510565162951536422, 2.566386769018988816E-16, 0.3090169943749472292 ) ) ;
#3366=CARTESIAN_POINT ( 'NONE',  ( 123.0533251596896918, -4.999999999999984901, -89.40347394098662903 ) ) ;
#3367=ORIENTED_EDGE ( 'NONE', *, *, #23339, .T. ) ;
#3368=DIRECTION ( 'NONE',  ( 0.9510565162951536422, 0.000000000000000000, -0.3090169943749475623 ) ) ;
#3371=EDGE_CURVE ( 'NONE', #4554, #22145, #6648, .T. ) ;
#3372=ORIENTED_EDGE ( 'NONE', *, *, #13657, .F. ) ;
#3375=LINE ( 'NONE', #10519, #14983 ) ;
#3376=ORIENTED_EDGE ( 'NONE', *, *, #6513, .T. ) ;
#3377=DIRECTION ( 'NONE',  ( -2.698458740408365879E-16, 1.000000000000000000, 0.000000000000000000 ) ) ;
#3379=AXIS2_PLACEMENT_3D ( 'NONE', #23689, #946, #24439 ) ;
#3382=FACE_BOUND ( 'NONE', #29804, .T. ) ;
#3386=DIRECTION ( 'NONE',  ( 0.5877852522924731371, 1.586114251531760728E-16, 0.8090169943749474513 ) ) ;
#3389=VECTOR ( 'NONE', #11402, 1000.000000000000000 ) ;
#3393=EDGE_LOOP ( 'NONE', ( #430, #28432, #8760, #4768 ) ) ;
#3396=LINE ( 'NONE', #511, #18039 ) ;
#3398=VERTEX_POINT ( 'NONE', #4355 ) ;
#3400=ORIENTED_EDGE ( 'NONE', *, *, #16305, .T. ) ;
#3402=EDGE_CURVE ( 'NONE', #27090, #11338, #13658, .T. ) ;
#3403=EDGE_CURVE ( 'NONE', #24408, #24131, #22681, .T. ) ;
#3406=EDGE_CURVE ( 'NONE', #16269, #29646, #4507, .T. ) ;
#3407=CARTESIAN_POINT ( 'NONE',  ( 176.1922820468852535, -1.999999999999969580, -2.083034168790677043 ) ) ;
#3411=DIRECTION ( 'NONE',  ( -2.698458740408365879E-16, 1.000000000000000000, 0.000000000000000000 ) ) ;
#3415=ORIENTED_EDGE ( 'NONE', *, *, #8987, .T. ) ;
#3417=EDGE_LOOP ( 'NONE', ( #25701, #28488, #21252, #25724 ) ) ;
#3419=VECTOR ( 'NONE', #1824, 1000.000000000000000 ) ;
#3420=CARTESIAN_POINT ( 'NONE',  ( 163.6922820468853104, -1.999999999999972689, -6.413161187712876909 ) ) ;
#3422=DIRECTION ( 'NONE',  ( -2.698458740408365879E-16, 1.000000000000000000, 0.000000000000000000 ) ) ;
#3423=CARTESIAN_POINT ( 'NONE',  ( 144.5152310637605524, -1.999999999999978018, -2.627941064794695691 ) ) ;
#3424=ORIENTED_EDGE ( 'NONE', *, *, #7605, .T. ) ;
#3429=FACE_OUTER_BOUND ( 'NONE', #5444, .T. ) ;
#3433=LINE ( 'NONE', #19295, #15174 ) ;
#3434=CARTESIAN_POINT ( 'NONE',  ( 142.2287565553230024, -1.999999999999978462, -3.509618943233403510 ) ) ;
#3437=ORIENTED_EDGE ( 'NONE', *, *, #21134, .F. ) ;
#3441=AXIS2_PLACEMENT_3D ( 'NONE', #19559, #24155, #23864 ) ;
#3443=DIRECTION ( 'NONE',  ( -6.938893903907227392E-16, 0.000000000000000000, -1.000000000000000000 ) ) ;
#3444=EDGE_CURVE ( 'NONE', #17843, #2040, #6353, .T. ) ;
#3445=AXIS2_PLACEMENT_3D ( 'NONE', #4645, #13936, #23267 ) ;
#3447=LINE ( 'NONE', #29273, #1850 ) ;
#3450=ORIENTED_EDGE ( 'NONE', *, *, #25757, .F. ) ;
#3451=CARTESIAN_POINT ( 'NONE',  ( 173.6922820468853104, -1.999999999999969580, -15.07341522555727664 ) ) ;
#3454=ORIENTED_EDGE ( 'NONE', *, *, #27182, .T. ) ;
#3457=VECTOR ( 'NONE', #21931, 999.9999999999998863 ) ;
#3459=VECTOR ( 'NONE', #10492, 1000.000000000000000 ) ;
#3460=ORIENTED_EDGE ( 'NONE', *, *, #10987, .T. ) ;
#3462=CARTESIAN_POINT ( 'NONE',  ( 169.5152310637604387, -4.999999999999971578, -2.627941064794695691 ) ) ;
#3466=CARTESIAN_POINT ( 'NONE',  ( 174.7287565553228319, -9.999999999999996447, 0.8205080756887930260 ) ) ;
#3469=CARTESIAN_POINT ( 'NONE',  ( 132.2287565553230024, -10.00000000000000888, -3.509618943233403510 ) ) ;
#3471=LINE ( 'NONE', #6212, #13421 ) ;
#3472=VECTOR ( 'NONE', #13062, 1000.000000000000000 ) ;
#3473=ORIENTED_EDGE ( 'NONE', *, *, #2007, .T. ) ;
#3474=AXIS2_PLACEMENT_3D ( 'NONE', #8157, #28824, #19302 ) ;
#3475=DIRECTION ( 'NONE',  ( -0.8090169943749474513, -2.183098979609982436E-16, 0.5877852522924731371 ) ) ;
#3476=LINE ( 'NONE', #12768, #8320 ) ;
#3478=EDGE_CURVE ( 'NONE', #27514, #28443, #27899, .T. ) ;
#3479=LINE ( 'NONE', #12462, #17572 ) ;
#3480=ORIENTED_EDGE ( 'NONE', *, *, #6299, .T. ) ;
#3481=EDGE_CURVE ( 'NONE', #14185, #102, #7415, .T. ) ;
#3482=ORIENTED_EDGE ( 'NONE', *, *, #29290, .T. ) ;
#3485=ORIENTED_EDGE ( 'NONE', *, *, #18589, .T. ) ;
#3486=ORIENTED_EDGE ( 'NONE', *, *, #5155, .F. ) ;
#3490=CARTESIAN_POINT ( 'NONE',  ( 86.45715817750404142, -4.999999999999993783, 62.81480226644314513 ) ) ;
#3491=CARTESIAN_POINT ( 'NONE',  ( 137.2287565553230309, -10.00000000000000533, -3.509618943233403510 ) ) ;
#3494=ORIENTED_EDGE ( 'NONE', *, *, #25411, .T. ) ;
#3495=LINE ( 'NONE', #28709, #20620 ) ;
#3496=VECTOR ( 'NONE', #5726, 1000.000000000000000 ) ;
#3498=VECTOR ( 'NONE', #15993, 1000.000000000000000 ) ;
#3499=ORIENTED_EDGE ( 'NONE', *, *, #9963, .F. ) ;
#3501=CARTESIAN_POINT ( 'NONE',  ( 142.2287565553230309, -1.999999999999978018, -29.49038105676660138 ) ) ;
#3504=ORIENTED_EDGE ( 'NONE', *, *, #22671, .T. ) ;
#3508=FACE_BOUND ( 'NONE', #13244, .T. ) ;
#3510=LINE ( 'NONE', #13103, #9532 ) ;
#3511=ORIENTED_EDGE ( 'NONE', *, *, #29290, .F. ) ;
#3513=CARTESIAN_POINT ( 'NONE',  ( 132.0152310637605808, -4.999999999999982236, -24.27857615940569147 ) ) ;
#3514=ORIENTED_EDGE ( 'NONE', *, *, #5438, .T. ) ;
#3516=VERTEX_POINT ( 'NONE', #23742 ) ;
#3517=ADVANCED_FACE ( 'NONE', ( #20981 ), #20825, .T. ) ;
#3519=EDGE_LOOP ( 'NONE', ( #20293, #10582, #11280, #18291 ) ) ;
#3522=CARTESIAN_POINT ( 'NONE',  ( 163.6922820468853672, -4.999999999999974243, -26.58683881228715862 ) ) ;
#3523=ORIENTED_EDGE ( 'NONE', *, *, #14405, .F. ) ;
#3529=DIRECTION ( 'NONE',  ( -1.110223024625156540E-16, 0.000000000000000000, -1.000000000000000000 ) ) ;
#3530=VECTOR ( 'NONE', #15251, 1000.000000000000000 ) ;
#3531=ADVANCED_FACE ( 'NONE', ( #16715 ), #7554, .T. ) ;
#3532=PLANE ( 'NONE',  #14588 ) ;
#3534=CARTESIAN_POINT ( 'NONE',  ( 158.6922820468854241, -1.999999999999974021, -32.39392330124607611 ) ) ;
#3536=CARTESIAN_POINT ( 'NONE',  ( 17.11749389674364963, -5.000000000000013323, -52.68222916370584130 ) ) ;
#3538=DIRECTION ( 'NONE',  ( 0.3090169943749472292, 8.338696094057992503E-17, -0.9510565162951536422 ) ) ;
#3542=ORIENTED_EDGE ( 'NONE', *, *, #8065, .T. ) ;
#3545=DIRECTION ( 'NONE',  ( -0.5877852522924731371, 0.000000000000000000, 0.8090169943749474513 ) ) ;
#3546=DIRECTION ( 'NONE',  ( 0.9510565162951535312, 2.566386769018988816E-16, -0.3090169943749475623 ) ) ;
#3548=VERTEX_POINT ( 'NONE', #21282 ) ;
#3549=DIRECTION ( 'NONE',  ( -0.8090169943749474513, -2.183098979609982436E-16, -0.5877852522924731371 ) ) ;
#3555=VERTEX_POINT ( 'NONE', #4655 ) ;
#3556=LINE ( 'NONE', #3407, #27249 ) ;
#3557=VECTOR ( 'NONE', #14688, 1000.000000000000000 ) ;
#3559=LINE ( 'NONE', #22479, #2414 ) ;
#3561=VERTEX_POINT ( 'NONE', #30208 ) ;
#3568=CARTESIAN_POINT ( 'NONE',  ( 129.5152310637605524, -10.00000000000000888, -13.05155085951650840 ) ) ;
#3569=LINE ( 'NONE', #14312, #16259 ) ;
#3570=EDGE_CURVE ( 'NONE', #20929, #27090, #9217, .T. ) ;
#3572=CARTESIAN_POINT ( 'NONE',  ( 176.1922820468853104, -1.999999999999969358, -22.25671179336496053 ) ) ;
#3573=FACE_OUTER_BOUND ( 'NONE', #7576, .T. ) ;
#3574=EDGE_CURVE ( 'NONE', #12466, #26303, #393, .T. ) ;
#3575=LINE ( 'NONE', #1739, #27088 ) ;
#3576=VECTOR ( 'NONE', #17067, 1000.000000000000000 ) ;
#3580=EDGE_LOOP ( 'NONE', ( #8529, #9094, #5921, #30149 ) ) ;
#3581=CARTESIAN_POINT ( 'NONE',  ( 134.5152310637605524, -10.00000000000000533, -30.37205893520530964 ) ) ;
#3582=LINE ( 'NONE', #1000, #19919 ) ;
#3583=CARTESIAN_POINT ( 'NONE',  ( 141.1922820468854525, -10.00000000000000533, -10.74328820663507678 ) ) ;
#3590=CARTESIAN_POINT ( 'NONE',  ( 164.5152310637604671, -1.999999999999972689, -2.627941064794695691 ) ) ;
#3594=VERTEX_POINT ( 'NONE', #12724 ) ;
#3595=PLANE ( 'NONE',  #15896 ) ;
#3598=VECTOR ( 'NONE', #28495, 1000.000000000000000 ) ;
#3599=ORIENTED_EDGE ( 'NONE', *, *, #2566, .F. ) ;
#3602=LINE ( 'NONE', #12897, #26508 ) ;
#3603=VERTEX_POINT ( 'NONE', #12422 ) ;
#3605=DIRECTION ( 'NONE',  ( 0.000000000000000000, 0.000000000000000000, -1.000000000000000000 ) ) ;
#3607=EDGE_CURVE ( 'NONE', #15349, #12234, #3147, .T. ) ;
#3608=EDGE_CURVE ( 'NONE', #23763, #18633, #6018, .T. ) ;
#3609=CARTESIAN_POINT ( 'NONE',  ( 163.6922820468852819, -4.999999999999973355, -0.6060766987539614181 ) ) ;
#3610=ADVANCED_FACE ( 'NONE', ( #10429 ), #10133, .T. ) ;
#3611=CARTESIAN_POINT ( 'NONE',  ( 148.6922820468854241, -4.999999999999977796, -17.92658477444275889 ) ) ;
#3615=CARTESIAN_POINT ( 'NONE',  ( 176.1922820468853388, -9.999999999999994671, -28.06379628232387802 ) ) ;
#3621=CARTESIAN_POINT ( 'NONE',  ( 131.1922820468854241, -10.00000000000000888, -22.25671179336495697 ) ) ;
#3624=CARTESIAN_POINT ( 'NONE',  ( 162.0152310637604103, -4.999999999999974243, -1.798730398669517009E-14 ) ) ;
#3625=CARTESIAN_POINT ( 'NONE',  ( 173.6922820468852535, -1.999999999999970468, 2.247092850131519715 ) ) ;
#3626=CARTESIAN_POINT ( 'NONE',  ( 171.1922820468852819, -9.999999999999996447, -2.083034168790677043 ) ) ;
#3627=ORIENTED_EDGE ( 'NONE', *, *, #23084, .F. ) ;
#3628=VERTEX_POINT ( 'NONE', #9979 ) ;
#3632=PLANE ( 'NONE',  #22856 ) ;
#3633=PLANE ( 'NONE',  #14533 ) ;
#3635=VECTOR ( 'NONE', #26212, 1000.000000000000000 ) ;
#3637=LINE ( 'NONE', #10647, #154 ) ;
#3639=EDGE_LOOP ( 'NONE', ( #9050, #22822, #15923, #16135, #21280 ) ) ;
#3640=EDGE_CURVE ( 'NONE', #8714, #19917, #8145, .T. ) ;
#3642=LINE ( 'NONE', #17222, #3459 ) ;
#3644=EDGE_CURVE ( 'NONE', #11898, #24567, #24488, .T. ) ;
#3651=ORIENTED_EDGE ( 'NONE', *, *, #18862, .T. ) ;
#3654=FACE_BOUND ( 'NONE', #4449, .T. ) ;
#3655=ORIENTED_EDGE ( 'NONE', *, *, #23252, .T. ) ;
#3656=ORIENTED_EDGE ( 'NONE', *, *, #20407, .T. ) ;
#3657=DIRECTION ( 'NONE',  ( 2.698458740408365879E-16, -1.000000000000000000, 0.000000000000000000 ) ) ;
#3658=VECTOR ( 'NONE', #7406, 1000.000000000000000 ) ;
#3660=LINE ( 'NONE', #14634, #18888 ) ;
#3662=CARTESIAN_POINT ( 'NONE',  ( 9.806324804231010717, -5.000000000000015099, 30.18076441017510803 ) ) ;
#3663=ORIENTED_EDGE ( 'NONE', *, *, #16797, .F. ) ;
#3665=ORIENTED_EDGE ( 'NONE', *, *, #29249, .T. ) ;
#3669=ORIENTED_EDGE ( 'NONE', *, *, #14273, .T. ) ;
#3671=VECTOR ( 'NONE', #21317, 1000.000000000000000 ) ;
#3674=FACE_BOUND ( 'NONE', #15846, .T. ) ;
#3675=EDGE_CURVE ( 'NONE', #28746, #9780, #15303, .T. ) ;
#3676=VECTOR ( 'NONE', #21236, 1000.000000000000000 ) ;
#3677=ORIENTED_EDGE ( 'NONE', *, *, #29652, .T. ) ;
#3679=CARTESIAN_POINT ( 'NONE',  ( 156.1922820468854241, -10.00000000000000000, -28.06379628232387802 ) ) ;
#3683=LINE ( 'NONE', #12983, #14852 ) ;
#3685=EDGE_LOOP ( 'NONE', ( #14827, #17290, #18917, #9630 ) ) ;
#3686=DIRECTION ( 'NONE',  ( 0.9510565162951536422, 2.566386769018988816E-16, 0.3090169943749472292 ) ) ;
#3689=ORIENTED_EDGE ( 'NONE', *, *, #19397, .T. ) ;
#3690=CIRCLE ( 'NONE', #28101, 8.000000000000007105 ) ;
#3692=FACE_OUTER_BOUND ( 'NONE', #3685, .T. ) ;
#3695=DIRECTION ( 'NONE',  ( 0.9510565162951535312, 2.566386769018988816E-16, -0.3090169943749475623 ) ) ;
#3696=ORIENTED_EDGE ( 'NONE', *, *, #25754, .F. ) ;
#3701=ORIENTED_EDGE ( 'NONE', *, *, #8983, .T. ) ;
#3704=CARTESIAN_POINT ( 'NONE',  ( 174.5152310637604387, -9.999999999999994671, -21.71180489736091346 ) ) ;
#3706=VERTEX_POINT ( 'NONE', #17162 ) ;
#3707=DIRECTION ( 'NONE',  ( 0.5877852522924731371, 1.586114251531760728E-16, 0.8090169943749474513 ) ) ;
#3708=ADVANCED_FACE ( 'NONE', ( #29263 ), #12873, .T. ) ;
#3711=AXIS2_PLACEMENT_3D ( 'NONE', #28349, #25553, #6799 ) ;
#3713=VERTEX_POINT ( 'NONE', #29107 ) ;
#3715=DIRECTION ( 'NONE',  ( 0.3090169943749472292, 8.338696094057992503E-17, -0.9510565162951536422 ) ) ;
#3716=LINE ( 'NONE', #26785, #28266 ) ;
#3717=VECTOR ( 'NONE', #5427, 1000.000000000000000 ) ;
#3718=DIRECTION ( 'NONE',  ( -2.698458740408365879E-16, 1.000000000000000000, 0.000000000000000000 ) ) ;
#3719=DIRECTION ( 'NONE',  ( -1.110223024625156540E-16, 0.000000000000000000, -1.000000000000000000 ) ) ;
#3720=CARTESIAN_POINT ( 'NONE',  ( 134.5152310637605808, -10.00000000000000533, -28.60870317832789311 ) ) ;
#3721=VECTOR ( 'NONE', #25280, 1000.000000000000000 ) ;
#3723=AXIS2_PLACEMENT_3D ( 'NONE', #1241, #5667, #14947 ) ;
#3725=ORIENTED_EDGE ( 'NONE', *, *, #25254, .T. ) ;
#3728=ORIENTED_EDGE ( 'NONE', *, *, #21754, .F. ) ;
#3729=FACE_OUTER_BOUND ( 'NONE', #23065, .T. ) ;
#3730=LINE ( 'NONE', #17602, #29725 ) ;
#3731=ORIENTED_EDGE ( 'NONE', *, *, #2071, .F. ) ;
#3735=ORIENTED_EDGE ( 'NONE', *, *, #11286, .F. ) ;
#3737=DIRECTION ( 'NONE',  ( 2.908569913943825554E-16, -1.000000000000000000, -0.000000000000000000 ) ) ;
#3740=DIRECTION ( 'NONE',  ( -0.9510565162951536422, -2.566386769018988816E-16, -0.3090169943749472292 ) ) ;
#3744=ORIENTED_EDGE ( 'NONE', *, *, #5489, .F. ) ;
#3745=CARTESIAN_POINT ( 'NONE',  ( 147.2287565553229740, -1.999999999999977129, -3.509618943233403510 ) ) ;
#3746=EDGE_CURVE ( 'NONE', #9765, #2890, #24338, .T. ) ;
#3751=VECTOR ( 'NONE', #23392, 1000.000000000000000 ) ;
#3752=ORIENTED_EDGE ( 'NONE', *, *, #2596, .T. ) ;
#3753=ORIENTED_EDGE ( 'NONE', *, *, #5511, .T. ) ;
#3754=DIRECTION ( 'NONE',  ( -0.5877852522924731371, -1.586114251531760235E-16, 0.8090169943749474513 ) ) ;
#3756=CARTESIAN_POINT ( 'NONE',  ( 144.5152310637605240, -10.00000000000000355, -4.391296821672111328 ) ) ;
#3759=CARTESIAN_POINT ( 'NONE',  ( 144.7287565553230024, -1.999999999999977573, -7.839745962155603820 ) ) ;
#3760=DIRECTION ( 'NONE',  ( -0.5877852522924731371, -1.586114251531760728E-16, -0.8090169943749474513 ) ) ;
#3761=VECTOR ( 'NONE', #6283, 1000.000000000000000 ) ;
#3762=DIRECTION ( 'NONE',  ( -0.8090169943749474513, -2.183098979609982436E-16, 0.5877852522924731371 ) ) ;
#3764=CARTESIAN_POINT ( 'NONE',  ( 176.1922820468852819, -1.999999999999969358, -10.74328820663507678 ) ) ;
#3767=VECTOR ( 'NONE', #10364, 1000.000000000000000 ) ;
#3769=CARTESIAN_POINT ( 'NONE',  ( 166.1922820468853388, -9.999999999999998224, -10.74328820663507678 ) ) ;
#3770=CARTESIAN_POINT ( 'NONE',  ( 172.7287565553229456, -9.999999999999971578, -36.50000000000000711 ) ) ;
#3773=LINE ( 'NONE', #10924, #6612 ) ;
#3775=EDGE_LOOP ( 'NONE', ( #13198, #6077, #9123, #12958 ) ) ;
#3778=DIRECTION ( 'NONE',  ( -0.8090169943749474513, -2.183098979609982436E-16, -0.5877852522924731371 ) ) ;
#3782=EDGE_CURVE ( 'NONE', #12691, #4011, #3433, .T. ) ;
#3787=VECTOR ( 'NONE', #21818, 1000.000000000000000 ) ;
#3788=LINE ( 'NONE', #29321, #15535 ) ;
#3789=CARTESIAN_POINT ( 'NONE',  ( 151.1922820468854241, -4.999999999999976907, -19.40354224447947828 ) ) ;
#3790=EDGE_CURVE ( 'NONE', #4117, #28729, #8735, .T. ) ;
#3792=AXIS2_PLACEMENT_3D ( 'NONE', #16831, #9950, #16984 ) ;
#3793=VERTEX_POINT ( 'NONE', #8886 ) ;
#3794=VERTEX_POINT ( 'NONE', #17749 ) ;
#3795=DIRECTION ( 'NONE',  ( -0.9510565162951536422, -2.566386769018988816E-16, -0.3090169943749472292 ) ) ;
#3799=LINE ( 'NONE', #13089, #12359 ) ;
#3802=EDGE_LOOP ( 'NONE', ( #12869, #5834, #5457, #26760 ) ) ;
#3804=VECTOR ( 'NONE', #9308, 1000.000000000000000 ) ;
#3807=FACE_BOUND ( 'NONE', #8755, .T. ) ;
#3808=ORIENTED_EDGE ( 'NONE', *, *, #16385, .T. ) ;
#3809=ORIENTED_EDGE ( 'NONE', *, *, #17753, .T. ) ;
#3810=VECTOR ( 'NONE', #22162, 1000.000000000000000 ) ;
#3811=CARTESIAN_POINT ( 'NONE',  ( 172.7287565553229456, -4.999999999999970690, -33.50000000000000000 ) ) ;
#3813=CARTESIAN_POINT ( 'NONE',  ( 149.5152310637605808, -4.999999999999976907, -19.94844914048349693 ) ) ;
#3814=ORIENTED_EDGE ( 'NONE', *, *, #5212, .T. ) ;
#3818=ORIENTED_EDGE ( 'NONE', *, *, #21933, .T. ) ;
#3823=ADVANCED_FACE ( 'NONE', ( #18016 ), #13136, .T. ) ;
#3824=ORIENTED_EDGE ( 'NONE', *, *, #6947, .F. ) ;
#3828=VECTOR ( 'NONE', #18384, 1000.000000000000000 ) ;
#3830=CARTESIAN_POINT ( 'NONE',  ( 164.5152310637604955, -1.999999999999971356, -30.37205893520531319 ) ) ;
#3832=ORIENTED_EDGE ( 'NONE', *, *, #4124, .T. ) ;
#3833=CARTESIAN_POINT ( 'NONE',  ( 152.0152310637605524, -10.00000000000000000, -26.04193191628311155 ) ) ;
#3834=CARTESIAN_POINT ( 'NONE',  ( 129.5152310637605808, -10.00000000000000888, -19.94844914048349338 ) ) ;
#3836=ORIENTED_EDGE ( 'NONE', *, *, #1931, .F. ) ;
#3838=DIRECTION ( 'NONE',  ( 1.000000000000000000, 2.698458740408365879E-16, -1.110223024625156540E-16 ) ) ;
#3842=ORIENTED_EDGE ( 'NONE', *, *, #16064, .T. ) ;
#3843=LINE ( 'NONE', #29535, #4470 ) ;
#3846=CARTESIAN_POINT ( 'NONE',  ( 176.1922820468853388, -1.999999999999968470, -28.06379628232387802 ) ) ;
#3847=DIRECTION ( 'NONE',  ( 1.110223024625156540E-16, 2.995891024602366092E-32, 1.000000000000000000 ) ) ;
#3848=ORIENTED_EDGE ( 'NONE', *, *, #11792, .F. ) ;
#3849=DIRECTION ( 'NONE',  ( -0.8090169943749474513, -2.183098979609982436E-16, 0.5877852522924731371 ) ) ;
#3850=ORIENTED_EDGE ( 'NONE', *, *, #24493, .T. ) ;
#3852=AXIS2_PLACEMENT_3D ( 'NONE', #6310, #8435, #24626 ) ;
#3855=VERTEX_POINT ( 'NONE', #6583 ) ;
#3856=EDGE_CURVE ( 'NONE', #2318, #6495, #8703, .T. ) ;
#3859=ADVANCED_FACE ( 'NONE', ( #17563 ), #15871, .T. ) ;
#3860=CARTESIAN_POINT ( 'NONE',  ( 164.7287565553229740, -1.999999999999970912, -33.82050807568879947 ) ) ;
#3863=DIRECTION ( 'NONE',  ( -2.698458740408365879E-16, 1.000000000000000000, 0.000000000000000000 ) ) ;
#3866=ORIENTED_EDGE ( 'NONE', *, *, #11834, .T. ) ;
#3867=EDGE_LOOP ( 'NONE', ( #11348, #30172, #3454, #2533, #20063 ) ) ;
#3868=DIRECTION ( 'NONE',  ( -0.9510565162951536422, 0.000000000000000000, -0.3090169943749472292 ) ) ;
#3869=DIRECTION ( 'NONE',  ( 0.9510565162951536422, 0.000000000000000000, -0.3090169943749475623 ) ) ;
#3870=PLANE ( 'NONE',  #5051 ) ;
#3871=DIRECTION ( 'NONE',  ( -2.698458740408365879E-16, 1.000000000000000000, 0.000000000000000000 ) ) ;
#3873=DIRECTION ( 'NONE',  ( -1.110223024625156540E-16, 0.000000000000000000, -1.000000000000000000 ) ) ;
#3874=FACE_OUTER_BOUND ( 'NONE', #25916, .T. ) ;
#3879=EDGE_LOOP ( 'NONE', ( #12280, #21299, #25060, #4877, #29548 ) ) ;
#3880=CARTESIAN_POINT ( 'NONE',  ( 76.21670420379477662, -4.999999999999996447, 55.37467694846187527 ) ) ;
#3881=DIRECTION ( 'NONE',  ( -2.698458740408365879E-16, 1.000000000000000000, 0.000000000000000000 ) ) ;
#3882=VERTEX_POINT ( 'NONE', #11301 ) ;
#3884=CARTESIAN_POINT ( 'NONE',  ( 172.7287565553229740, -84.33034373659253902, -41.50000000000000711 ) ) ;
#3885=LINE ( 'NONE', #12573, #18048 ) ;
#3887=ORIENTED_EDGE ( 'NONE', *, *, #27588, .F. ) ;
#3888=ORIENTED_EDGE ( 'NONE', *, *, #11210, .F. ) ;
#3889=LINE ( 'NONE', #1755, #22253 ) ;
#3891=DIRECTION ( 'NONE',  ( 0.5877852522924731371, 0.000000000000000000, 0.8090169943749474513 ) ) ;
#3895=DIRECTION ( 'NONE',  ( -2.698458740408365879E-16, 1.000000000000000000, 0.000000000000000000 ) ) ;
#3898=ADVANCED_FACE ( 'NONE', ( #24598 ), #20604, .T. ) ;
#3899=CARTESIAN_POINT ( 'NONE',  ( 176.1922820468852535, -9.999999999999994671, -4.936203717676158398 ) ) ;
#3900=AXIS2_PLACEMENT_3D ( 'NONE', #6246, #8521, #17823 ) ;
#3904=ORIENTED_EDGE ( 'NONE', *, *, #11114, .T. ) ;
#3906=CARTESIAN_POINT ( 'NONE',  ( 154.7287565553229172, -4.999999999999976019, -16.50000000000000000 ) ) ;
#3909=LINE ( 'NONE', #4504, #23804 ) ;
#3910=DIRECTION ( 'NONE',  ( -0.9510565162951536422, -2.566386769018988816E-16, -0.3090169943749472292 ) ) ;
#3915=EDGE_CURVE ( 'NONE', #20048, #2560, #27070, .T. ) ;
#3917=VECTOR ( 'NONE', #16976, 1000.000000000000000 ) ;
#3918=LINE ( 'NONE', #3615, #18302 ) ;
#3920=VECTOR ( 'NONE', #13647, 1000.000000000000000 ) ;
#3922=CARTESIAN_POINT ( 'NONE',  ( 141.1922820468854525, -10.00000000000000533, -19.40354224447947473 ) ) ;
#3925=CARTESIAN_POINT ( 'NONE',  ( 137.0152310637605808, -4.999999999999980460, -1.521174642513229767E-14 ) ) ;
#3927=ORIENTED_EDGE ( 'NONE', *, *, #18941, .T. ) ;
#3928=FACE_OUTER_BOUND ( 'NONE', #13646, .T. ) ;
#3929=LINE ( 'NONE', #25134, #22475 ) ;
#3930=LINE ( 'NONE', #11087, #7824 ) ;
#3931=VERTEX_POINT ( 'NONE', #5977 ) ;
#3934=AXIS2_PLACEMENT_3D ( 'NONE', #11544, #581, #25760 ) ;
#3936=VECTOR ( 'NONE', #6769, 1000.000000000000000 ) ;
#3939=FACE_OUTER_BOUND ( 'NONE', #21966, .T. ) ;
#3944=DIRECTION ( 'NONE',  ( 0.9510565162951536422, 2.566386769018988816E-16, 0.3090169943749472292 ) ) ;
#3945=ORIENTED_EDGE ( 'NONE', *, *, #12796, .F. ) ;
#3947=ORIENTED_EDGE ( 'NONE', *, *, #10935, .F. ) ;
#3949=VECTOR ( 'NONE', #4963, 1000.000000000000000 ) ;
#3952=EDGE_CURVE ( 'NONE', #18704, #6853, #3843, .T. ) ;
#3954=EDGE_LOOP ( 'NONE', ( #24631, #30157, #16632, #3485, #1097 ) ) ;
#3955=VECTOR ( 'NONE', #24601, 1000.000000000000000 ) ;
#3958=EDGE_CURVE ( 'NONE', #26594, #27211, #25055, .T. ) ;
#3961=FACE_BOUND ( 'NONE', #43, .T. ) ;
#3962=ORIENTED_EDGE ( 'NONE', *, *, #16480, .T. ) ;
#3964=VERTEX_POINT ( 'NONE', #22764 ) ;
#3967=CARTESIAN_POINT ( 'NONE',  ( 147.0152310637605808, -4.999999999999977796, -15.61832212156129707 ) ) ;
#3969=ORIENTED_EDGE ( 'NONE', *, *, #6710, .T. ) ;
#3974=CARTESIAN_POINT ( 'NONE',  ( 137.0152310637605808, -10.00000000000000533, -34.70218595412750773 ) ) ;
#3975=VECTOR ( 'NONE', #9218, 1000.000000000000000 ) ;
#3976=AXIS2_PLACEMENT_3D ( 'NONE', #27570, #13480, #29741 ) ;
#3979=CARTESIAN_POINT ( 'NONE',  ( 167.0152310637604387, -9.999999999999998224, -8.721423840594312082 ) ) ;
#3980=ORIENTED_EDGE ( 'NONE', *, *, #19480, .F. ) ;
#3981=CARTESIAN_POINT ( 'NONE',  ( 171.1922820468853672, -1.999999999999970912, -28.06379628232387446 ) ) ;
#3982=EDGE_CURVE ( 'NONE', #11963, #12041, #13292, .T. ) ;
#3984=CARTESIAN_POINT ( 'NONE',  ( 152.2287565553229456, -10.00000000000000178, -3.509618943233403510 ) ) ;
#3987=EDGE_CURVE ( 'NONE', #8714, #30251, #13558, .T. ) ;
#3988=CARTESIAN_POINT ( 'NONE',  ( 144.5152310637605524, -10.00000000000000355, -13.05155085951651195 ) ) ;
#3993=DIRECTION ( 'NONE',  ( -2.698458740408365879E-16, 1.000000000000000000, 0.000000000000000000 ) ) ;
#3995=DIRECTION ( 'NONE',  ( -6.938893903907227392E-16, 0.000000000000000000, -1.000000000000000000 ) ) ;
#3996=DIRECTION ( 'NONE',  ( 2.698458740408365879E-16, -1.000000000000000000, 0.000000000000000000 ) ) ;
#3997=VERTEX_POINT ( 'NONE', #20868 ) ;
#3998=DIRECTION ( 'NONE',  ( -0.9510565162951536422, -2.566386769018988816E-16, -0.3090169943749472292 ) ) ;
#3999=ORIENTED_EDGE ( 'NONE', *, *, #2447, .F. ) ;
#4005=DIRECTION ( 'NONE',  ( -0.5877852522924731371, 0.000000000000000000, 0.8090169943749474513 ) ) ;
#4006=DIRECTION ( 'NONE',  ( -2.698458740408365879E-16, 1.000000000000000000, 0.000000000000000000 ) ) ;
#4010=VECTOR ( 'NONE', #20726, 1000.000000000000000 ) ;
#4011=VERTEX_POINT ( 'NONE', #27352 ) ;
#4012=LINE ( 'NONE', #13756, #9851 ) ;
#4013=DIRECTION ( 'NONE',  ( -0.8090169943749474513, -2.183098979609982436E-16, -0.5877852522924731371 ) ) ;
#4014=DIRECTION ( 'NONE',  ( -2.698458740408365879E-16, 1.000000000000000000, 0.000000000000000000 ) ) ;
#4015=CARTESIAN_POINT ( 'NONE',  ( 166.1922820468853388, -9.999999999999998224, -13.59645775552055902 ) ) ;
#4016=CARTESIAN_POINT ( 'NONE',  ( 131.1922820468854241, -10.00000000000000888, -10.74328820663507322 ) ) ;
#4017=VECTOR ( 'NONE', #29712, 1000.000000000000000 ) ;
#4019=CARTESIAN_POINT ( 'NONE',  ( 159.5152310637604387, -1.999999999999974021, -4.391296821672111328 ) ) ;
#4022=EDGE_CURVE ( 'NONE', #29656, #2898, #29959, .T. ) ;
#4026=PLANE ( 'NONE',  #9054 ) ;
#4030=VECTOR ( 'NONE', #3049, 1000.000000000000000 ) ;
#4031=CARTESIAN_POINT ( 'NONE',  ( 158.6922820468853672, -1.999999999999974021, -17.92658477444275889 ) ) ;
#4032=LINE ( 'NONE', #27272, #19022 ) ;
#4033=CARTESIAN_POINT ( 'NONE',  ( 171.1922820468853104, -1.999999999999970912, -10.74328820663507678 ) ) ;
#4035=ORIENTED_EDGE ( 'NONE', *, *, #1035, .T. ) ;
#4036=ORIENTED_EDGE ( 'NONE', *, *, #18299, .F. ) ;
#4037=LINE ( 'NONE', #25394, #14432 ) ;
#4040=FACE_OUTER_BOUND ( 'NONE', #26078, .T. ) ;
#4042=CARTESIAN_POINT ( 'NONE',  ( 159.7287565553229172, -10.00000000000000000, -7.839745962155603820 ) ) ;
#4044=ORIENTED_EDGE ( 'NONE', *, *, #21385, .F. ) ;
#4045=LINE ( 'NONE', #1768, #2767 ) ;
#4048=VECTOR ( 'NONE', #3051, 1000.000000000000000 ) ;
#4051=EDGE_LOOP ( 'NONE', ( #25843, #9045, #24810, #16363 ) ) ;
#4054=VECTOR ( 'NONE', #3944, 1000.000000000000000 ) ;
#4055=CARTESIAN_POINT ( 'NONE',  ( 131.1922820468854241, -1.999999999999981348, -28.06379628232387446 ) ) ;
#4056=ORIENTED_EDGE ( 'NONE', *, *, #8991, .T. ) ;
#4057=CARTESIAN_POINT ( 'NONE',  ( 162.0152310637605524, -1.999999999999971800, -32.93883019725009120 ) ) ;
#4058=CARTESIAN_POINT ( 'NONE',  ( 174.5152310637604671, -4.999999999999970690, -30.37205893520531319 ) ) ;
#4059=EDGE_CURVE ( 'NONE', #6652, #10981, #11553, .T. ) ;
#4063=EDGE_CURVE ( 'NONE', #17748, #21455, #20471, .T. ) ;
#4067=LINE ( 'NONE', #13360, #11957 ) ;
#4070=LINE ( 'NONE', #4216, #11971 ) ;
#4072=CARTESIAN_POINT ( 'NONE',  ( 134.5152310637605808, -1.999999999999980460, -2.627941064794695691 ) ) ;
#4076=ORIENTED_EDGE ( 'NONE', *, *, #7569, .F. ) ;
#4077=DIRECTION ( 'NONE',  ( 1.000000000000000000, 2.698458740408365879E-16, -1.110223024625156540E-16 ) ) ;
#4078=DIRECTION ( 'NONE',  ( -2.698458740408365879E-16, 1.000000000000000000, 0.000000000000000000 ) ) ;
#4079=DIRECTION ( 'NONE',  ( -2.698458740408365879E-16, 1.000000000000000000, 0.000000000000000000 ) ) ;
#4080=VECTOR ( 'NONE', #26669, 1000.000000000000000 ) ;
#4081=VERTEX_POINT ( 'NONE', #20423 ) ;
#4082=ORIENTED_EDGE ( 'NONE', *, *, #26433, .T. ) ;
#4087=LINE ( 'NONE', #29785, #6288 ) ;
#4088=DIRECTION ( 'NONE',  ( 0.5877852522924731371, 1.586114251531760728E-16, -0.8090169943749474513 ) ) ;
#4090=EDGE_CURVE ( 'NONE', #12211, #2375, #15838, .T. ) ;
#4092=EDGE_LOOP ( 'NONE', ( #27708, #21953, #17341, #22837, #17500 ) ) ;
#4094=LINE ( 'NONE', #17808, #20438 ) ;
#4095=ORIENTED_EDGE ( 'NONE', *, *, #21581, .F. ) ;
#4097=DIRECTION ( 'NONE',  ( -0.8090169943749474513, -2.183098979609982436E-16, -0.5877852522924731371 ) ) ;
#4098=VECTOR ( 'NONE', #11393, 1000.000000000000000 ) ;
#4100=CARTESIAN_POINT ( 'NONE',  ( 164.5152310637604671, -9.999999999999998224, -13.05155085951651195 ) ) ;
#4107=FACE_BOUND ( 'NONE', #26154, .T. ) ;
#4108=ORIENTED_EDGE ( 'NONE', *, *, #13246, .T. ) ;
#4109=VERTEX_POINT ( 'NONE', #16754 ) ;
#4110=DIRECTION ( 'NONE',  ( -2.698458740408365879E-16, 1.000000000000000000, -0.000000000000000000 ) ) ;
#4114=PLANE ( 'NONE',  #7657 ) ;
#4115=ORIENTED_EDGE ( 'NONE', *, *, #7121, .T. ) ;
#4117=VERTEX_POINT ( 'NONE', #23627 ) ;
#4121=AXIS2_PLACEMENT_3D ( 'NONE', #6841, #420, #13692 ) ;
#4123=EDGE_CURVE ( 'NONE', #28074, #22328, #26077, .T. ) ;
#4124=EDGE_CURVE ( 'NONE', #9369, #3213, #284, .T. ) ;
#4126=ORIENTED_EDGE ( 'NONE', *, *, #16829, .T. ) ;
#4127=VECTOR ( 'NONE', #4619, 1000.000000000000000 ) ;
#4129=LINE ( 'NONE', #25188, #18150 ) ;
#4133=LINE ( 'NONE', #29978, #16048 ) ;
#4134=ORIENTED_EDGE ( 'NONE', *, *, #11212, .T. ) ;
#4136=LINE ( 'NONE', #9, #13405 ) ;
#4137=VECTOR ( 'NONE', #1595, 1000.000000000000000 ) ;
#4140=CARTESIAN_POINT ( 'NONE',  ( 133.6922820468854241, -4.999999999999982236, -32.39392330124607611 ) ) ;
#4141=VERTEX_POINT ( 'NONE', #9874 ) ;
#4144=DIRECTION ( 'NONE',  ( -0.8090169943749474513, -2.183098979609982436E-16, -0.5877852522924731371 ) ) ;
#4145=ORIENTED_EDGE ( 'NONE', *, *, #1240, .F. ) ;
#4146=DIRECTION ( 'NONE',  ( -0.5877852522924731371, -1.586114251531760728E-16, -0.8090169943749474513 ) ) ;
#4147=ORIENTED_EDGE ( 'NONE', *, *, #14357, .F. ) ;
#4151=VERTEX_POINT ( 'NONE', #21173 ) ;
#4154=EDGE_CURVE ( 'NONE', #28443, #2968, #2434, .T. ) ;
#4156=EDGE_CURVE ( 'NONE', #280, #619, #132, .T. ) ;
#4159=VERTEX_POINT ( 'NONE', #13991 ) ;
#4161=EDGE_LOOP ( 'NONE', ( #2882, #13992, #391, #6242, #6168 ) ) ;
#4163=CARTESIAN_POINT ( 'NONE',  ( 25.15155720165195063, -5.000000000000010658, -77.40853353384594016 ) ) ;
#4164=LINE ( 'NONE', #13458, #6693 ) ;
#4165=CARTESIAN_POINT ( 'NONE',  ( 166.1922820468853672, -1.999999999999971356, -19.40354224447947828 ) ) ;
#4166=CARTESIAN_POINT ( 'NONE',  ( 144.7287565553230309, -10.00000000000000355, -16.50000000000000355 ) ) ;
#4168=CARTESIAN_POINT ( 'NONE',  ( 142.0152310637605524, -4.999999999999979572, -8.721423840594312082 ) ) ;
#4170=CARTESIAN_POINT ( 'NONE',  ( 168.6922820468853388, -1.999999999999971356, -17.92658477444275889 ) ) ;
#4171=VERTEX_POINT ( 'NONE', #588 ) ;
#4174=VECTOR ( 'NONE', #22383, 1000.000000000000000 ) ;
#4175=FACE_OUTER_BOUND ( 'NONE', #1570, .T. ) ;
#4177=DIRECTION ( 'NONE',  ( -1.110223024625156540E-16, 0.000000000000000000, -1.000000000000000000 ) ) ;
#4178=DIRECTION ( 'NONE',  ( 0.5877852522924731371, 1.586114251531760728E-16, -0.8090169943749474513 ) ) ;
#4180=ORIENTED_EDGE ( 'NONE', *, *, #14324, .F. ) ;
#4181=ORIENTED_EDGE ( 'NONE', *, *, #7200, .T. ) ;
#4182=DIRECTION ( 'NONE',  ( -2.698458740408365879E-16, 1.000000000000000000, 0.000000000000000000 ) ) ;
#4186=LINE ( 'NONE', #6029, #12235 ) ;
#4187=EDGE_LOOP ( 'NONE', ( #4230, #10530, #26158, #23284 ) ) ;
#4189=CARTESIAN_POINT ( 'NONE',  ( 136.1922820468854241, -1.999999999999980460, -22.25671179336495697 ) ) ;
#4191=ORIENTED_EDGE ( 'NONE', *, *, #13246, .F. ) ;
#4192=FACE_OUTER_BOUND ( 'NONE', #20337, .T. ) ;
#4195=ADVANCED_FACE ( 'NONE', ( #7594 ), #21029, .T. ) ;
#4198=EDGE_CURVE ( 'NONE', #6890, #11977, #25924, .T. ) ;
#4200=ORIENTED_EDGE ( 'NONE', *, *, #9236, .F. ) ;
#4202=AXIS2_PLACEMENT_3D ( 'NONE', #23588, #21139, #7263 ) ;
#4204=DIRECTION ( 'NONE',  ( 0.3090169943749472292, 8.338696094057992503E-17, -0.9510565162951536422 ) ) ;
#4205=LINE ( 'NONE', #8327, #1471 ) ;
#4206=LINE ( 'NONE', #25115, #6747 ) ;
#4207=LINE ( 'NONE', #27445, #27547 ) ;
#4214=VECTOR ( 'NONE', #30216, 1000.000000000000000 ) ;
#4215=DIRECTION ( 'NONE',  ( -2.698458740408365879E-16, 1.000000000000000000, 0.000000000000000000 ) ) ;
#4216=CARTESIAN_POINT ( 'NONE',  ( 133.7287565553229456, -4.000000000000003553, 8.500000000000003553 ) ) ;
#4218=DIRECTION ( 'NONE',  ( 0.9510565162951536422, 2.566386769018988816E-16, 0.3090169943749472292 ) ) ;
#4219=EDGE_LOOP ( 'NONE', ( #592, #19702, #1563, #16813 ) ) ;
#4220=LINE ( 'NONE', #29621, #18324 ) ;
#4222=ORIENTED_EDGE ( 'NONE', *, *, #9963, .T. ) ;
#4223=LINE ( 'NONE', #22999, #19793 ) ;
#4225=VECTOR ( 'NONE', #7313, 1000.000000000000000 ) ;
#4227=ORIENTED_EDGE ( 'NONE', *, *, #17622, .F. ) ;
#4230=ORIENTED_EDGE ( 'NONE', *, *, #20240, .T. ) ;
#4232=ADVANCED_FACE ( 'NONE', ( #25601 ), #23476, .T. ) ;
#4234=EDGE_CURVE ( 'NONE', #2172, #2945, #12011, .T. ) ;
#4235=CARTESIAN_POINT ( 'NONE',  ( 172.2287565553228887, -1.999999999999970024, -12.16987298107780369 ) ) ;
#4236=ADVANCED_FACE ( 'NONE', ( #3038 ), #21326, .T. ) ;
#4238=VECTOR ( 'NONE', #7975, 1000.000000000000000 ) ;
#4239=ORIENTED_EDGE ( 'NONE', *, *, #18884, .T. ) ;
#4240=LINE ( 'NONE', #21152, #14271 ) ;
#4241=CARTESIAN_POINT ( 'NONE',  ( 172.0152310637604671, -4.999999999999970690, -26.04193191628311155 ) ) ;
#4242=ORIENTED_EDGE ( 'NONE', *, *, #10480, .F. ) ;
#4244=DIRECTION ( 'NONE',  ( -0.8090169943749474513, -2.183098979609982436E-16, -0.5877852522924731371 ) ) ;
#4245=VECTOR ( 'NONE', #14961, 999.9999999999998863 ) ;
#4247=ORIENTED_EDGE ( 'NONE', *, *, #20819, .F. ) ;
#4248=CARTESIAN_POINT ( 'NONE',  ( 149.5152310637606092, -10.00000000000000178, -28.60870317832789667 ) ) ;
#4252=VERTEX_POINT ( 'NONE', #9263 ) ;
#4254=DIRECTION ( 'NONE',  ( -2.698458740408365879E-16, 1.000000000000000000, 0.000000000000000000 ) ) ;
#4256=CARTESIAN_POINT ( 'NONE',  ( 142.0152310637605808, -10.00000000000000355, -17.38167787843871182 ) ) ;
#4258=DIRECTION ( 'NONE',  ( 0.9510565162951536422, 0.000000000000000000, -0.3090169943749475623 ) ) ;
#4261=CARTESIAN_POINT ( 'NONE',  ( 105.8449596982085836, -4.999999999999988454, -76.90086459576200184 ) ) ;
#4262=EDGE_LOOP ( 'NONE', ( #482, #26047, #14335, #26472, #19065 ) ) ;
#4263=ORIENTED_EDGE ( 'NONE', *, *, #23252, .F. ) ;
#4264=CARTESIAN_POINT ( 'NONE',  ( 97.96609169890469104, -4.999999999999991118, 71.17653192172720367 ) ) ;
#4265=ORIENTED_EDGE ( 'NONE', *, *, #22032, .F. ) ;
#4267=AXIS2_PLACEMENT_3D ( 'NONE', #7829, #24166, #5696 ) ;
#4270=EDGE_LOOP ( 'NONE', ( #27964, #4375, #10250, #2763 ) ) ;
#4272=CARTESIAN_POINT ( 'NONE',  ( 166.1922820468853672, -4.999999999999972466, -28.06379628232387802 ) ) ;
#4273=CYLINDRICAL_SURFACE ( 'NONE', #5951, 3.000000000000002665 ) ;
#4274=EDGE_CURVE ( 'NONE', #19861, #4517, #18590, .T. ) ;
#4276=DIRECTION ( 'NONE',  ( -0.8090169943749474513, -2.183098979609982436E-16, 0.5877852522924731371 ) ) ;
#4277=DIRECTION ( 'NONE',  ( 0.9510565162951535312, 2.566386769018988816E-16, -0.3090169943749475623 ) ) ;
#4278=VECTOR ( 'NONE', #20908, 1000.000000000000000 ) ;
#4279=EDGE_LOOP ( 'NONE', ( #8590, #23241, #26425, #4448, #7928 ) ) ;
#4280=DIRECTION ( 'NONE',  ( -2.698458740408365879E-16, 1.000000000000000000, 0.000000000000000000 ) ) ;
#4281=DIRECTION ( 'NONE',  ( -2.698458740408365879E-16, 1.000000000000000000, 0.000000000000000000 ) ) ;
#4282=CARTESIAN_POINT ( 'NONE',  ( 148.6922820468853672, -10.00000000000000355, 2.247092850131519715 ) ) ;
#4283=VECTOR ( 'NONE', #20313, 1000.000000000000000 ) ;
#4284=ORIENTED_EDGE ( 'NONE', *, *, #18689, .F. ) ;
#4286=CARTESIAN_POINT ( 'NONE',  ( 130.7287565553229456, -4.999999999999983125, 3.500000000000003109 ) ) ;
#4290=ADVANCED_FACE ( 'NONE', ( #5766 ), #12617, .T. ) ;
#4291=VERTEX_POINT ( 'NONE', #17648 ) ;
#4293=VERTEX_POINT ( 'NONE', #21934 ) ;
#4294=DIRECTION ( 'NONE',  ( -0.8090169943749474513, -2.183098979609982436E-16, -0.5877852522924731371 ) ) ;
#4296=CARTESIAN_POINT ( 'NONE',  ( 161.1922820468853388, -9.999999999999998224, -10.74328820663507678 ) ) ;
#4297=CARTESIAN_POINT ( 'NONE',  ( 159.5152310637604387, -1.999999999999974021, -4.391296821672111328 ) ) ;
#4298=ORIENTED_EDGE ( 'NONE', *, *, #28149, .F. ) ;
#4299=CARTESIAN_POINT ( 'NONE',  ( 127.7287565553229598, -1.999999999999982681, -33.50000000000000000 ) ) ;
#4304=VECTOR ( 'NONE', #27271, 1000.000000000000000 ) ;
#4308=VECTOR ( 'NONE', #29668, 999.9999999999998863 ) ;
#4310=VERTEX_POINT ( 'NONE', #29000 ) ;
#4311=LINE ( 'NONE', #20928, #2577 ) ;
#4314=CARTESIAN_POINT ( 'NONE',  ( 163.6922820468853672, -1.999999999999972244, -26.58683881228715862 ) ) ;
#4316=DIRECTION ( 'NONE',  ( -2.698458740408365879E-16, 1.000000000000000000, 0.000000000000000000 ) ) ;
#4318=EDGE_CURVE ( 'NONE', #5150, #6558, #3479, .T. ) ;
#4319=AXIS2_PLACEMENT_3D ( 'NONE', #7754, #17063, #26391 ) ;
#4321=VERTEX_POINT ( 'NONE', #29148 ) ;
#4323=EDGE_CURVE ( 'NONE', #17861, #8041, #5461, .T. ) ;
#4325=LINE ( 'NONE', #23245, #3936 ) ;
#4326=CARTESIAN_POINT ( 'NONE',  ( 98.45422169453954098, -4.999999999999990230, -71.53117912275099854 ) ) ;
#4327=EDGE_CURVE ( 'NONE', #10549, #28746, #1347, .T. ) ;
#4329=EDGE_LOOP ( 'NONE', ( #16127, #13012, #24777, #7957 ) ) ;
#4332=LINE ( 'NONE', #27278, #22744 ) ;
#4334=VECTOR ( 'NONE', #17777, 1000.000000000000000 ) ;
#4336=CARTESIAN_POINT ( 'NONE',  ( 137.0152310637605524, -4.999999999999980460, -1.521174642513229451E-14 ) ) ;
#4338=FACE_OUTER_BOUND ( 'NONE', #23479, .T. ) ;
#4340=VERTEX_POINT ( 'NONE', #6065 ) ;
#4341=DIRECTION ( 'NONE',  ( -2.698458740408365879E-16, 1.000000000000000000, 0.000000000000000000 ) ) ;
#4342=( NAMED_UNIT ( * ) SI_UNIT ( $, .STERADIAN. ) SOLID_ANGLE_UNIT ( ) );
#4346=ORIENTED_EDGE ( 'NONE', *, *, #1277, .F. ) ;
#4347=CARTESIAN_POINT ( 'NONE',  ( 169.5152310637605240, -9.999999999999994671, -28.60870317832789667 ) ) ;
#4348=VECTOR ( 'NONE', #9477, 1000.000000000000000 ) ;
#4352=CARTESIAN_POINT ( 'NONE',  ( 107.5362657617971820, -4.999999999999988454, -78.12967037883245780 ) ) ;
#4355=CARTESIAN_POINT ( 'NONE',  ( 167.0152310637604387, -1.999999999999972244, 1.702185954127501066 ) ) ;
#4358=EDGE_CURVE ( 'NONE', #22694, #2461, #15203, .T. ) ;
#4361=EDGE_CURVE ( 'NONE', #29222, #4117, #10634, .T. ) ;
#4362=EDGE_CURVE ( 'NONE', #16946, #16967, #19944, .T. ) ;
#4364=PLANE ( 'NONE',  #29591 ) ;
#4365=ADVANCED_FACE ( 'NONE', ( #15352 ), #15048, .T. ) ;
#4367=LINE ( 'NONE', #29918, #25349 ) ;
#4368=ORIENTED_EDGE ( 'NONE', *, *, #9964, .T. ) ;
#4369=LINE ( 'NONE', #13670, #26633 ) ;
#4371=VERTEX_POINT ( 'NONE', #28859 ) ;
#4373=DIRECTION ( 'NONE',  ( 0.9510565162951535312, 2.566386769018988816E-16, -0.3090169943749475623 ) ) ;
#4374=LINE ( 'NONE', #24996, #18052 ) ;
#4375=ORIENTED_EDGE ( 'NONE', *, *, #20770, .F. ) ;
#4376=FACE_OUTER_BOUND ( 'NONE', #7178, .T. ) ;
#4378=VECTOR ( 'NONE', #11391, 1000.000000000000000 ) ;
#4384=VERTEX_POINT ( 'NONE', #14894 ) ;
#4391=EDGE_LOOP ( 'NONE', ( #13774, #20993, #1262, #3346, #16201 ) ) ;
#4392=ORIENTED_EDGE ( 'NONE', *, *, #25112, .T. ) ;
#4394=DIRECTION ( 'NONE',  ( -0.9510565162951536422, -2.566386769018988816E-16, -0.3090169943749472292 ) ) ;
#4395=VECTOR ( 'NONE', #13833, 1000.000000000000000 ) ;
#4397=ORIENTED_EDGE ( 'NONE', *, *, #2348, .F. ) ;
#4400=EDGE_LOOP ( 'NONE', ( #4498, #8803, #25683, #21105 ) ) ;
#4401=EDGE_CURVE ( 'NONE', #22420, #8035, #12919, .T. ) ;
#4404=DIRECTION ( 'NONE',  ( -2.698458740408365879E-16, 1.000000000000000000, 0.000000000000000000 ) ) ;
#4405=ADVANCED_FACE ( 'NONE', ( #7895 ), #724, .T. ) ;
#4407=LINE ( 'NONE', #27193, #3389 ) ;
#4408=EDGE_CURVE ( 'NONE', #3548, #22258, #3336, .T. ) ;
#4409=PLANE ( 'NONE',  #1822 ) ;
#4410=AXIS2_PLACEMENT_3D ( 'NONE', #29847, #8853, #18167 ) ;
#4411=ORIENTED_EDGE ( 'NONE', *, *, #24280, .F. ) ;
#4412=VECTOR ( 'NONE', #12874, 1000.000000000000000 ) ;
#4413=CARTESIAN_POINT ( 'NONE',  ( 139.7287565553230024, -10.00000000000000533, 0.8205080756887930260 ) ) ;
#4415=EDGE_LOOP ( 'NONE', ( #19865, #7183, #11633, #28782 ) ) ;
#4418=VERTEX_POINT ( 'NONE', #24382 ) ;
#4424=LINE ( 'NONE', #23045, #6936 ) ;
#4426=DIRECTION ( 'NONE',  ( -2.698458740408365879E-16, 1.000000000000000000, 0.000000000000000000 ) ) ;
#4427=AXIS2_PLACEMENT_3D ( 'NONE', #20098, #27758, #15665 ) ;
#4428=DIRECTION ( 'NONE',  ( -2.698458740408366372E-16, 1.000000000000000000, 0.000000000000000000 ) ) ;
#4429=VECTOR ( 'NONE', #12918, 1000.000000000000000 ) ;
#4434=ORIENTED_EDGE ( 'NONE', *, *, #26971, .T. ) ;
#4440=CARTESIAN_POINT ( 'NONE',  ( 174.5152310637604387, -1.999999999999969358, -21.71180489736091346 ) ) ;
#4441=ADVANCED_FACE ( 'NONE', ( #4376 ), #10790, .T. ) ;
#4442=ORIENTED_EDGE ( 'NONE', *, *, #8692, .T. ) ;
#4443=ORIENTED_EDGE ( 'NONE', *, *, #22460, .T. ) ;
#4448=ORIENTED_EDGE ( 'NONE', *, *, #27732, .T. ) ;
#4449=EDGE_LOOP ( 'NONE', ( #23196, #28449, #29700, #23102, #15467 ) ) ;
#4450=DIRECTION ( 'NONE',  ( -0.5877852522924731371, -1.586114251531760728E-16, -0.8090169943749474513 ) ) ;
#4451=EDGE_LOOP ( 'NONE', ( #14119, #19459, #2931, #19006 ) ) ;
#4454=ORIENTED_EDGE ( 'NONE', *, *, #14324, .T. ) ;
#4456=VECTOR ( 'NONE', #7861, 1000.000000000000000 ) ;
#4458=LINE ( 'NONE', #2780, #15973 ) ;
#4459=DIRECTION ( 'NONE',  ( -2.698458740408365879E-16, 1.000000000000000000, 0.000000000000000000 ) ) ;
#4463=ORIENTED_EDGE ( 'NONE', *, *, #16308, .F. ) ;
#4464=ORIENTED_EDGE ( 'NONE', *, *, #15971, .F. ) ;
#4465=EDGE_CURVE ( 'NONE', #9448, #1955, #8640, .T. ) ;
#4466=DIRECTION ( 'NONE',  ( -2.698458740408365879E-16, 1.000000000000000000, 0.000000000000000000 ) ) ;
#4469=LINE ( 'NONE', #13759, #452 ) ;
#4470=VECTOR ( 'NONE', #1873, 1000.000000000000000 ) ;
#4471=CARTESIAN_POINT ( 'NONE',  ( 14.01590296442413397, -5.000000000000014211, -43.13651381225401593 ) ) ;
#4472=ADVANCED_FACE ( 'NONE', ( #11380 ), #2104, .T. ) ;
#4475=ORIENTED_EDGE ( 'NONE', *, *, #19340, .F. ) ;
#4480=CARTESIAN_POINT ( 'NONE',  ( 158.6922820468853956, -1.999999999999973133, -23.73366926340167637 ) ) ;
#4481=DIRECTION ( 'NONE',  ( 0.9510565162951536422, 2.566386769018988816E-16, 0.3090169943749472292 ) ) ;
#4482=DIRECTION ( 'NONE',  ( -0.9510565162951536422, -2.566386769018988816E-16, -0.3090169943749472292 ) ) ;
#4483=EDGE_LOOP ( 'NONE', ( #18513, #16334, #16487, #12207 ) ) ;
#4485=DIRECTION ( 'NONE',  ( -2.698458740408365879E-16, 1.000000000000000000, 0.000000000000000000 ) ) ;
#4489=CARTESIAN_POINT ( 'NONE',  ( 171.1922820468853104, -9.999999999999996447, -13.59645775552055902 ) ) ;
#4490=CARTESIAN_POINT ( 'NONE',  ( 104.9340031866765344, -4.999999999999988454, 76.23901594897056100 ) ) ;
#4491=VECTOR ( 'NONE', #1130, 1000.000000000000000 ) ;
#4493=EDGE_LOOP ( 'NONE', ( #12397, #10329, #21160, #18160 ) ) ;
#4495=SURFACE_SIDE_STYLE ('',( #18072 ) ) ;
#4498=ORIENTED_EDGE ( 'NONE', *, *, #8284, .T. ) ;
#4499=EDGE_CURVE ( 'NONE', #11139, #22675, #6820, .T. ) ;
#4501=ADVANCED_FACE ( 'NONE', ( #27156 ), #6519, .T. ) ;
#4502=DIRECTION ( 'NONE',  ( 0.9510565162951536422, 0.000000000000000000, -0.3090169943749475623 ) ) ;
#4503=DIRECTION ( 'NONE',  ( -0.8090169943749474513, -2.183098979609982436E-16, 0.5877852522924731371 ) ) ;
#4504=CARTESIAN_POINT ( 'NONE',  ( 164.5152310637604671, -4.999999999999973355, -1.826485974285146553E-14 ) ) ;
#4505=CARTESIAN_POINT ( 'NONE',  ( 176.1922820468853388, -9.999999999999994671, -28.06379628232387802 ) ) ;
#4507=LINE ( 'NONE', #22535, #26779 ) ;
#4513=CARTESIAN_POINT ( 'NONE',  ( 168.6922820468853388, -1.999999999999970912, -15.07341522555727664 ) ) ;
#4514=DIRECTION ( 'NONE',  ( -0.5877852522924731371, -1.586114251531760728E-16, -0.8090169943749474513 ) ) ;
#4516=ORIENTED_EDGE ( 'NONE', *, *, #20817, .T. ) ;
#4517=VERTEX_POINT ( 'NONE', #29475 ) ;
#4518=LINE ( 'NONE', #1793, #3721 ) ;
#4520=ORIENTED_EDGE ( 'NONE', *, *, #10904, .T. ) ;
#4522=FACE_OUTER_BOUND ( 'NONE', #52, .T. ) ;
#4523=AXIS2_PLACEMENT_3D ( 'NONE', #18153, #29674, #27513 ) ;
#4526=ORIENTED_EDGE ( 'NONE', *, *, #4631, .F. ) ;
#4531=VECTOR ( 'NONE', #29792, 1000.000000000000000 ) ;
#4532=LINE ( 'NONE', #5246, #23531 ) ;
#4534=EDGE_CURVE ( 'NONE', #12234, #22051, #24997, .T. ) ;
#4535=EDGE_CURVE ( 'NONE', #27081, #14637, #20683, .T. ) ;
#4536=VERTEX_POINT ( 'NONE', #22852 ) ;
#4537=EDGE_CURVE ( 'NONE', #28890, #29995, #11236, .T. ) ;
#4538=CARTESIAN_POINT ( 'NONE',  ( 137.0152310637605808, -10.00000000000000533, 1.702185954127501066 ) ) ;
#4540=EDGE_LOOP ( 'NONE', ( #10859, #19017, #15432, #25172 ) ) ;
#4546=ORIENTED_EDGE ( 'NONE', *, *, #11285, .F. ) ;
#4547=VECTOR ( 'NONE', #6004, 1000.000000000000000 ) ;
#4548=DIRECTION ( 'NONE',  ( 1.000000000000000000, 2.698458740408365879E-16, -1.110223024625156540E-16 ) ) ;
#4549=LINE ( 'NONE', #27632, #22098 ) ;
#4551=FACE_BOUND ( 'NONE', #21761, .T. ) ;
#4552=ORIENTED_EDGE ( 'NONE', *, *, #26866, .T. ) ;
#4553=LINE ( 'NONE', #9108, #1333 ) ;
#4554=VERTEX_POINT ( 'NONE', #6669 ) ;
#4555=PLANE ( 'NONE',  #17335 ) ;
#4558=CARTESIAN_POINT ( 'NONE',  ( 143.6922820468854525, -10.00000000000000355, -35.24709285013155835 ) ) ;
#4559=VERTEX_POINT ( 'NONE', #22553 ) ;
#4563=ORIENTED_EDGE ( 'NONE', *, *, #2859, .T. ) ;
#4565=DIRECTION ( 'NONE',  ( 0.5877852522924731371, 0.000000000000000000, 0.8090169943749474513 ) ) ;
#4567=DIRECTION ( 'NONE',  ( 1.000000000000000000, 2.891205793294675861E-16, 0.000000000000000000 ) ) ;
#4569=ADVANCED_FACE ( 'NONE', ( #25135 ), #24842, .T. ) ;
#4571=ADVANCED_FACE ( 'NONE', ( #13373 ), #1802, .T. ) ;
#4572=EDGE_CURVE ( 'NONE', #8702, #1753, #3930, .T. ) ;
#4573=CARTESIAN_POINT ( 'NONE',  ( 139.5152310637605808, -1.999999999999978684, -30.37205893520530964 ) ) ;
#4575=DIRECTION ( 'NONE',  ( -0.5877852522924731371, -1.586114251531760728E-16, -0.8090169943749474513 ) ) ;
#4576=DIRECTION ( 'NONE',  ( 1.110223024625156540E-16, 2.995891024602366092E-32, 1.000000000000000000 ) ) ;
#4578=LINE ( 'NONE', #13867, #12860 ) ;
#4581=DIRECTION ( 'NONE',  ( 0.3090169943749472292, 8.338696094057992503E-17, -0.9510565162951536422 ) ) ;
#4584=ORIENTED_EDGE ( 'NONE', *, *, #6778, .F. ) ;
#4585=DIRECTION ( 'NONE',  ( 1.110223024625156540E-16, 2.995891024602366092E-32, 1.000000000000000000 ) ) ;
#4589=ORIENTED_EDGE ( 'NONE', *, *, #12510, .T. ) ;
#4590=ORIENTED_EDGE ( 'NONE', *, *, #5811, .T. ) ;
#4592=VECTOR ( 'NONE', #17190, 1000.000000000000000 ) ;
#4594=DIRECTION ( 'NONE',  ( -0.5877852522924731371, 0.000000000000000000, 0.8090169943749474513 ) ) ;
#4595=CARTESIAN_POINT ( 'NONE',  ( 172.2287565553228603, -9.999999999999996447, -3.509618943233403510 ) ) ;
#4597=DIRECTION ( 'NONE',  ( -2.698458740408365879E-16, 1.000000000000000000, 0.000000000000000000 ) ) ;
#4600=EDGE_CURVE ( 'NONE', #12211, #6477, #20119, .T. ) ;
#4603=ORIENTED_EDGE ( 'NONE', *, *, #14358, .F. ) ;
#4604=FACE_OUTER_BOUND ( 'NONE', #16842, .T. ) ;
#4605=LINE ( 'NONE', #18184, #8375 ) ;
#4609=EDGE_CURVE ( 'NONE', #7377, #12234, #15831, .T. ) ;
#4610=ADVANCED_FACE ( 'NONE', ( #26070 ), #23160, .T. ) ;
#4611=EDGE_CURVE ( 'NONE', #29985, #2754, #16747, .T. ) ;
#4612=ORIENTED_EDGE ( 'NONE', *, *, #29568, .T. ) ;
#4613=DIRECTION ( 'NONE',  ( -2.698458740408365879E-16, 1.000000000000000000, 0.000000000000000000 ) ) ;
#4614=AXIS2_PLACEMENT_3D ( 'NONE', #2267, #16431, #20700 ) ;
#4615=DIRECTION ( 'NONE',  ( 0.5877852522924731371, 1.586114251531760728E-16, 0.8090169943749474513 ) ) ;
#4616=DIRECTION ( 'NONE',  ( -2.698458740408365879E-16, 1.000000000000000000, 0.000000000000000000 ) ) ;
#4619=DIRECTION ( 'NONE',  ( -2.698458740408365879E-16, 1.000000000000000000, 0.000000000000000000 ) ) ;
#4620=DIRECTION ( 'NONE',  ( -1.110223024625156540E-16, 0.000000000000000000, -1.000000000000000000 ) ) ;
#4624=CARTESIAN_POINT ( 'NONE',  ( 147.2287565553230309, -1.999999999999976241, -20.83012701892220520 ) ) ;
#4628=ORIENTED_EDGE ( 'NONE', *, *, #25839, .F. ) ;
#4629=DIRECTION ( 'NONE',  ( 0.9510565162951536422, 2.566386769018988816E-16, 0.3090169943749472292 ) ) ;
#4631=EDGE_CURVE ( 'NONE', #23086, #4159, #5145, .T. ) ;
#4632=EDGE_LOOP ( 'NONE', ( #8031, #6777, #17058, #3627 ) ) ;
#4634=PLANE ( 'NONE',  #25901 ) ;
#4635=VECTOR ( 'NONE', #20043, 1000.000000000000000 ) ;
#4636=DIRECTION ( 'NONE',  ( -0.9510565162951536422, -2.566386769018988816E-16, -0.3090169943749472292 ) ) ;
#4638=ORIENTED_EDGE ( 'NONE', *, *, #25417, .T. ) ;
#4643=EDGE_CURVE ( 'NONE', #24422, #5460, #27933, .T. ) ;
#4644=EDGE_LOOP ( 'NONE', ( #11937, #14628, #193, #8461 ) ) ;
#4645=CARTESIAN_POINT ( 'NONE',  ( 172.7287565553229740, -84.33034373659253902, 0.5000000000000029976 ) ) ;
#4646=PLANE ( 'NONE',  #11850 ) ;
#4647=FACE_OUTER_BOUND ( 'NONE', #20785, .T. ) ;
#4648=DIRECTION ( 'NONE',  ( -0.8090169943749474513, -2.183098979609982436E-16, 0.5877852522924731371 ) ) ;
#4654=EDGE_LOOP ( 'NONE', ( #1947, #10487, #21648, #23003 ) ) ;
#4655=CARTESIAN_POINT ( 'NONE',  ( 133.7287565553229456, -4.999999999999982236, 3.500000000000003109 ) ) ;
#4656=DIRECTION ( 'NONE',  ( 0.3090169943749475623, 8.338696094058001131E-17, 0.9510565162951536422 ) ) ;
#4657=CARTESIAN_POINT ( 'NONE',  ( 162.0152310637604671, -9.999999999999998224, -17.38167787843871182 ) ) ;
#4659=CARTESIAN_POINT ( 'NONE',  ( 156.1922820468853388, -4.999999999999976019, -4.936203717676158398 ) ) ;
#4661=VECTOR ( 'NONE', #20378, 1000.000000000000000 ) ;
#4663=ADVANCED_FACE ( 'NONE', ( #16436 ), #2277, .T. ) ;
#4664=ORIENTED_EDGE ( 'NONE', *, *, #30029, .F. ) ;
#4665=CARTESIAN_POINT ( 'NONE',  ( 134.5152310637605524, -10.00000000000000533, -13.05155085951650840 ) ) ;
#4666=DIRECTION ( 'NONE',  ( 0.3090169943749472292, 8.338696094057992503E-17, -0.9510565162951536422 ) ) ;
#4670=VERTEX_POINT ( 'NONE', #14437 ) ;
#4671=ORIENTED_EDGE ( 'NONE', *, *, #1971, .T. ) ;
#4674=AXIS2_PLACEMENT_3D ( 'NONE', #15161, #1457, #3153 ) ;
#4677=ORIENTED_EDGE ( 'NONE', *, *, #19141, .T. ) ;
#4678=DIRECTION ( 'NONE',  ( -2.698458740408365879E-16, 1.000000000000000000, 0.000000000000000000 ) ) ;
#4680=ORIENTED_EDGE ( 'NONE', *, *, #29006, .T. ) ;
#4681=DIRECTION ( 'NONE',  ( -0.8090169943749474513, -2.183098979609982436E-16, -0.5877852522924731371 ) ) ;
#4683=DIRECTION ( 'NONE',  ( 0.3090169943749472292, 8.338696094057992503E-17, -0.9510565162951536422 ) ) ;
#4685=VECTOR ( 'NONE', #3695, 1000.000000000000000 ) ;
#4687=VERTEX_POINT ( 'NONE', #6993 ) ;
#4692=CARTESIAN_POINT ( 'NONE',  ( 167.0152310637604671, -9.999999999999998224, -6.958068083716895558 ) ) ;
#4694=ADVANCED_FACE ( 'NONE', ( #2425 ), #11702, .T. ) ;
#4695=ORIENTED_EDGE ( 'NONE', *, *, #28646, .T. ) ;
#4696=CARTESIAN_POINT ( 'NONE',  ( 149.7287565553229740, -10.00000000000000178, -7.839745962155603820 ) ) ;
#4697=EDGE_CURVE ( 'NONE', #23239, #19711, #275, .T. ) ;
#4699=EDGE_CURVE ( 'NONE', #24045, #23305, #21471, .T. ) ;
#4700=ORIENTED_EDGE ( 'NONE', *, *, #14059, .F. ) ;
#4701=FACE_OUTER_BOUND ( 'NONE', #27171, .T. ) ;
#4706=VERTEX_POINT ( 'NONE', #28236 ) ;
#4709=CARTESIAN_POINT ( 'NONE',  ( 23.64023604348281893, -5.000000000000011546, -72.75716528596417731 ) ) ;
#4711=LINE ( 'NONE', #19052, #14228 ) ;
#4712=AXIS2_PLACEMENT_3D ( 'NONE', #30144, #11897, #4597 ) ;
#4714=EDGE_LOOP ( 'NONE', ( #6279, #5406, #28251, #28461 ) ) ;
#4715=DIRECTION ( 'NONE',  ( -2.698458740408365879E-16, 1.000000000000000000, 0.000000000000000000 ) ) ;
#4716=DIRECTION ( 'NONE',  ( -0.7071067811865460184, -0.7071067811865490160, -0.000000000000000000 ) ) ;
#4719=CARTESIAN_POINT ( 'NONE',  ( 138.6922820468854525, -10.00000000000000533, -9.266330736598359152 ) ) ;
#4721=DIRECTION ( 'NONE',  ( 0.5877852522924731371, 0.000000000000000000, 0.8090169943749474513 ) ) ;
#4722=FACE_OUTER_BOUND ( 'NONE', #2027, .T. ) ;
#4725=ORIENTED_EDGE ( 'NONE', *, *, #15479, .T. ) ;
#4727=VECTOR ( 'NONE', #28775, 1000.000000000000000 ) ;
#4730=DIRECTION ( 'NONE',  ( 0.9510565162951536422, 2.566386769018988816E-16, 0.3090169943749472292 ) ) ;
#4732=ADVANCED_FACE ( 'NONE', ( #14284 ), #7290, .T. ) ;
#4733=ORIENTED_EDGE ( 'NONE', *, *, #17446, .F. ) ;
#4734=VECTOR ( 'NONE', #1310, 1000.000000000000000 ) ;
#4736=CARTESIAN_POINT ( 'NONE',  ( 151.1922820468854241, -1.999999999999975353, -19.40354224447947828 ) ) ;
#4737=EDGE_CURVE ( 'NONE', #26487, #5681, #21316, .T. ) ;
#4739=LINE ( 'NONE', #23069, #7843 ) ;
#4740=LINE ( 'NONE', #23823, #13990 ) ;
#4744=EDGE_LOOP ( 'NONE', ( #11353, #13537, #14566, #10646, #473 ) ) ;
#4746=ORIENTED_EDGE ( 'NONE', *, *, #13724, .F. ) ;
#4752=CARTESIAN_POINT ( 'NONE',  ( 157.0152310637604671, -4.999999999999975131, -8.721423840594312082 ) ) ;
#4756=VECTOR ( 'NONE', #10057, 1000.000000000000000 ) ;
#4757=ORIENTED_EDGE ( 'NONE', *, *, #18036, .T. ) ;
#4758=FACE_BOUND ( 'NONE', #25990, .T. ) ;
#4759=AXIS2_PLACEMENT_3D ( 'NONE', #12061, #27989, #5050 ) ;
#4761=VECTOR ( 'NONE', #23688, 1000.000000000000000 ) ;
#4763=DIRECTION ( 'NONE',  ( -2.698458740408365879E-16, 1.000000000000000000, 0.000000000000000000 ) ) ;
#4765=DIRECTION ( 'NONE',  ( -0.9510565162951536422, -2.566386769018988816E-16, -0.3090169943749472292 ) ) ;
#4768=ORIENTED_EDGE ( 'NONE', *, *, #21340, .F. ) ;
#4770=ORIENTED_EDGE ( 'NONE', *, *, #18063, .F. ) ;
#4771=EDGE_CURVE ( 'NONE', #20749, #25811, #19033, .T. ) ;
#4772=ADVANCED_FACE ( 'NONE', ( #4994 ), #25457, .T. ) ;
#4773=AXIS2_PLACEMENT_3D ( 'NONE', #8021, #15645, #24977 ) ;
#4775=DIRECTION ( 'NONE',  ( 1.110223024625156540E-16, 2.995891024602366092E-32, 1.000000000000000000 ) ) ;
#4777=EDGE_CURVE ( 'NONE', #28404, #26171, #3327, .T. ) ;
#4781=CARTESIAN_POINT ( 'NONE',  ( 180.7287565553229456, -9.999999999999968026, 0.5000000000000029976 ) ) ;
#4782=ADVANCED_FACE ( 'NONE', ( #15039 ), #5910, .T. ) ;
#4784=AXIS2_PLACEMENT_3D ( 'NONE', #6748, #22623, #16038 ) ;
#4787=CARTESIAN_POINT ( 'NONE',  ( 146.1922820468854525, -10.00000000000000178, -28.06379628232387446 ) ) ;
#4789=ORIENTED_EDGE ( 'NONE', *, *, #24738, .F. ) ;
#4793=ORIENTED_EDGE ( 'NONE', *, *, #26532, .T. ) ;
#4794=DIRECTION ( 'NONE',  ( 0.9510565162951536422, 0.000000000000000000, -0.3090169943749475623 ) ) ;
#4796=CARTESIAN_POINT ( 'NONE',  ( 139.5152310637605808, -4.999999999999980460, -21.71180489736090991 ) ) ;
#4798=AXIS2_PLACEMENT_3D ( 'NONE', #28549, #7601, #29008 ) ;
#4799=LINE ( 'NONE', #6390, #8802 ) ;
#4800=CARTESIAN_POINT ( 'NONE',  ( 133.6922820468854241, -10.00000000000000711, -26.58683881228715506 ) ) ;
#4802=VECTOR ( 'NONE', #24698, 1000.000000000000000 ) ;
#4806=DIRECTION ( 'NONE',  ( -0.9510565162951536422, -2.566386769018988323E-16, 0.3090169943749475623 ) ) ;
#4808=CARTESIAN_POINT ( 'NONE',  ( 154.5152310637605240, -10.00000000000000000, -11.28819510263909542 ) ) ;
#4811=ORIENTED_EDGE ( 'NONE', *, *, #17073, .T. ) ;
#4812=DIRECTION ( 'NONE',  ( -0.7071067811865501263, -0.7071067811865449082, 9.966407208441821704E-16 ) ) ;
#4815=ORIENTED_EDGE ( 'NONE', *, *, #14440, .F. ) ;
#4816=DIRECTION ( 'NONE',  ( 1.000000000000000000, 2.698458740408365879E-16, -1.110223024625156540E-16 ) ) ;
#4819=ORIENTED_EDGE ( 'NONE', *, *, #18035, .T. ) ;
#4823=VERTEX_POINT ( 'NONE', #10164 ) ;
#4824=VECTOR ( 'NONE', #10131, 1000.000000000000000 ) ;
#4827=VECTOR ( 'NONE', #6875, 1000.000000000000000 ) ;
#4829=ORIENTED_EDGE ( 'NONE', *, *, #15719, .F. ) ;
#4831=ORIENTED_EDGE ( 'NONE', *, *, #7603, .F. ) ;
#4833=CARTESIAN_POINT ( 'NONE',  ( 162.0152310637605240, -1.999999999999971800, -34.70218595412750773 ) ) ;
#4834=ORIENTED_EDGE ( 'NONE', *, *, #16936, .T. ) ;
#4835=CARTESIAN_POINT ( 'NONE',  ( 174.5152310637604671, -9.999999999999994671, -19.94844914048349693 ) ) ;
#4836=PLANE ( 'NONE',  #19991 ) ;
#4841=DIRECTION ( 'NONE',  ( -0.8090169943749474513, -2.183098979609982436E-16, -0.5877852522924731371 ) ) ;
#4842=CARTESIAN_POINT ( 'NONE',  ( 138.6922820468854525, -10.00000000000000533, -35.24709285013155835 ) ) ;
#4845=VECTOR ( 'NONE', #26869, 1000.000000000000000 ) ;
#4846=CARTESIAN_POINT ( 'NONE',  ( 163.6922820468853388, -9.999999999999998224, -17.92658477444275889 ) ) ;
#4847=ORIENTED_EDGE ( 'NONE', *, *, #2007, .F. ) ;
#4848=FACE_OUTER_BOUND ( 'NONE', #24730, .T. ) ;
#4851=ORIENTED_EDGE ( 'NONE', *, *, #5434, .T. ) ;
#4853=ORIENTED_EDGE ( 'NONE', *, *, #15755, .T. ) ;
#4856=CARTESIAN_POINT ( 'NONE',  ( 151.1922820468853956, -4.999999999999976907, -10.74328820663507678 ) ) ;
#4857=CARTESIAN_POINT ( 'NONE',  ( 177.2287565553228887, -9.999999999999994671, -20.83012701892220520 ) ) ;
#4859=PLANE ( 'NONE',  #9835 ) ;
#4860=AXIS2_PLACEMENT_3D ( 'NONE', #27661, #6428, #15717 ) ;
#4862=VECTOR ( 'NONE', #27059, 1000.000000000000000 ) ;
#4863=DIRECTION ( 'NONE',  ( 1.110223024625156540E-16, 2.995891024602366092E-32, 1.000000000000000000 ) ) ;
#4864=EDGE_CURVE ( 'NONE', #24083, #13474, #12757, .T. ) ;
#4865=DIRECTION ( 'NONE',  ( -0.9510565162951536422, -2.566386769018988323E-16, 0.3090169943749475623 ) ) ;
#4866=ADVANCED_FACE ( 'NONE', ( #21621 ), #7585, .T. ) ;
#4868=EDGE_CURVE ( 'NONE', #26851, #26883, #19477, .T. ) ;
#4870=CARTESIAN_POINT ( 'NONE',  ( 139.7287565553230309, -1.999999999999978684, -7.839745962155603820 ) ) ;
#4872=VECTOR ( 'NONE', #26962, 1000.000000000000000 ) ;
#4875=VERTEX_POINT ( 'NONE', #29140 ) ;
#4877=ORIENTED_EDGE ( 'NONE', *, *, #22315, .T. ) ;
#4878=CARTESIAN_POINT ( 'NONE',  ( 133.6922820468854241, -1.999999999999980904, -6.413161187712875133 ) ) ;
#4881=FACE_OUTER_BOUND ( 'NONE', #25539, .T. ) ;
#4882=ORIENTED_EDGE ( 'NONE', *, *, #25973, .T. ) ;
#4883=AXIS2_PLACEMENT_3D ( 'NONE', #3030, #14287, #2875 ) ;
#4886=DIRECTION ( 'NONE',  ( 1.000000000000000000, 2.698458740408365879E-16, -1.110223024625156540E-16 ) ) ;
#4887=VECTOR ( 'NONE', #13790, 1000.000000000000000 ) ;
#4889=DIRECTION ( 'NONE',  ( 0.5877852522924731371, 0.000000000000000000, 0.8090169943749474513 ) ) ;
#4891=ORIENTED_EDGE ( 'NONE', *, *, #2008, .F. ) ;
#4892=CARTESIAN_POINT ( 'NONE',  ( 172.0152310637604955, -9.999999999999994671, -34.70218595412750773 ) ) ;
#4893=ORIENTED_EDGE ( 'NONE', *, *, #13107, .F. ) ;
#4895=VERTEX_POINT ( 'NONE', #8177 ) ;
#4899=ORIENTED_EDGE ( 'NONE', *, *, #9409, .T. ) ;
#4907=DIRECTION ( 'NONE',  ( -0.5877852522924731371, -1.586114251531760235E-16, 0.8090169943749474513 ) ) ;
#4908=EDGE_CURVE ( 'NONE', #13418, #11002, #28848, .T. ) ;
#4909=EDGE_CURVE ( 'NONE', #27640, #17911, #17489, .T. ) ;
#4912=DIRECTION ( 'NONE',  ( 0.3090169943749475623, 8.338696094058001131E-17, 0.9510565162951536422 ) ) ;
#4913=CARTESIAN_POINT ( 'NONE',  ( 98.87704821043671188, -4.999999999999990230, -71.83838056851863030 ) ) ;
#4917=CARTESIAN_POINT ( 'NONE',  ( 154.7287565553229172, -10.00000000000000178, -16.50000000000000000 ) ) ;
#4919=ORIENTED_EDGE ( 'NONE', *, *, #13655, .T. ) ;
#4920=CARTESIAN_POINT ( 'NONE',  ( 180.7287565553229456, -3.999999999999989786, -33.50000000000000000 ) ) ;
#4922=AXIS2_PLACEMENT_3D ( 'NONE', #18520, #21110, #18818 ) ;
#4930=EDGE_LOOP ( 'NONE', ( #21403, #17413, #15713, #27252 ) ) ;
#4931=DIRECTION ( 'NONE',  ( -0.8090169943749474513, -2.183098979609982436E-16, -0.5877852522924731371 ) ) ;
#4933=VERTEX_POINT ( 'NONE', #10316 ) ;
#4936=PLANE ( 'NONE',  #13038 ) ;
#4938=VERTEX_POINT ( 'NONE', #24525 ) ;
#4939=DIRECTION ( 'NONE',  ( -0.5877852522924731371, -1.586114251531760235E-16, 0.8090169943749474513 ) ) ;
#4944=ORIENTED_EDGE ( 'NONE', *, *, #5929, .F. ) ;
#4946=DIRECTION ( 'NONE',  ( 0.3090169943749475623, 8.338696094058001131E-17, 0.9510565162951536422 ) ) ;
#4948=EDGE_CURVE ( 'NONE', #11956, #19044, #7886, .T. ) ;
#4950=EDGE_CURVE ( 'NONE', #1366, #22270, #24228, .T. ) ;
#4951=CARTESIAN_POINT ( 'NONE',  ( 136.1922820468854241, -4.999999999999980460, -4.936203717676158398 ) ) ;
#4952=ADVANCED_FACE ( 'NONE', ( #24078 ), #3179, .T. ) ;
#4953=LINE ( 'NONE', #18833, #25633 ) ;
#4954=CARTESIAN_POINT ( 'NONE',  ( 156.1922820468854241, -1.999999999999974021, -30.91696583120936026 ) ) ;
#4955=DIRECTION ( 'NONE',  ( 0.5877852522924731371, 0.000000000000000000, 0.8090169943749474513 ) ) ;
#4960=VERTEX_POINT ( 'NONE', #26522 ) ;
#4963=DIRECTION ( 'NONE',  ( -2.698458740408365879E-16, 1.000000000000000000, 0.000000000000000000 ) ) ;
#4964=DIRECTION ( 'NONE',  ( 0.5877852522924731371, 1.586114251531760728E-16, -0.8090169943749474513 ) ) ;
#4966=CARTESIAN_POINT ( 'NONE',  ( 139.5152310637605808, -10.00000000000000533, -2.627941064794695691 ) ) ;
#4968=ORIENTED_EDGE ( 'NONE', *, *, #28836, .T. ) ;
#4969=DIRECTION ( 'NONE',  ( -2.698458740408365879E-16, 1.000000000000000000, 0.000000000000000000 ) ) ;
#4970=CARTESIAN_POINT ( 'NONE',  ( 133.7287565553229456, -9.999999999999980460, 0.5000000000000029976 ) ) ;
#4972=ORIENTED_EDGE ( 'NONE', *, *, #11405, .T. ) ;
#4977=AXIS2_PLACEMENT_3D ( 'NONE', #26476, #3276, #10264 ) ;
#4981=VECTOR ( 'NONE', #16040, 1000.000000000000000 ) ;
#4982=ORIENTED_EDGE ( 'NONE', *, *, #4572, .T. ) ;
#4983=EDGE_CURVE ( 'NONE', #11457, #12771, #22385, .T. ) ;
#4984=DIRECTION ( 'NONE',  ( -0.9510565162951536422, 0.000000000000000000, -0.3090169943749472292 ) ) ;
#4985=EDGE_CURVE ( 'NONE', #13044, #8301, #27456, .T. ) ;
#4988=LINE ( 'NONE', #30088, #4098 ) ;
#4989=DIRECTION ( 'NONE',  ( 0.5877852522924731371, 0.000000000000000000, 0.8090169943749474513 ) ) ;
#4993=VECTOR ( 'NONE', #2599, 1000.000000000000000 ) ;
#4994=FACE_OUTER_BOUND ( 'NONE', #10305, .T. ) ;
#4995=DIRECTION ( 'NONE',  ( -0.5877852522924731371, -1.586114251531760728E-16, -0.8090169943749474513 ) ) ;
#4998=DIRECTION ( 'NONE',  ( 0.5877852522924731371, 1.586114251531760728E-16, 0.8090169943749474513 ) ) ;
#5000=ORIENTED_EDGE ( 'NONE', *, *, #24560, .T. ) ;
#5001=ORIENTED_EDGE ( 'NONE', *, *, #4358, .T. ) ;
#5002=DIRECTION ( 'NONE',  ( 1.110223024625156540E-16, 2.995891024602366092E-32, 1.000000000000000000 ) ) ;
#5003=VERTEX_POINT ( 'NONE', #20529 ) ;
#5004=DIRECTION ( 'NONE',  ( -0.9510565162951536422, -2.566386769018988323E-16, 0.3090169943749475623 ) ) ;
#5005=VECTOR ( 'NONE', #25618, 1000.000000000000000 ) ;
#5006=ORIENTED_EDGE ( 'NONE', *, *, #4699, .T. ) ;
#5007=DIRECTION ( 'NONE',  ( 1.908098474094866580E-16, -0.7071067811865481278, -0.7071067811865469066 ) ) ;
#5010=EDGE_CURVE ( 'NONE', #14, #22156, #29616, .T. ) ;
#5013=CARTESIAN_POINT ( 'NONE',  ( 168.6922820468852819, -9.999999999999998224, 2.247092850131519715 ) ) ;
#5015=LINE ( 'NONE', #14304, #5005 ) ;
#5017=CARTESIAN_POINT ( 'NONE',  ( 180.7287565553229740, -84.33034373659253902, 0.5000000000000029976 ) ) ;
#5019=CARTESIAN_POINT ( 'NONE',  ( 153.6922820468854241, -1.999999999999974909, -26.58683881228715862 ) ) ;
#5021=VECTOR ( 'NONE', #23927, 1000.000000000000000 ) ;
#5023=LINE ( 'NONE', #5904, #20399 ) ;
#5025=VERTEX_POINT ( 'NONE', #11076 ) ;
#5032=ORIENTED_EDGE ( 'NONE', *, *, #11212, .F. ) ;
#5033=VECTOR ( 'NONE', #18274, 1000.000000000000000 ) ;
#5036=LINE ( 'NONE', #12345, #8685 ) ;
#5038=CARTESIAN_POINT ( 'NONE',  ( 147.0152310637605524, -10.00000000000000178, -6.958068083716895558 ) ) ;
#5039=ORIENTED_EDGE ( 'NONE', *, *, #2717, .T. ) ;
#5040=DIRECTION ( 'NONE',  ( -0.8090169943749474513, -2.183098979609982436E-16, -0.5877852522924731371 ) ) ;
#5041=ORIENTED_EDGE ( 'NONE', *, *, #20481, .T. ) ;
#5043=EDGE_CURVE ( 'NONE', #26475, #5593, #6207, .T. ) ;
#5048=ORIENTED_EDGE ( 'NONE', *, *, #26142, .T. ) ;
#5049=EDGE_CURVE ( 'NONE', #22761, #29150, #8483, .T. ) ;
#5050=DIRECTION ( 'NONE',  ( 0.5877852522924731371, 0.000000000000000000, 0.8090169943749474513 ) ) ;
#5051=AXIS2_PLACEMENT_3D ( 'NONE', #27093, #15602, #10265 ) ;
#5057=ORIENTED_EDGE ( 'NONE', *, *, #30196, .T. ) ;
#5058=FACE_BOUND ( 'NONE', #21629, .T. ) ;
#5059=CARTESIAN_POINT ( 'NONE',  ( 151.1922820468854241, -1.999999999999976685, -19.40354224447947828 ) ) ;
#5060=LINE ( 'NONE', #19691, #29688 ) ;
#5062=CARTESIAN_POINT ( 'NONE',  ( 157.0152310637604671, -1.999999999999974465, -8.721423840594312082 ) ) ;
#5064=VECTOR ( 'NONE', #2457, 1000.000000000000000 ) ;
#5068=CARTESIAN_POINT ( 'NONE',  ( 156.1922820468853388, -4.999999999999976019, -2.083034168790677043 ) ) ;
#5069=ORIENTED_EDGE ( 'NONE', *, *, #29993, .T. ) ;
#5071=ORIENTED_EDGE ( 'NONE', *, *, #17582, .F. ) ;
#5074=DIRECTION ( 'NONE',  ( 0.9510565162951536422, 2.566386769018988816E-16, 0.3090169943749472292 ) ) ;
#5077=ORIENTED_EDGE ( 'NONE', *, *, #27482, .F. ) ;
#5078=DIRECTION ( 'NONE',  ( 0.3090169943749472292, 8.338696094057992503E-17, -0.9510565162951536422 ) ) ;
#5080=ADVANCED_FACE ( 'NONE', ( #29767 ), #17784, .T. ) ;
#5081=EDGE_LOOP ( 'NONE', ( #2441, #27057, #21294, #23293 ) ) ;
#5086=EDGE_CURVE ( 'NONE', #5568, #27071, #29464, .T. ) ;
#5087=CARTESIAN_POINT ( 'NONE',  ( 148.6922820468853672, -1.999999999999977573, -0.6060766987539614181 ) ) ;
#5089=EDGE_CURVE ( 'NONE', #4291, #20426, #24830, .T. ) ;
#5091=ORIENTED_EDGE ( 'NONE', *, *, #27098, .T. ) ;
#5092=CYLINDRICAL_SURFACE ( 'NONE', #15418, 3.000000000000002665 ) ;
#5095=VECTOR ( 'NONE', #23427, 1000.000000000000000 ) ;
#5098=ORIENTED_EDGE ( 'NONE', *, *, #20511, .T. ) ;
#5100=FACE_OUTER_BOUND ( 'NONE', #29736, .T. ) ;
#5102=DIRECTION ( 'NONE',  ( 0.5877852522924731371, 1.586114251531760728E-16, 0.8090169943749474513 ) ) ;
#5108=ORIENTED_EDGE ( 'NONE', *, *, #28150, .T. ) ;
#5109=CARTESIAN_POINT ( 'NONE',  ( 174.5152310637604955, -9.999999999999994671, -28.60870317832789667 ) ) ;
#5112=CARTESIAN_POINT ( 'NONE',  ( 22.20786350129493059, -5.000000000000011546, -68.34877589377062179 ) ) ;
#5113=DIRECTION ( 'NONE',  ( 0.9510565162951536422, 2.566386769018988816E-16, 0.3090169943749472292 ) ) ;
#5115=DIRECTION ( 'NONE',  ( 0.5877852522924731371, 1.586114251531760728E-16, -0.8090169943749474513 ) ) ;
#5118=CARTESIAN_POINT ( 'NONE',  ( 157.0152310637605524, -9.999999999999998224, -24.27857615940569502 ) ) ;
#5127=VECTOR ( 'NONE', #19327, 1000.000000000000000 ) ;
#5129=VERTEX_POINT ( 'NONE', #27144 ) ;
#5132=ORIENTED_EDGE ( 'NONE', *, *, #16484, .F. ) ;
#5133=VECTOR ( 'NONE', #27522, 999.9999999999998863 ) ;
#5134=EDGE_LOOP ( 'NONE', ( #28756, #26610, #7566, #11979 ) ) ;
#5135=DIRECTION ( 'NONE',  ( 0.3090169943749472292, 8.338696094057992503E-17, -0.9510565162951536422 ) ) ;
#5136=LINE ( 'NONE', #4833, #23865 ) ;
#5138=LINE ( 'NONE', #12443, #2190 ) ;
#5139=FACE_OUTER_BOUND ( 'NONE', #11007, .T. ) ;
#5143=ORIENTED_EDGE ( 'NONE', *, *, #5010, .T. ) ;
#5145=LINE ( 'NONE', #425, #34 ) ;
#5146=LINE ( 'NONE', #7291, #28098 ) ;
#5149=DIRECTION ( 'NONE',  ( -2.698458740408365879E-16, 1.000000000000000000, 0.000000000000000000 ) ) ;
#5150=VERTEX_POINT ( 'NONE', #29301 ) ;
#5151=VECTOR ( 'NONE', #13987, 1000.000000000000000 ) ;
#5152=LINE ( 'NONE', #14890, #19280 ) ;
#5153=ORIENTED_EDGE ( 'NONE', *, *, #7399, .F. ) ;
#5155=EDGE_CURVE ( 'NONE', #6477, #10414, #17639, .T. ) ;
#5156=CARTESIAN_POINT ( 'NONE',  ( 176.1922820468852819, -9.999999999999994671, -10.74328820663507678 ) ) ;
#5158=EDGE_CURVE ( 'NONE', #8151, #28202, #1640, .T. ) ;
#5159=DIRECTION ( 'NONE',  ( -0.9510565162951536422, -2.566386769018988816E-16, -0.3090169943749472292 ) ) ;
#5160=EDGE_LOOP ( 'NONE', ( #8266, #9035, #468, #28301 ) ) ;
#5161=ADVANCED_FACE ( 'NONE', ( #17932 ), #27307, .T. ) ;
#5166=LINE ( 'NONE', #14457, #12598 ) ;
#5167=DIRECTION ( 'NONE',  ( -0.5877852522924731371, 0.000000000000000000, 0.8090169943749474513 ) ) ;
#5168=VECTOR ( 'NONE', #30067, 1000.000000000000000 ) ;
#5170=LINE ( 'NONE', #21495, #10354 ) ;
#5171=CARTESIAN_POINT ( 'NONE',  ( 141.1922820468854525, -4.999999999999979572, -10.74328820663507678 ) ) ;
#5173=DIRECTION ( 'NONE',  ( 0.5877852522924731371, 1.586114251531760728E-16, 0.8090169943749474513 ) ) ;
#5175=CARTESIAN_POINT ( 'NONE',  ( 172.2287565553228887, -9.999999999999996447, -12.16987298107780369 ) ) ;
#5177=CARTESIAN_POINT ( 'NONE',  ( 147.2287565553230024, -10.00000000000000355, -12.16987298107780369 ) ) ;
#5179=ORIENTED_EDGE ( 'NONE', *, *, #8988, .T. ) ;
#5184=CARTESIAN_POINT ( 'NONE',  ( 133.7287565553229172, -1.999999999999980904, -39.49999999999997158 ) ) ;
#5188=AXIS2_PLACEMENT_3D ( 'NONE', #11973, #21292, #19599 ) ;
#5190=CARTESIAN_POINT ( 'NONE',  ( 136.1922820468854241, -1.999999999999980460, -22.25671179336495697 ) ) ;
#5191=VERTEX_POINT ( 'NONE', #1788 ) ;
#5194=ORIENTED_EDGE ( 'NONE', *, *, #27653, .T. ) ;
#5195=ADVANCED_FACE ( 'NONE', ( #23436 ), #13950, .T. ) ;
#5197=ORIENTED_EDGE ( 'NONE', *, *, #21304, .T. ) ;
#5198=VECTOR ( 'NONE', #17273, 1000.000000000000000 ) ;
#5203=ORIENTED_EDGE ( 'NONE', *, *, #9761, .F. ) ;
#5206=ORIENTED_EDGE ( 'NONE', *, *, #29448, .T. ) ;
#5210=DIRECTION ( 'NONE',  ( 1.110223024625156540E-16, 2.995891024602366092E-32, 1.000000000000000000 ) ) ;
#5211=DIRECTION ( 'NONE',  ( 0.9510565162951535312, 2.566386769018988816E-16, -0.3090169943749475623 ) ) ;
#5212=EDGE_CURVE ( 'NONE', #22963, #28478, #28206, .T. ) ;
#5213=DIRECTION ( 'NONE',  ( -0.5877852522924731371, 0.000000000000000000, 0.8090169943749474513 ) ) ;
#5214=LINE ( 'NONE', #12227, #16942 ) ;
#5215=DIRECTION ( 'NONE',  ( -1.110223024625156540E-16, 0.000000000000000000, -1.000000000000000000 ) ) ;
#5216=VECTOR ( 'NONE', #15582, 999.9999999999998863 ) ;
#5218=VECTOR ( 'NONE', #19848, 999.9999999999998863 ) ;
#5220=CARTESIAN_POINT ( 'NONE',  ( 166.1922820468853388, -1.999999999999972244, -13.59645775552055902 ) ) ;
#5221=CARTESIAN_POINT ( 'NONE',  ( 129.5152310637605808, -1.999999999999982236, -19.94844914048349338 ) ) ;
#5222=ORIENTED_EDGE ( 'NONE', *, *, #28393, .T. ) ;
#5224=ORIENTED_EDGE ( 'NONE', *, *, #11440, .F. ) ;
#5226=PLANE ( 'NONE',  #22450 ) ;
#5227=DIRECTION ( 'NONE',  ( 1.000000000000000000, 0.000000000000000000, -0.000000000000000000 ) ) ;
#5228=CARTESIAN_POINT ( 'NONE',  ( 168.6922820468853672, -1.999999999999971356, -32.39392330124607611 ) ) ;
#5229=ORIENTED_EDGE ( 'NONE', *, *, #13147, .F. ) ;
#5230=CARTESIAN_POINT ( 'NONE',  ( 141.1922820468854525, -1.999999999999978684, -30.91696583120935671 ) ) ;
#5235=ORIENTED_EDGE ( 'NONE', *, *, #4983, .T. ) ;
#5236=VECTOR ( 'NONE', #15579, 999.9999999999998863 ) ;
#5237=DIRECTION ( 'NONE',  ( -0.5877852522924731371, 0.000000000000000000, 0.8090169943749474513 ) ) ;
#5240=EDGE_LOOP ( 'NONE', ( #26853, #27752, #16114, #5838 ) ) ;
#5241=FACE_OUTER_BOUND ( 'NONE', #19291, .T. ) ;
#5243=VECTOR ( 'NONE', #11939, 1000.000000000000000 ) ;
#5245=ORIENTED_EDGE ( 'NONE', *, *, #31, .F. ) ;
#5246=CARTESIAN_POINT ( 'NONE',  ( 129.5152310637605808, -1.999999999999982236, -28.60870317832789311 ) ) ;
#5249=CARTESIAN_POINT ( 'NONE',  ( 129.5152310637605808, -10.00000000000000888, -19.94844914048349338 ) ) ;
#5251=FACE_OUTER_BOUND ( 'NONE', #13545, .T. ) ;
#5252=ADVANCED_FACE ( 'NONE', ( #16101 ), #25424, .T. ) ;
#5253=ADVANCED_FACE ( 'NONE', ( #7260 ), #90, .T. ) ;
#5254=CARTESIAN_POINT ( 'NONE',  ( 169.7287565553230024, -4.999999999999971578, -33.82050807568879947 ) ) ;
#5256=EDGE_CURVE ( 'NONE', #7473, #26028, #7416, .T. ) ;
#5257=DIRECTION ( 'NONE',  ( -1.000000000000000000, -2.698458740408365879E-16, 1.779203565104417375E-16 ) ) ;
#5258=AXIS2_PLACEMENT_3D ( 'NONE', #27198, #22887, #6251 ) ;
#5259=EDGE_CURVE ( 'NONE', #22420, #7083, #9373, .T. ) ;
#5265=DIRECTION ( 'NONE',  ( 1.000000000000000000, 2.698458740408366372E-16, 0.000000000000000000 ) ) ;
#5266=VECTOR ( 'NONE', #22020, 1000.000000000000000 ) ;
#5268=CARTESIAN_POINT ( 'NONE',  ( 158.6922820468853956, -9.999999999999998224, -23.73366926340167637 ) ) ;
#5269=CARTESIAN_POINT ( 'NONE',  ( 172.0152310637604955, -4.999999999999971578, -24.27857615940569502 ) ) ;
#5270=CARTESIAN_POINT ( 'NONE',  ( 154.5152310637605240, -1.999999999999974909, -11.28819510263909542 ) ) ;
#5273=LINE ( 'NONE', #28511, #13445 ) ;
#5275=PLANE ( 'NONE',  #5188 ) ;
#5276=LINE ( 'NONE', #14863, #17595 ) ;
#5287=EDGE_LOOP ( 'NONE', ( #25747, #27176, #5955, #9495 ) ) ;
#5288=PLANE ( 'NONE',  #13769 ) ;
#5289=VECTOR ( 'NONE', #9423, 1000.000000000000000 ) ;
#5290=EDGE_CURVE ( 'NONE', #24650, #30115, #11510, .T. ) ;
#5291=VECTOR ( 'NONE', #28598, 1000.000000000000000 ) ;
#5292=CARTESIAN_POINT ( 'NONE',  ( 139.7287565553230309, -4.999999999999980460, -33.82050807568879947 ) ) ;
#5293=ORIENTED_EDGE ( 'NONE', *, *, #26892, .T. ) ;
#5294=EDGE_CURVE ( 'NONE', #27047, #24269, #9679, .T. ) ;
#5295=EDGE_CURVE ( 'NONE', #2569, #1403, #13802, .T. ) ;
#5296=LINE ( 'NONE', #7882, #225 ) ;
#5297=EDGE_CURVE ( 'NONE', #28729, #17627, #18546, .T. ) ;
#5298=CARTESIAN_POINT ( 'NONE',  ( 174.7287565553228887, -9.999999999999994671, -16.50000000000000355 ) ) ;
#5302=CARTESIAN_POINT ( 'NONE',  ( 134.5152310637605808, -1.999999999999980460, -11.28819510263909187 ) ) ;
#5304=PLANE ( 'NONE',  #4883 ) ;
#5306=ORIENTED_EDGE ( 'NONE', *, *, #13528, .F. ) ;
#5307=VECTOR ( 'NONE', #22043, 1000.000000000000000 ) ;
#5308=DIRECTION ( 'NONE',  ( 1.110223024625156540E-16, 2.995891024602366092E-32, 1.000000000000000000 ) ) ;
#5309=DIRECTION ( 'NONE',  ( -2.698458740408365879E-16, 1.000000000000000000, 0.000000000000000000 ) ) ;
#5310=ORIENTED_EDGE ( 'NONE', *, *, #17546, .T. ) ;
#5312=AXIS2_PLACEMENT_3D ( 'NONE', #9738, #19056, #28412 ) ;
#5313=ORIENTED_EDGE ( 'NONE', *, *, #20289, .F. ) ;
#5318=PLANE ( 'NONE',  #29735 ) ;
#5320=EDGE_CURVE ( 'NONE', #15263, #11825, #11819, .T. ) ;
#5321=ORIENTED_EDGE ( 'NONE', *, *, #21642, .T. ) ;
#5322=LINE ( 'NONE', #14612, #23547 ) ;
#5323=CARTESIAN_POINT ( 'NONE',  ( 108.6946756682487774, -4.999999999999987566, -78.97130444073225419 ) ) ;
#5324=AXIS2_PLACEMENT_3D ( 'NONE', #26751, #19841, #13127 ) ;
#5326=ORIENTED_EDGE ( 'NONE', *, *, #8582, .F. ) ;
#5327=EDGE_CURVE ( 'NONE', #5386, #4109, #21284, .T. ) ;
#5330=DIRECTION ( 'NONE',  ( 1.110223024625156540E-16, 2.995891024602366092E-32, 1.000000000000000000 ) ) ;
#5331=EDGE_CURVE ( 'NONE', #5737, #28689, #6961, .T. ) ;
#5332=VECTOR ( 'NONE', #16739, 1000.000000000000000 ) ;
#5333=EDGE_CURVE ( 'NONE', #4933, #13070, #18701, .T. ) ;
#5335=FACE_OUTER_BOUND ( 'NONE', #20108, .T. ) ;
#5337=EDGE_LOOP ( 'NONE', ( #17433, #15477, #14331, #20210 ) ) ;
#5342=DIRECTION ( 'NONE',  ( 8.163404592832029035E-16, 2.202861047501738386E-31, 1.000000000000000000 ) ) ;
#5343=VERTEX_POINT ( 'NONE', #14102 ) ;
#5345=DIRECTION ( 'NONE',  ( -2.698458740408365879E-16, 1.000000000000000000, 0.000000000000000000 ) ) ;
#5347=CARTESIAN_POINT ( 'NONE',  ( 154.5152310637605524, -10.00000000000000000, -19.94844914048349693 ) ) ;
#5348=ORIENTED_EDGE ( 'NONE', *, *, #19315, .F. ) ;
#5349=CARTESIAN_POINT ( 'NONE',  ( 143.6922820468854241, -10.00000000000000355, -9.266330736598359152 ) ) ;
#5350=EDGE_LOOP ( 'NONE', ( #16424, #10741, #20017, #21684, #1618 ) ) ;
#5352=VERTEX_POINT ( 'NONE', #246 ) ;
#5353=VECTOR ( 'NONE', #28123, 1000.000000000000000 ) ;
#5357=ORIENTED_EDGE ( 'NONE', *, *, #5434, .F. ) ;
#5359=LINE ( 'NONE', #19381, #5749 ) ;
#5362=LINE ( 'NONE', #21533, #25442 ) ;
#5366=PLANE ( 'NONE',  #305 ) ;
#5367=FACE_BOUND ( 'NONE', #18828, .T. ) ;
#5368=EDGE_CURVE ( 'NONE', #280, #25774, #9522, .T. ) ;
#5370=EDGE_CURVE ( 'NONE', #1829, #18677, #11369, .T. ) ;
#5371=DIRECTION ( 'NONE',  ( -0.8090169943749474513, -2.183098979609982436E-16, 0.5877852522924731371 ) ) ;
#5372=CARTESIAN_POINT ( 'NONE',  ( 167.0152310637605240, -1.999999999999970468, -34.70218595412750773 ) ) ;
#5373=AXIS2_PLACEMENT_3D ( 'NONE', #16405, #13952, #92 ) ;
#5374=LINE ( 'NONE', #644, #17496 ) ;
#5376=VECTOR ( 'NONE', #10117, 1000.000000000000000 ) ;
#5378=LINE ( 'NONE', #5678, #26551 ) ;
#5379=CARTESIAN_POINT ( 'NONE',  ( 129.5152310637605524, -10.00000000000000888, -13.05155085951650840 ) ) ;
#5380=ORIENTED_EDGE ( 'NONE', *, *, #685, .T. ) ;
#5383=CARTESIAN_POINT ( 'NONE',  ( 149.5152310637605524, -10.00000000000000178, -21.71180489736091346 ) ) ;
#5384=CARTESIAN_POINT ( 'NONE',  ( 171.1922820468853672, -1.999999999999970024, -30.91696583120936026 ) ) ;
#5385=DIRECTION ( 'NONE',  ( 0.3090169943749472292, 8.338696094057992503E-17, -0.9510565162951536422 ) ) ;
#5386=VERTEX_POINT ( 'NONE', #9069 ) ;
#5387=DIRECTION ( 'NONE',  ( -0.8090169943749474513, -2.183098979609982436E-16, -0.5877852522924731371 ) ) ;
#5389=ORIENTED_EDGE ( 'NONE', *, *, #5929, .T. ) ;
#5391=VECTOR ( 'NONE', #17269, 1000.000000000000000 ) ;
#5396=ORIENTED_EDGE ( 'NONE', *, *, #17148, .T. ) ;
#5398=EDGE_CURVE ( 'NONE', #18781, #22599, #28816, .T. ) ;
#5399=AXIS2_PLACEMENT_3D ( 'NONE', #22865, #4244, #24709 ) ;
#5402=CARTESIAN_POINT ( 'NONE',  ( 166.1922820468853388, -9.999999999999998224, -10.74328820663507678 ) ) ;
#5403=ORIENTED_EDGE ( 'NONE', *, *, #9926, .T. ) ;
#5405=CARTESIAN_POINT ( 'NONE',  ( 169.5152310637604103, -9.999999999999996447, -4.391296821672111328 ) ) ;
#5406=ORIENTED_EDGE ( 'NONE', *, *, #2234, .F. ) ;
#5409=CARTESIAN_POINT ( 'NONE',  ( 138.6922820468854525, -1.999999999999979572, -35.24709285013155835 ) ) ;
#5410=LINE ( 'NONE', #21726, #24307 ) ;
#5412=CARTESIAN_POINT ( 'NONE',  ( 104.9993066664142702, -4.999999999999988454, -76.28646170422676676 ) ) ;
#5417=ORIENTED_EDGE ( 'NONE', *, *, #17404, .F. ) ;
#5419=CARTESIAN_POINT ( 'NONE',  ( 133.6922820468854241, -10.00000000000000711, -32.39392330124607611 ) ) ;
#5420=CARTESIAN_POINT ( 'NONE',  ( 147.0152310637604955, -4.999999999999977796, -0.06116980274991495881 ) ) ;
#5421=DIRECTION ( 'NONE',  ( 0.9510565162951536422, 0.000000000000000000, -0.3090169943749475623 ) ) ;
#5423=DIRECTION ( 'NONE',  ( 0.9510565162951535312, 2.566386769018988816E-16, -0.3090169943749475623 ) ) ;
#5425=CARTESIAN_POINT ( 'NONE',  ( 146.1922820468853956, -10.00000000000000355, -4.936203717676158398 ) ) ;
#5427=DIRECTION ( 'NONE',  ( 0.9510565162951536422, 2.566386769018988816E-16, 0.3090169943749472292 ) ) ;
#5428=CARTESIAN_POINT ( 'NONE',  ( 147.2287565553230024, -4.999999999999977796, -12.16987298107780013 ) ) ;
#5431=ORIENTED_EDGE ( 'NONE', *, *, #9761, .T. ) ;
#5433=VECTOR ( 'NONE', #10011, 1000.000000000000000 ) ;
#5434=EDGE_CURVE ( 'NONE', #12418, #13408, #28507, .T. ) ;
#5435=CARTESIAN_POINT ( 'NONE',  ( 0.000000000000000000, 0.000000000000000000, 0.000000000000000000 ) ) ;
#5437=VECTOR ( 'NONE', #6781, 1000.000000000000000 ) ;
#5438=EDGE_CURVE ( 'NONE', #8637, #3882, #14708, .T. ) ;
#5440=ORIENTED_EDGE ( 'NONE', *, *, #12648, .F. ) ;
#5441=ORIENTED_EDGE ( 'NONE', *, *, #2251, .T. ) ;
#5443=CARTESIAN_POINT ( 'NONE',  ( 167.0152310637604955, -4.999999999999972466, -15.61832212156129707 ) ) ;
#5444=EDGE_LOOP ( 'NONE', ( #22931, #25946, #40, #17730 ) ) ;
#5446=ORIENTED_EDGE ( 'NONE', *, *, #26971, .F. ) ;
#5448=DIRECTION ( 'NONE',  ( -2.698458740408365879E-16, 1.000000000000000000, 0.000000000000000000 ) ) ;
#5449=PLANE ( 'NONE',  #1973 ) ;
#5453=DIRECTION ( 'NONE',  ( 0.5877852522924731371, 1.586114251531760728E-16, -0.8090169943749474513 ) ) ;
#5456=CARTESIAN_POINT ( 'NONE',  ( 157.0152310637604955, -10.00000000000000000, -17.38167787843871182 ) ) ;
#5457=ORIENTED_EDGE ( 'NONE', *, *, #5545, .F. ) ;
#5459=DIRECTION ( 'NONE',  ( 0.9510565162951535312, 2.566386769018988816E-16, -0.3090169943749475623 ) ) ;
#5460=VERTEX_POINT ( 'NONE', #3434 ) ;
#5461=LINE ( 'NONE', #3626, #21476 ) ;
#5462=ORIENTED_EDGE ( 'NONE', *, *, #4535, .T. ) ;
#5463=ORIENTED_EDGE ( 'NONE', *, *, #11516, .T. ) ;
#5468=EDGE_CURVE ( 'NONE', #10339, #21691, #22048, .T. ) ;
#5470=DIRECTION ( 'NONE',  ( -2.698458740408365879E-16, 1.000000000000000000, 0.000000000000000000 ) ) ;
#5471=DIRECTION ( 'NONE',  ( -0.5877852522924731371, -1.586114251531760235E-16, 0.8090169943749474513 ) ) ;
#5472=VECTOR ( 'NONE', #26276, 1000.000000000000000 ) ;
#5474=CARTESIAN_POINT ( 'NONE',  ( 144.7287565553229740, -4.999999999999978684, 0.8205080756888000204 ) ) ;
#5475=DIRECTION ( 'NONE',  ( -0.8090169943749474513, -2.183098979609982436E-16, 0.5877852522924731371 ) ) ;
#5476=DIRECTION ( 'NONE',  ( 0.5877852522924731371, 1.586114251531760728E-16, 0.8090169943749474513 ) ) ;
#5477=DIRECTION ( 'NONE',  ( 0.3090169943749475623, 8.338696094058001131E-17, 0.9510565162951536422 ) ) ;
#5479=FACE_OUTER_BOUND ( 'NONE', #28221, .T. ) ;
#5483=ORIENTED_EDGE ( 'NONE', *, *, #10564, .T. ) ;
#5485=VECTOR ( 'NONE', #8648, 1000.000000000000000 ) ;
#5488=FACE_BOUND ( 'NONE', #11156, .T. ) ;
#5489=EDGE_CURVE ( 'NONE', #22161, #24130, #28872, .T. ) ;
#5492=LINE ( 'NONE', #14775, #20387 ) ;
#5494=DIRECTION ( 'NONE',  ( -2.698458740408365879E-16, 1.000000000000000000, 0.000000000000000000 ) ) ;
#5496=CARTESIAN_POINT ( 'NONE',  ( 164.7287565553228887, -9.999999999999998224, -7.839745962155603820 ) ) ;
#5497=ORIENTED_EDGE ( 'NONE', *, *, #25324, .F. ) ;
#5499=VERTEX_POINT ( 'NONE', #1150 ) ;
#5504=VECTOR ( 'NONE', #24251, 1000.000000000000000 ) ;
#5505=EDGE_CURVE ( 'NONE', #12263, #18517, #843, .T. ) ;
#5506=CARTESIAN_POINT ( 'NONE',  ( 7.497985849899103883, -5.000000000000015987, 23.07642761220746053 ) ) ;
#5507=VERTEX_POINT ( 'NONE', #26645 ) ;
#5508=EDGE_CURVE ( 'NONE', #16977, #7341, #12572, .T. ) ;
#5509=ORIENTED_EDGE ( 'NONE', *, *, #4362, .F. ) ;
#5510=EDGE_CURVE ( 'NONE', #20748, #22102, #17455, .T. ) ;
#5511=EDGE_CURVE ( 'NONE', #7152, #24650, #23744, .T. ) ;
#5512=CARTESIAN_POINT ( 'NONE',  ( 157.0152310637605240, -1.999999999999973577, -26.04193191628311155 ) ) ;
#5517=VECTOR ( 'NONE', #20251, 1000.000000000000000 ) ;
#5518=CARTESIAN_POINT ( 'NONE',  ( 158.6922820468853672, -1.999999999999974021, -17.92658477444275889 ) ) ;
#5519=FACE_BOUND ( 'NONE', #29648, .T. ) ;
#5520=PLANE ( 'NONE',  #8187 ) ;
#5521=CARTESIAN_POINT ( 'NONE',  ( 167.0152310637604955, -9.999999999999996447, -26.04193191628311155 ) ) ;
#5523=CARTESIAN_POINT ( 'NONE',  ( 169.5152310637604103, -4.999999999999971578, -4.391296821672111328 ) ) ;
#5525=CARTESIAN_POINT ( 'NONE',  ( 138.6922820468854525, -1.999999999999979572, -23.73366926340167282 ) ) ;
#5526=DIRECTION ( 'NONE',  ( 0.3090169943749475623, 8.338696094058001131E-17, 0.9510565162951536422 ) ) ;
#5527=VERTEX_POINT ( 'NONE', #12127 ) ;
#5530=VECTOR ( 'NONE', #12749, 1000.000000000000000 ) ;
#5533=LINE ( 'NONE', #5384, #12043 ) ;
#5534=DIRECTION ( 'NONE',  ( 0.9510565162951536422, 2.566386769018988816E-16, 0.3090169943749472292 ) ) ;
#5535=ORIENTED_EDGE ( 'NONE', *, *, #3478, .F. ) ;
#5536=VERTEX_POINT ( 'NONE', #5269 ) ;
#5543=ORIENTED_EDGE ( 'NONE', *, *, #17232, .T. ) ;
#5544=ORIENTED_EDGE ( 'NONE', *, *, #18205, .F. ) ;
#5545=EDGE_CURVE ( 'NONE', #17674, #7452, #19593, .T. ) ;
#5546=ORIENTED_EDGE ( 'NONE', *, *, #24561, .T. ) ;
#5547=LINE ( 'NONE', #12699, #3810 ) ;
#5553=ORIENTED_EDGE ( 'NONE', *, *, #19314, .T. ) ;
#5556=EDGE_LOOP ( 'NONE', ( #3191, #25186, #25550, #16516 ) ) ;
#5557=CARTESIAN_POINT ( 'NONE',  ( 100.8158076689448990, -4.999999999999990230, 73.24697176669747023 ) ) ;
#5559=PLANE ( 'NONE',  #20139 ) ;
#5560=CARTESIAN_POINT ( 'NONE',  ( 177.2287565553228603, -9.999999999999994671, -12.16987298107780369 ) ) ;
#5561=DIRECTION ( 'NONE',  ( -2.698458740408365879E-16, 1.000000000000000000, 0.000000000000000000 ) ) ;
#5566=ADVANCED_FACE ( 'NONE', ( #7706 ), #12277, .T. ) ;
#5568=VERTEX_POINT ( 'NONE', #19446 ) ;
#5569=DIRECTION ( 'NONE',  ( -2.698458740408365879E-16, 1.000000000000000000, 0.000000000000000000 ) ) ;
#5573=CARTESIAN_POINT ( 'NONE',  ( 172.7287565553229456, -1.999999999999970468, -39.49999999999997868 ) ) ;
#5574=DIRECTION ( 'NONE',  ( 0.9510565162951535312, 2.566386769018988816E-16, -0.3090169943749475623 ) ) ;
#5580=DIRECTION ( 'NONE',  ( 0.3090169943749475623, 8.338696094058001131E-17, 0.9510565162951536422 ) ) ;
#5584=ORIENTED_EDGE ( 'NONE', *, *, #20407, .F. ) ;
#5585=ADVANCED_FACE ( 'NONE', ( #25087 ), #24637, .T. ) ;
#5593=VERTEX_POINT ( 'NONE', #11186 ) ;
#5594=CARTESIAN_POINT ( 'NONE',  ( 156.1922820468853388, -1.999999999999975353, -4.936203717676158398 ) ) ;
#5596=DIRECTION ( 'NONE',  ( -0.9510565162951536422, 0.000000000000000000, -0.3090169943749472292 ) ) ;
#5598=CARTESIAN_POINT ( 'NONE',  ( 176.1922820468853388, -1.999999999999968914, -30.91696583120936026 ) ) ;
#5599=EDGE_CURVE ( 'NONE', #28522, #13253, #11039, .T. ) ;
#5600=EDGE_CURVE ( 'NONE', #28929, #16735, #15156, .T. ) ;
#5603=EDGE_CURVE ( 'NONE', #9294, #12464, #6322, .T. ) ;
#5608=CARTESIAN_POINT ( 'NONE',  ( 139.5152310637605808, -4.999999999999980460, -30.37205893520530964 ) ) ;
#5609=PLANE ( 'NONE',  #19830 ) ;
#5610=ORIENTED_EDGE ( 'NONE', *, *, #23733, .F. ) ;
#5611=LINE ( 'NONE', #17053, #9020 ) ;
#5612=LINE ( 'NONE', #17498, #11729 ) ;
#5613=CARTESIAN_POINT ( 'NONE',  ( 172.0152310637605240, -9.999999999999994671, -32.93883019725009120 ) ) ;
#5616=VERTEX_POINT ( 'NONE', #20341 ) ;
#5621=DIRECTION ( 'NONE',  ( 1.000000000000000000, 2.698458740408365879E-16, -1.110223024625156540E-16 ) ) ;
#5622=CARTESIAN_POINT ( 'NONE',  ( 147.0152310637605808, -4.999999999999977796, -1.632196944975745421E-14 ) ) ;
#5623=VECTOR ( 'NONE', #7029, 1000.000000000000000 ) ;
#5624=DIRECTION ( 'NONE',  ( 1.000000000000000000, 2.698458740408367851E-16, 0.000000000000000000 ) ) ;
#5625=VERTEX_POINT ( 'NONE', #29881 ) ;
#5626=LINE ( 'NONE', #17218, #18154 ) ;
#5627=ORIENTED_EDGE ( 'NONE', *, *, #131, .F. ) ;
#5629=DIRECTION ( 'NONE',  ( -0.9510565162951536422, 0.000000000000000000, -0.3090169943749472292 ) ) ;
#5630=ORIENTED_EDGE ( 'NONE', *, *, #25616, .T. ) ;
#5631=CARTESIAN_POINT ( 'NONE',  ( 138.6922820468854525, -10.00000000000000533, -15.07341522555727309 ) ) ;
#5632=DIRECTION ( 'NONE',  ( -0.5877852522924731371, -1.586114251531760728E-16, -0.8090169943749474513 ) ) ;
#5635=EDGE_CURVE ( 'NONE', #29774, #16222, #22650, .T. ) ;
#5636=ORIENTED_EDGE ( 'NONE', *, *, #11075, .T. ) ;
#5640=ADVANCED_FACE ( 'NONE', ( #13030 ), #8446, .T. ) ;
#5641=VECTOR ( 'NONE', #27305, 1000.000000000000000 ) ;
#5642=ADVANCED_FACE ( 'NONE', ( #15304 ), #18203, .T. ) ;
#5645=FACE_BOUND ( 'NONE', #6825, .T. ) ;
#5646=ORIENTED_EDGE ( 'NONE', *, *, #30084, .T. ) ;
#5648=DIRECTION ( 'NONE',  ( -0.5877852522924731371, -1.586114251531760728E-16, -0.8090169943749474513 ) ) ;
#5651=ORIENTED_EDGE ( 'NONE', *, *, #12787, .F. ) ;
#5652=FACE_OUTER_BOUND ( 'NONE', #9794, .T. ) ;
#5655=VECTOR ( 'NONE', #14438, 1000.000000000000000 ) ;
#5659=VECTOR ( 'NONE', #22086, 1000.000000000000000 ) ;
#5660=DIRECTION ( 'NONE',  ( 0.5877852522924731371, 1.586114251531760728E-16, 0.8090169943749474513 ) ) ;
#5667=DIRECTION ( 'NONE',  ( 1.000000000000000000, 2.698458740408365879E-16, -1.110223024625156540E-16 ) ) ;
#5668=FACE_BOUND ( 'NONE', #14783, .T. ) ;
#5670=EDGE_CURVE ( 'NONE', #4933, #28698, #19894, .T. ) ;
#5671=CARTESIAN_POINT ( 'NONE',  ( 159.5152310637605524, -9.999999999999998224, -28.60870317832789667 ) ) ;
#5673=ADVANCED_FACE ( 'NONE', ( #10744 ), #13471, .T. ) ;
#5675=VECTOR ( 'NONE', #24995, 1000.000000000000000 ) ;
#5676=EDGE_CURVE ( 'NONE', #14294, #15364, #22801, .T. ) ;
#5678=CARTESIAN_POINT ( 'NONE',  ( 169.5152310637604103, -1.999999999999971356, -4.391296821672111328 ) ) ;
#5679=ORIENTED_EDGE ( 'NONE', *, *, #26474, .F. ) ;
#5681=VERTEX_POINT ( 'NONE', #24491 ) ;
#5682=AXIS2_PLACEMENT_3D ( 'NONE', #24761, #3849, #27534 ) ;
#5686=CARTESIAN_POINT ( 'NONE',  ( 163.6922820468852819, -4.999999999999973355, 2.247092850131519715 ) ) ;
#5687=DIRECTION ( 'NONE',  ( 1.000000000000000000, 2.698458740408365879E-16, -1.110223024625156540E-16 ) ) ;
#5688=CARTESIAN_POINT ( 'NONE',  ( 169.5152310637604955, -9.999999999999996447, -19.94844914048349693 ) ) ;
#5689=VERTEX_POINT ( 'NONE', #17751 ) ;
#5690=CARTESIAN_POINT ( 'NONE',  ( 146.1922820468854525, -4.999999999999977796, -28.06379628232387446 ) ) ;
#5691=EDGE_LOOP ( 'NONE', ( #25456, #20125, #14195, #24805, #29229, #4475, #29846, #20602, #11377, #17139, #25592, #13367, #27041, #366, #14238, #12342, #22997, #1733, #21799, #20684, #7129, #10058, #8788, #7596, #22296, #19648, #9789, #18188, #22749, #5704, #955, #1348, #16477, #18743, #3400, #16144, #30212, #3947, #13630, #17564, #14278, #2418, #24597, #17325 ) ) ;
#5695=ORIENTED_EDGE ( 'NONE', *, *, #14261, .T. ) ;
#5696=DIRECTION ( 'NONE',  ( 0.5877852522924731371, 0.000000000000000000, 0.8090169943749474513 ) ) ;
#5698=CARTESIAN_POINT ( 'NONE',  ( 131.1922820468854241, -10.00000000000000888, -19.40354224447947473 ) ) ;
#5699=FACE_OUTER_BOUND ( 'NONE', #6897, .T. ) ;
#5702=VECTOR ( 'NONE', #3707, 1000.000000000000000 ) ;
#5703=ORIENTED_EDGE ( 'NONE', *, *, #19196, .F. ) ;
#5704=ORIENTED_EDGE ( 'NONE', *, *, #1661, .F. ) ;
#5707=ORIENTED_EDGE ( 'NONE', *, *, #9572, .T. ) ;
#5708=AXIS2_PLACEMENT_3D ( 'NONE', #27635, #6700, #2133 ) ;
#5709=LINE ( 'NONE', #3420, #655 ) ;
#5710=LINE ( 'NONE', #21582, #830 ) ;
#5711=VECTOR ( 'NONE', #20482, 1000.000000000000000 ) ;
#5715=DIRECTION ( 'NONE',  ( 0.9510565162951536422, 0.000000000000000000, -0.3090169943749475623 ) ) ;
#5718=EDGE_CURVE ( 'NONE', #22368, #4371, #4032, .T. ) ;
#5721=DIRECTION ( 'NONE',  ( -2.698458740408365879E-16, 1.000000000000000000, 0.000000000000000000 ) ) ;
#5723=DIRECTION ( 'NONE',  ( -2.698458740408365879E-16, 1.000000000000000000, 0.000000000000000000 ) ) ;
#5724=DIRECTION ( 'NONE',  ( -2.698458740408365879E-16, 1.000000000000000000, 0.000000000000000000 ) ) ;
#5725=VECTOR ( 'NONE', #14670, 1000.000000000000000 ) ;
#5726=DIRECTION ( 'NONE',  ( 0.9510565162951535312, 2.566386769018988816E-16, -0.3090169943749475623 ) ) ;
#5728=VERTEX_POINT ( 'NONE', #23397 ) ;
#5729=CARTESIAN_POINT ( 'NONE',  ( 172.0152310637604103, -1.999999999999970912, 1.702185954127501066 ) ) ;
#5731=AXIS2_PLACEMENT_3D ( 'NONE', #4787, #12249, #5237 ) ;
#5732=CARTESIAN_POINT ( 'NONE',  ( 175.7287565553229456, -9.999999999999971578, 3.500000000000003109 ) ) ;
#5733=LINE ( 'NONE', #29115, #25409 ) ;
#5737=VERTEX_POINT ( 'NONE', #6616 ) ;
#5738=LINE ( 'NONE', #28975, #9575 ) ;
#5742=EDGE_CURVE ( 'NONE', #26944, #29723, #6925, .T. ) ;
#5744=VECTOR ( 'NONE', #26266, 1000.000000000000000 ) ;
#5745=CARTESIAN_POINT ( 'NONE',  ( 133.7287565553229456, -4.000000000000003553, 8.500000000000007105 ) ) ;
#5746=ORIENTED_EDGE ( 'NONE', *, *, #20653, .F. ) ;
#5747=ORIENTED_EDGE ( 'NONE', *, *, #13351, .T. ) ;
#5749=VECTOR ( 'NONE', #3228, 999.9999999999998863 ) ;
#5750=CARTESIAN_POINT ( 'NONE',  ( 3.839988787535719261, -5.000000000000016875, 11.81827027433623734 ) ) ;
#5751=DIRECTION ( 'NONE',  ( 0.5877852522924731371, 1.586114251531760728E-16, -0.8090169943749474513 ) ) ;
#5758=CARTESIAN_POINT ( 'NONE',  ( 144.5152310637605808, -1.999999999999977573, -11.28819510263909542 ) ) ;
#5760=LINE ( 'NONE', #8030, #12677 ) ;
#5761=CARTESIAN_POINT ( 'NONE',  ( 172.0152310637603819, -9.999999999999996447, -0.06116980274991495881 ) ) ;
#5762=ORIENTED_EDGE ( 'NONE', *, *, #19383, .F. ) ;
#5763=LINE ( 'NONE', #1190, #25645 ) ;
#5765=VECTOR ( 'NONE', #15786, 1000.000000000000000 ) ;
#5766=FACE_OUTER_BOUND ( 'NONE', #4493, .T. ) ;
#5767=ORIENTED_EDGE ( 'NONE', *, *, #25832, .T. ) ;
#5768=ORIENTED_EDGE ( 'NONE', *, *, #25320, .F. ) ;
#5769=EDGE_LOOP ( 'NONE', ( #24998, #8551, #27947, #23201 ) ) ;
#5774=PLANE ( 'NONE',  #4798 ) ;
#5777=EDGE_CURVE ( 'NONE', #25730, #17843, #21102, .T. ) ;
#5778=ORIENTED_EDGE ( 'NONE', *, *, #16959, .T. ) ;
#5779=LINE ( 'NONE', #19348, #14724 ) ;
#5780=DIRECTION ( 'NONE',  ( 0.3090169943749472292, 8.338696094057992503E-17, -0.9510565162951536422 ) ) ;
#5781=ORIENTED_EDGE ( 'NONE', *, *, #28760, .T. ) ;
#5782=CARTESIAN_POINT ( 'NONE',  ( 162.0152310637604671, -9.999999999999998224, -6.958068083716895558 ) ) ;
#5784=EDGE_CURVE ( 'NONE', #18885, #26241, #15909, .T. ) ;
#5787=VECTOR ( 'NONE', #28803, 1000.000000000000000 ) ;
#5788=EDGE_LOOP ( 'NONE', ( #5194, #14429, #11267, #8827 ) ) ;
#5792=FACE_BOUND ( 'NONE', #24163, .T. ) ;
#5795=ORIENTED_EDGE ( 'NONE', *, *, #18303, .T. ) ;
#5799=EDGE_LOOP ( 'NONE', ( #13620, #22872, #14489, #22037 ) ) ;
#5801=VERTEX_POINT ( 'NONE', #20943 ) ;
#5803=EDGE_LOOP ( 'NONE', ( #17200, #22567, #7220, #29454, #6630 ) ) ;
#5806=VERTEX_POINT ( 'NONE', #28168 ) ;
#5807=DIRECTION ( 'NONE',  ( -1.110223024625156540E-16, 0.000000000000000000, -1.000000000000000000 ) ) ;
#5811=EDGE_CURVE ( 'NONE', #13972, #18723, #27712, .T. ) ;
#5812=EDGE_CURVE ( 'NONE', #25860, #102, #9487, .T. ) ;
#5813=EDGE_CURVE ( 'NONE', #25448, #20344, #13771, .T. ) ;
#5814=VECTOR ( 'NONE', #19882, 1000.000000000000000 ) ;
#5815=EDGE_CURVE ( 'NONE', #21366, #8557, #11474, .T. ) ;
#5817=CARTESIAN_POINT ( 'NONE',  ( 149.5152310637605524, -4.999999999999976907, -1.659952520591374019E-14 ) ) ;
#5818=DIRECTION ( 'NONE',  ( -0.9510565162951536422, 0.000000000000000000, -0.3090169943749472292 ) ) ;
#5819=CARTESIAN_POINT ( 'NONE',  ( 157.2287565553230024, -10.00000000000000000, -29.49038105676660493 ) ) ;
#5821=CARTESIAN_POINT ( 'NONE',  ( 8.452900878024367515, -5.000000000000015099, 26.01535387366982732 ) ) ;
#5822=DIRECTION ( 'NONE',  ( -2.698458740408365879E-16, 1.000000000000000000, 0.000000000000000000 ) ) ;
#5825=ORIENTED_EDGE ( 'NONE', *, *, #26743, .T. ) ;
#5826=AXIS2_PLACEMENT_3D ( 'NONE', #3984, #9135, #1865 ) ;
#5827=LINE ( 'NONE', #17119, #4245 ) ;
#5830=ORIENTED_EDGE ( 'NONE', *, *, #11572, .T. ) ;
#5833=PLANE ( 'NONE',  #17397 ) ;
#5834=ORIENTED_EDGE ( 'NONE', *, *, #8754, .F. ) ;
#5835=AXIS2_PLACEMENT_3D ( 'NONE', #28711, #5477, #12635 ) ;
#5836=ORIENTED_EDGE ( 'NONE', *, *, #520, .F. ) ;
#5837=DIRECTION ( 'NONE',  ( -0.5877852522924731371, 0.000000000000000000, 0.8090169943749474513 ) ) ;
#5838=ORIENTED_EDGE ( 'NONE', *, *, #8004, .F. ) ;
#5840=VERTEX_POINT ( 'NONE', #4624 ) ;
#5852=EDGE_CURVE ( 'NONE', #17919, #2926, #4325, .T. ) ;
#5854=VERTEX_POINT ( 'NONE', #2359 ) ;
#5855=LINE ( 'NONE', #5557, #21047 ) ;
#5856=AXIS2_PLACEMENT_3D ( 'NONE', #14008, #23492, #18911 ) ;
#5857=AXIS2_PLACEMENT_3D ( 'NONE', #21397, #20937, #25527 ) ;
#5858=LINE ( 'NONE', #11018, #7276 ) ;
#5859=VECTOR ( 'NONE', #6537, 1000.000000000000000 ) ;
#5860=CARTESIAN_POINT ( 'NONE',  ( 133.7287565553229456, -9.999999999999980460, 8.500000000000003553 ) ) ;
#5861=AXIS2_PLACEMENT_3D ( 'NONE', #6196, #17920, #22828 ) ;
#5862=LINE ( 'NONE', #15144, #16421 ) ;
#5863=DIRECTION ( 'NONE',  ( -0.9510565162951536422, 0.000000000000000000, -0.3090169943749472292 ) ) ;
#5864=LINE ( 'NONE', #4019, #16301 ) ;
#5869=VECTOR ( 'NONE', #14448, 1000.000000000000000 ) ;
#5872=DIRECTION ( 'NONE',  ( 0.5877852522924731371, 0.000000000000000000, 0.8090169943749474513 ) ) ;
#5873=CARTESIAN_POINT ( 'NONE',  ( 133.6922820468854241, -10.00000000000000711, -15.07341522555727309 ) ) ;
#5876=DIRECTION ( 'NONE',  ( 0.9510565162951536422, 0.000000000000000000, -0.3090169943749475623 ) ) ;
#5877=FACE_OUTER_BOUND ( 'NONE', #11328, .T. ) ;
#5879=ORIENTED_EDGE ( 'NONE', *, *, #6746, .T. ) ;
#5880=PLANE ( 'NONE',  #4674 ) ;
#5882=EDGE_CURVE ( 'NONE', #23347, #888, #18667, .T. ) ;
#5884=CARTESIAN_POINT ( 'NONE',  ( 139.7287565553230309, -4.999999999999979572, -25.16025403784439973 ) ) ;
#5885=DIRECTION ( 'NONE',  ( -2.698458740408365879E-16, 1.000000000000000000, 0.000000000000000000 ) ) ;
#5888=DIRECTION ( 'NONE',  ( 0.5877852522924731371, 1.586114251531760728E-16, -0.8090169943749474513 ) ) ;
#5890=ORIENTED_EDGE ( 'NONE', *, *, #17332, .T. ) ;
#5891=DIRECTION ( 'NONE',  ( -0.5877852522924731371, -1.586114251531760728E-16, -0.8090169943749474513 ) ) ;
#5894=EDGE_CURVE ( 'NONE', #7473, #26271, #13623, .T. ) ;
#5896=EDGE_CURVE ( 'NONE', #18587, #13963, #9646, .T. ) ;
#5897=EDGE_CURVE ( 'NONE', #9309, #16652, #2514, .T. ) ;
#5898=LINE ( 'NONE', #1170, #12713 ) ;
#5901=LINE ( 'NONE', #29130, #12656 ) ;
#5904=CARTESIAN_POINT ( 'NONE',  ( 167.2287565553229456, -9.999999999999998224, -20.83012701892220520 ) ) ;
#5906=DIRECTION ( 'NONE',  ( -2.698458740408365879E-16, 1.000000000000000000, 0.000000000000000000 ) ) ;
#5910=PLANE ( 'NONE',  #13225 ) ;
#5913=DIRECTION ( 'NONE',  ( 0.5877852522924731371, 1.586114251531760728E-16, -0.8090169943749474513 ) ) ;
#5914=CARTESIAN_POINT ( 'NONE',  ( 138.6922820468854241, -1.999999999999980016, -0.6060766987539614181 ) ) ;
#5915=VECTOR ( 'NONE', #9559, 1000.000000000000000 ) ;
#5916=ORIENTED_EDGE ( 'NONE', *, *, #2413, .T. ) ;
#5918=LINE ( 'NONE', #27153, #5659 ) ;
#5920=DIRECTION ( 'NONE',  ( -0.5877852522924731371, 0.000000000000000000, 0.8090169943749474513 ) ) ;
#5921=ORIENTED_EDGE ( 'NONE', *, *, #9051, .F. ) ;
#5925=ADVANCED_FACE ( 'NONE', ( #21249 ), #27563, .T. ) ;
#5927=LINE ( 'NONE', #15212, #2860 ) ;
#5928=FACE_OUTER_BOUND ( 'NONE', #4329, .T. ) ;
#5929=EDGE_CURVE ( 'NONE', #6861, #23077, #26599, .T. ) ;
#5930=CARTESIAN_POINT ( 'NONE',  ( 142.0152310637606092, -10.00000000000000355, -32.93883019725009120 ) ) ;
#5932=ORIENTED_EDGE ( 'NONE', *, *, #17141, .F. ) ;
#5933=CARTESIAN_POINT ( 'NONE',  ( 173.6922820468852819, -1.999999999999970024, -6.413161187712876909 ) ) ;
#5934=LINE ( 'NONE', #24099, #25336 ) ;
#5935=EDGE_LOOP ( 'NONE', ( #25680, #9529, #20094, #11677 ) ) ;
#5936=DIRECTION ( 'NONE',  ( 0.3090169943749472292, 8.338696094057992503E-17, -0.9510565162951536422 ) ) ;
#5937=CARTESIAN_POINT ( 'NONE',  ( 152.2287565553229456, -4.999999999999976907, -3.509618943233400401 ) ) ;
#5942=VERTEX_POINT ( 'NONE', #28321 ) ;
#5945=FACE_BOUND ( 'NONE', #13298, .T. ) ;
#5946=ADVANCED_FACE ( 'NONE', ( #7516 ), #19557, .T. ) ;
#5947=ORIENTED_EDGE ( 'NONE', *, *, #10800, .T. ) ;
#5949=VERTEX_POINT ( 'NONE', #12532 ) ;
#5951=AXIS2_PLACEMENT_3D ( 'NONE', #29827, #8837, #4567 ) ;
#5952=DIRECTION ( 'NONE',  ( 0.9510565162951536422, 2.566386769018988816E-16, 0.3090169943749472292 ) ) ;
#5954=PLANE ( 'NONE',  #25201 ) ;
#5955=ORIENTED_EDGE ( 'NONE', *, *, #17783, .F. ) ;
#5957=EDGE_LOOP ( 'NONE', ( #3542, #4853, #18816, #22389, #19255 ) ) ;
#5960=DIRECTION ( 'NONE',  ( -2.698458740408365879E-16, 1.000000000000000000, 0.000000000000000000 ) ) ;
#5961=ORIENTED_EDGE ( 'NONE', *, *, #24957, .T. ) ;
#5962=LINE ( 'NONE', #935, #3530 ) ;
#5964=VECTOR ( 'NONE', #21578, 1000.000000000000000 ) ;
#5966=PLANE ( 'NONE',  #1594 ) ;
#5967=VECTOR ( 'NONE', #29486, 1000.000000000000000 ) ;
#5968=ORIENTED_EDGE ( 'NONE', *, *, #10161, .F. ) ;
#5969=LINE ( 'NONE', #10383, #19014 ) ;
#5971=DIRECTION ( 'NONE',  ( 0.9510565162951536422, 2.566386769018988816E-16, 0.3090169943749472292 ) ) ;
#5972=CARTESIAN_POINT ( 'NONE',  ( 139.7287565553230309, -4.999999999999980460, -7.839745962155600267 ) ) ;
#5974=EDGE_CURVE ( 'NONE', #18890, #20837, #960, .T. ) ;
#5975=PLANE ( 'NONE',  #13494 ) ;
#5976=ORIENTED_EDGE ( 'NONE', *, *, #1242, .F. ) ;
#5977=CARTESIAN_POINT ( 'NONE',  ( 157.0152310637604955, -4.999999999999975131, -6.958068083716895558 ) ) ;
#5978=ORIENTED_EDGE ( 'NONE', *, *, #19578, .F. ) ;
#5981=DIRECTION ( 'NONE',  ( -0.5877852522924731371, 0.000000000000000000, 0.8090169943749474513 ) ) ;
#5984=EDGE_LOOP ( 'NONE', ( #28943, #21665, #1195, #13828, #12735 ) ) ;
#5986=ORIENTED_EDGE ( 'NONE', *, *, #8660, .T. ) ;
#5990=ORIENTED_EDGE ( 'NONE', *, *, #21425, .T. ) ;
#5991=CARTESIAN_POINT ( 'NONE',  ( 159.7287565553229740, -1.999999999999972689, -25.16025403784440329 ) ) ;
#5995=CARTESIAN_POINT ( 'NONE',  ( 103.8408967599626749, -4.999999999999989342, -75.44482764232697036 ) ) ;
#5998=ORIENTED_EDGE ( 'NONE', *, *, #3032, .T. ) ;
#6001=FACE_OUTER_BOUND ( 'NONE', #22884, .T. ) ;
#6002=VECTOR ( 'NONE', #5476, 1000.000000000000000 ) ;
#6004=DIRECTION ( 'NONE',  ( 0.9510565162951535312, 2.566386769018988816E-16, -0.3090169943749475623 ) ) ;
#6005=DIRECTION ( 'NONE',  ( -2.698458740408365879E-16, 1.000000000000000000, 0.000000000000000000 ) ) ;
#6006=FACE_OUTER_BOUND ( 'NONE', #1713, .T. ) ;
#6007=CARTESIAN_POINT ( 'NONE',  ( 163.6922820468853104, -4.999999999999973355, -9.266330736598359152 ) ) ;
#6008=VECTOR ( 'NONE', #1208, 1000.000000000000000 ) ;
#6012=ADVANCED_FACE ( 'NONE', ( #24015 ), #5226, .T. ) ;
#6013=EDGE_CURVE ( 'NONE', #24548, #9707, #16675, .T. ) ;
#6014=VERTEX_POINT ( 'NONE', #5686 ) ;
#6016=DIRECTION ( 'NONE',  ( 1.000000000000000000, 2.698458740408365879E-16, -1.110223024625156540E-16 ) ) ;
#6018=LINE ( 'NONE', #8297, #22448 ) ;
#6021=DIRECTION ( 'NONE',  ( -0.9510565162951536422, -2.566386769018988816E-16, -0.3090169943749472292 ) ) ;
#6025=ORIENTED_EDGE ( 'NONE', *, *, #6948, .F. ) ;
#6026=LINE ( 'NONE', #22352, #10017 ) ;
#6029=CARTESIAN_POINT ( 'NONE',  ( 147.0152310637605524, -1.999999999999977129, -6.958068083716895558 ) ) ;
#6031=CARTESIAN_POINT ( 'NONE',  ( 130.7287565553229456, -4.999999999999983125, 3.500000000000003109 ) ) ;
#6033=ORIENTED_EDGE ( 'NONE', *, *, #28282, .F. ) ;
#6034=CARTESIAN_POINT ( 'NONE',  ( 113.9712810924319797, -4.999999999999986677, -82.80498268490511293 ) ) ;
#6035=EDGE_LOOP ( 'NONE', ( #19667, #11495, #14664, #1767, #10738 ) ) ;
#6039=VECTOR ( 'NONE', #4014, 1000.000000000000000 ) ;
#6040=ORIENTED_EDGE ( 'NONE', *, *, #27075, .T. ) ;
#6043=FACE_OUTER_BOUND ( 'NONE', #15318, .T. ) ;
#6044=CARTESIAN_POINT ( 'NONE',  ( 127.7287565553229740, -1.999999999999982681, 0.5000000000000397460 ) ) ;
#6045=DIRECTION ( 'NONE',  ( -2.698458740408365879E-16, 1.000000000000000000, 0.000000000000000000 ) ) ;
#6050=DIRECTION ( 'NONE',  ( -2.698458740408365879E-16, 1.000000000000000000, 0.000000000000000000 ) ) ;
#6053=VECTOR ( 'NONE', #26711, 1000.000000000000000 ) ;
#6056=EDGE_CURVE ( 'NONE', #6774, #12566, #19405, .T. ) ;
#6057=EDGE_CURVE ( 'NONE', #18517, #21669, #21405, .T. ) ;
#6059=FACE_OUTER_BOUND ( 'NONE', #14935, .T. ) ;
#6060=CARTESIAN_POINT ( 'NONE',  ( 172.2287565553229172, -1.999999999999969580, -20.83012701892220520 ) ) ;
#6062=VERTEX_POINT ( 'NONE', #802 ) ;
#6063=PLANE ( 'NONE',  #10995 ) ;
#6064=CARTESIAN_POINT ( 'NONE',  ( 134.7287565553230024, -10.00000000000000711, -33.82050807568879947 ) ) ;
#6065=CARTESIAN_POINT ( 'NONE',  ( 164.5152310637604387, -4.999999999999973355, -4.391296821672111328 ) ) ;
#6066=ORIENTED_EDGE ( 'NONE', *, *, #29403, .T. ) ;
#6072=CARTESIAN_POINT ( 'NONE',  ( 163.6922820468852819, -1.999999999999973133, 2.247092850131519715 ) ) ;
#6073=FACE_OUTER_BOUND ( 'NONE', #24845, .T. ) ;
#6074=FACE_OUTER_BOUND ( 'NONE', #13336, .T. ) ;
#6075=VECTOR ( 'NONE', #17923, 1000.000000000000000 ) ;
#6077=ORIENTED_EDGE ( 'NONE', *, *, #2755, .F. ) ;
#6078=DIRECTION ( 'NONE',  ( -0.5877852522924731371, 0.000000000000000000, 0.8090169943749474513 ) ) ;
#6079=DIRECTION ( 'NONE',  ( -2.698458740408365879E-16, 1.000000000000000000, 0.000000000000000000 ) ) ;
#6086=EDGE_CURVE ( 'NONE', #29734, #26271, #21697, .T. ) ;
#6087=EDGE_CURVE ( 'NONE', #23116, #17842, #509, .T. ) ;
#6091=FACE_BOUND ( 'NONE', #15265, .T. ) ;
#6092=ADVANCED_FACE ( 'NONE', ( #28610 ), #7667, .T. ) ;
#6093=ORIENTED_EDGE ( 'NONE', *, *, #7697, .T. ) ;
#6094=CARTESIAN_POINT ( 'NONE',  ( 172.2287565553228603, -1.999999999999970468, -3.509618943233403510 ) ) ;
#6095=VECTOR ( 'NONE', #14244, 1000.000000000000000 ) ;
#6097=CARTESIAN_POINT ( 'NONE',  ( 132.0152310637605808, -10.00000000000000711, -24.27857615940569147 ) ) ;
#6098=ORIENTED_EDGE ( 'NONE', *, *, #9758, .F. ) ;
#6099=LINE ( 'NONE', #8528, #29641 ) ;
#6100=ORIENTED_EDGE ( 'NONE', *, *, #3033, .T. ) ;
#6105=FACE_OUTER_BOUND ( 'NONE', #5799, .T. ) ;
#6106=EDGE_LOOP ( 'NONE', ( #8573, #12990, #11398, #46 ) ) ;
#6110=ORIENTED_EDGE ( 'NONE', *, *, #17913, .T. ) ;
#6112=FACE_BOUND ( 'NONE', #4092, .T. ) ;
#6113=VECTOR ( 'NONE', #23197, 999.9999999999998863 ) ;
#6115=LINE ( 'NONE', #24746, #21089 ) ;
#6117=CARTESIAN_POINT ( 'NONE',  ( 151.1922820468854241, -4.999999999999976907, -22.25671179336496053 ) ) ;
#6119=ORIENTED_EDGE ( 'NONE', *, *, #20622, .F. ) ;
#6120=DIRECTION ( 'NONE',  ( -0.8090169943749474513, -2.183098979609982436E-16, 0.5877852522924731371 ) ) ;
#6123=EDGE_CURVE ( 'NONE', #10558, #22420, #10242, .T. ) ;
#6125=LINE ( 'NONE', #128, #24662 ) ;
#6127=DIRECTION ( 'NONE',  ( -0.8090169943749474513, -2.183098979609982436E-16, -0.5877852522924731371 ) ) ;
#6128=ORIENTED_EDGE ( 'NONE', *, *, #21680, .F. ) ;
#6129=VECTOR ( 'NONE', #1375, 999.9999999999998863 ) ;
#6131=PLANE ( 'NONE',  #19539 ) ;
#6132=PLANE ( 'NONE',  #17425 ) ;
#6133=DIRECTION ( 'NONE',  ( -0.5877852522924731371, -1.586114251531760235E-16, 0.8090169943749474513 ) ) ;
#6136=ORIENTED_EDGE ( 'NONE', *, *, #18264, .F. ) ;
#6140=VERTEX_POINT ( 'NONE', #17566 ) ;
#6141=ORIENTED_EDGE ( 'NONE', *, *, #10477, .T. ) ;
#6143=CARTESIAN_POINT ( 'NONE',  ( 134.5152310637605808, -4.999999999999981348, -2.627941064794695691 ) ) ;
#6144=CARTESIAN_POINT ( 'NONE',  ( 134.7287565553230024, -10.00000000000000711, -16.50000000000000000 ) ) ;
#6145=CARTESIAN_POINT ( 'NONE',  ( 131.1922820468854241, -4.999999999999982236, -10.74328820663507322 ) ) ;
#6147=AXIS2_PLACEMENT_3D ( 'NONE', #16087, #4503, #28639 ) ;
#6149=ORIENTED_EDGE ( 'NONE', *, *, #2491, .T. ) ;
#6150=ORIENTED_EDGE ( 'NONE', *, *, #21754, .T. ) ;
#6151=EDGE_CURVE ( 'NONE', #3855, #25397, #10396, .T. ) ;
#6155=AXIS2_PLACEMENT_3D ( 'NONE', #21450, #25892, #16864 ) ;
#6156=DIRECTION ( 'NONE',  ( -2.698458740408365879E-16, 1.000000000000000000, 0.000000000000000000 ) ) ;
#6157=LINE ( 'NONE', #24781, #29670 ) ;
#6158=CARTESIAN_POINT ( 'NONE',  ( 157.0152310637604387, -10.00000000000000000, -0.06116980274991495881 ) ) ;
#6160=LINE ( 'NONE', #8287, #11433 ) ;
#6161=VECTOR ( 'NONE', #23741, 1000.000000000000000 ) ;
#6165=VERTEX_POINT ( 'NONE', #29219 ) ;
#6167=DIRECTION ( 'NONE',  ( -0.5877852522924731371, 0.000000000000000000, 0.8090169943749474513 ) ) ;
#6168=ORIENTED_EDGE ( 'NONE', *, *, #3675, .T. ) ;
#6171=CARTESIAN_POINT ( 'NONE',  ( 139.5152310637606092, -4.999999999999979572, -28.60870317832789311 ) ) ;
#6174=DIRECTION ( 'NONE',  ( 1.110223024625156540E-16, 2.995891024602366092E-32, 1.000000000000000000 ) ) ;
#6176=DIRECTION ( 'NONE',  ( -2.698458740408365879E-16, 1.000000000000000000, 0.000000000000000000 ) ) ;
#6177=CARTESIAN_POINT ( 'NONE',  ( 142.0152310637606092, -10.00000000000000355, -24.27857615940569147 ) ) ;
#6180=LINE ( 'NONE', #15168, #22295 ) ;
#6182=EDGE_LOOP ( 'NONE', ( #27277, #9247, #2340, #21506, #17026 ) ) ;
#6184=ORIENTED_EDGE ( 'NONE', *, *, #13385, .T. ) ;
#6188=VECTOR ( 'NONE', #4620, 1000.000000000000000 ) ;
#6189=ORIENTED_EDGE ( 'NONE', *, *, #14859, .T. ) ;
#6190=ADVANCED_FACE ( 'NONE', ( #20014 ), #29692, .T. ) ;
#6193=ADVANCED_FACE ( 'NONE', ( #27073 ), #15270, .T. ) ;
#6195=CARTESIAN_POINT ( 'NONE',  ( 158.6922820468853388, -10.00000000000000000, -9.266330736598359152 ) ) ;
#6196=CARTESIAN_POINT ( 'NONE',  ( 159.5152310637604955, -9.999999999999998224, -11.28819510263909542 ) ) ;
#6197=CARTESIAN_POINT ( 'NONE',  ( 171.1922820468853388, -1.999999999999970468, -22.25671179336496053 ) ) ;
#6198=FACE_OUTER_BOUND ( 'NONE', #8677, .T. ) ;
#6199=AXIS2_PLACEMENT_3D ( 'NONE', #18966, #7226, #5227 ) ;
#6207=LINE ( 'NONE', #25124, #18077 ) ;
#6208=FACE_OUTER_BOUND ( 'NONE', #16911, .T. ) ;
#6212=CARTESIAN_POINT ( 'NONE',  ( 18.23030615683139644, -5.000000000000012434, -56.10711313654469024 ) ) ;
#6216=DIRECTION ( 'NONE',  ( 0.9510565162951536422, 2.566386769018988816E-16, 0.3090169943749472292 ) ) ;
#6217=DIRECTION ( 'NONE',  ( -0.9510565162951536422, -2.566386769018988816E-16, -0.3090169943749472292 ) ) ;
#6218=ORIENTED_EDGE ( 'NONE', *, *, #6821, .T. ) ;
#6224=DIRECTION ( 'NONE',  ( -0.5877852522924731371, -1.586114251531760728E-16, -0.8090169943749474513 ) ) ;
#6225=CARTESIAN_POINT ( 'NONE',  ( 167.2287565553229740, -9.999999999999996447, -29.49038105676660493 ) ) ;
#6226=LINE ( 'NONE', #22564, #17185 ) ;
#6228=ADVANCED_FACE ( 'NONE', ( #8256 ), #1412, .T. ) ;
#6229=EDGE_CURVE ( 'NONE', #29408, #10756, #1711, .T. ) ;
#6230=ADVANCED_FACE ( 'NONE', ( #3692 ), #6131, .T. ) ;
#6231=ORIENTED_EDGE ( 'NONE', *, *, #30222, .F. ) ;
#6233=CARTESIAN_POINT ( 'NONE',  ( 129.5152310637605808, -10.00000000000000888, -28.60870317832789311 ) ) ;
#6234=VECTOR ( 'NONE', #18342, 1000.000000000000000 ) ;
#6237=DIRECTION ( 'NONE',  ( -0.5877852522924731371, 0.000000000000000000, 0.8090169943749474513 ) ) ;
#6240=ORIENTED_EDGE ( 'NONE', *, *, #25702, .T. ) ;
#6242=ORIENTED_EDGE ( 'NONE', *, *, #21166, .T. ) ;
#6243=AXIS2_PLACEMENT_3D ( 'NONE', #13325, #29575, #2322 ) ;
#6246=CARTESIAN_POINT ( 'NONE',  ( 149.5152310637604955, -10.00000000000000178, -4.391296821672111328 ) ) ;
#6247=ORIENTED_EDGE ( 'NONE', *, *, #28616, .T. ) ;
#6249=CARTESIAN_POINT ( 'NONE',  ( 142.2287565553230024, -10.00000000000000533, -3.509618943233403510 ) ) ;
#6251=DIRECTION ( 'NONE',  ( 0.9510565162951536422, 0.000000000000000000, -0.3090169943749475623 ) ) ;
#6252=EDGE_LOOP ( 'NONE', ( #16969, #7148, #15001, #14025 ) ) ;
#6254=EDGE_LOOP ( 'NONE', ( #18779, #18525, #7670, #21521, #10674, #3039 ) ) ;
#6259=CARTESIAN_POINT ( 'NONE',  ( 154.5152310637604671, -10.00000000000000178, -4.391296821672111328 ) ) ;
#6260=ORIENTED_EDGE ( 'NONE', *, *, #24740, .T. ) ;
#6261=DIRECTION ( 'NONE',  ( 0.9510565162951535312, 2.566386769018988816E-16, -0.3090169943749475623 ) ) ;
#6263=EDGE_CURVE ( 'NONE', #27224, #23986, #24760, .T. ) ;
#6264=VECTOR ( 'NONE', #3364, 1000.000000000000000 ) ;
#6265=EDGE_CURVE ( 'NONE', #4310, #16894, #27385, .T. ) ;
#6268=ADVANCED_FACE ( 'NONE', ( #25058 ), #27232, .T. ) ;
#6269=PLANE ( 'NONE',  #3087 ) ;
#6270=VECTOR ( 'NONE', #21492, 1000.000000000000000 ) ;
#6271=EDGE_LOOP ( 'NONE', ( #28727, #8049, #22630, #25535 ) ) ;
#6272=CARTESIAN_POINT ( 'NONE',  ( 157.0152310637605524, -4.999999999999975131, -24.27857615940569502 ) ) ;
#6274=LINE ( 'NONE', #13870, #29277 ) ;
#6279=ORIENTED_EDGE ( 'NONE', *, *, #9714, .F. ) ;
#6283=DIRECTION ( 'NONE',  ( 0.9510565162951535312, 2.566386769018988816E-16, -0.3090169943749475623 ) ) ;
#6284=EDGE_LOOP ( 'NONE', ( #27724, #3824, #23982, #27001 ) ) ;
#6285=DIRECTION ( 'NONE',  ( -2.698458740408365879E-16, 1.000000000000000000, 0.000000000000000000 ) ) ;
#6286=ORIENTED_EDGE ( 'NONE', *, *, #28912, .T. ) ;
#6288=VECTOR ( 'NONE', #22244, 1000.000000000000000 ) ;
#6291=ORIENTED_EDGE ( 'NONE', *, *, #22136, .T. ) ;
#6295=DIRECTION ( 'NONE',  ( -0.5877852522924731371, 0.000000000000000000, 0.8090169943749474513 ) ) ;
#6296=AXIS2_PLACEMENT_3D ( 'NONE', #20170, #19570, #26618 ) ;
#6299=EDGE_CURVE ( 'NONE', #10211, #14083, #22768, .T. ) ;
#6300=EDGE_CURVE ( 'NONE', #19520, #17576, #6895, .T. ) ;
#6301=EDGE_CURVE ( 'NONE', #14224, #7426, #18170, .T. ) ;
#6302=VERTEX_POINT ( 'NONE', #9453 ) ;
#6305=VECTOR ( 'NONE', #8594, 1000.000000000000000 ) ;
#6307=PLANE ( 'NONE',  #19178 ) ;
#6309=AXIS2_PLACEMENT_3D ( 'NONE', #6158, #12712, #29562 ) ;
#6310=CARTESIAN_POINT ( 'NONE',  ( 143.6922820468854525, -10.00000000000000355, -15.07341522555727664 ) ) ;
#6314=VECTOR ( 'NONE', #418, 1000.000000000000000 ) ;
#6317=CARTESIAN_POINT ( 'NONE',  ( 158.6922820468854241, -1.999999999999972689, -32.39392330124607611 ) ) ;
#6318=LINE ( 'NONE', #27414, #1317 ) ;
#6319=ORIENTED_EDGE ( 'NONE', *, *, #13892, .F. ) ;
#6322=LINE ( 'NONE', #13326, #25856 ) ;
#6323=CARTESIAN_POINT ( 'NONE',  ( 162.0152310637604955, -9.999999999999998224, -15.61832212156129707 ) ) ;
#6325=ORIENTED_EDGE ( 'NONE', *, *, #16896, .T. ) ;
#6326=ORIENTED_EDGE ( 'NONE', *, *, #11426, .F. ) ;
#6327=DIRECTION ( 'NONE',  ( 0.5877852522924731371, 1.586114251531760728E-16, -0.8090169943749474513 ) ) ;
#6333=CARTESIAN_POINT ( 'NONE',  ( 147.0152310637605808, -1.999999999999976241, -26.04193191628311155 ) ) ;
#6335=ORIENTED_EDGE ( 'NONE', *, *, #26532, .F. ) ;
#6336=CARTESIAN_POINT ( 'NONE',  ( 172.7287565553229456, -4.999999999999971578, 3.500000000000003109 ) ) ;
#6340=VECTOR ( 'NONE', #11029, 1000.000000000000000 ) ;
#6341=VECTOR ( 'NONE', #5906, 1000.000000000000000 ) ;
#6342=EDGE_CURVE ( 'NONE', #11008, #929, #11155, .T. ) ;
#6343=VECTOR ( 'NONE', #11063, 1000.000000000000000 ) ;
#6346=CARTESIAN_POINT ( 'NONE',  ( 174.5152310637604387, -9.999999999999994671, -11.28819510263909542 ) ) ;
#6349=VECTOR ( 'NONE', #21442, 1000.000000000000000 ) ;
#6351=CARTESIAN_POINT ( 'NONE',  ( 137.0152310637605808, -1.999999999999979572, -17.38167787843870826 ) ) ;
#6352=CARTESIAN_POINT ( 'NONE',  ( 133.6922820468854241, -1.999999999999981348, -15.07341522555727309 ) ) ;
#6353=LINE ( 'NONE', #8476, #4334 ) ;
#6359=LINE ( 'NONE', #25122, #23682 ) ;
#6361=CARTESIAN_POINT ( 'NONE',  ( 136.1922820468854241, -10.00000000000000533, -13.59645775552055547 ) ) ;
#6362=DIRECTION ( 'NONE',  ( -0.9510565162951536422, -2.566386769018988816E-16, -0.3090169943749472292 ) ) ;
#6364=CARTESIAN_POINT ( 'NONE',  ( 154.7287565553230024, -1.999999999999974021, -25.16025403784440329 ) ) ;
#6365=CARTESIAN_POINT ( 'NONE',  ( 142.2287565553230309, -10.00000000000000533, -12.16987298107780369 ) ) ;
#6367=ADVANCED_FACE ( 'NONE', ( #9147 ), #18631, .T. ) ;
#6368=ADVANCED_FACE ( 'NONE', ( #16185 ), #6736, .T. ) ;
#6370=LINE ( 'NONE', #12917, #5675 ) ;
#6371=CARTESIAN_POINT ( 'NONE',  ( 176.1922820468853388, -9.999999999999994671, -30.91696583120936026 ) ) ;
#6372=EDGE_CURVE ( 'NONE', #9595, #15913, #7039, .T. ) ;
#6373=CARTESIAN_POINT ( 'NONE',  ( 162.0152310637604955, -9.999999999999998224, -26.04193191628311155 ) ) ;
#6374=ORIENTED_EDGE ( 'NONE', *, *, #16959, .F. ) ;
#6375=ORIENTED_EDGE ( 'NONE', *, *, #10559, .F. ) ;
#6380=VECTOR ( 'NONE', #18965, 1000.000000000000000 ) ;
#6383=CARTESIAN_POINT ( 'NONE',  ( 134.5152310637605808, -10.00000000000000533, -11.28819510263909187 ) ) ;
#6386=EDGE_LOOP ( 'NONE', ( #8265, #17702, #14316, #10337 ) ) ;
#6387=DIRECTION ( 'NONE',  ( -0.5877852522924731371, -1.586114251531760235E-16, 0.8090169943749474513 ) ) ;
#6388=CARTESIAN_POINT ( 'NONE',  ( 152.0152310637604955, -10.00000000000000178, -15.61832212156129351 ) ) ;
#6389=ORIENTED_EDGE ( 'NONE', *, *, #3982, .F. ) ;
#6390=CARTESIAN_POINT ( 'NONE',  ( 134.7287565553230024, -1.999999999999980460, -25.16025403784439973 ) ) ;
#6391=DIRECTION ( 'NONE',  ( 0.3090169943749475623, 8.338696094058001131E-17, 0.9510565162951536422 ) ) ;
#6392=VECTOR ( 'NONE', #24987, 1000.000000000000000 ) ;
#6395=EDGE_LOOP ( 'NONE', ( #13261, #15694, #18419, #27452 ) ) ;
#6396=VECTOR ( 'NONE', #6585, 1000.000000000000000 ) ;
#6398=EDGE_LOOP ( 'NONE', ( #15075, #22901, #9265, #14465 ) ) ;
#6400=FACE_OUTER_BOUND ( 'NONE', #27355, .T. ) ;
#6402=DIRECTION ( 'NONE',  ( -2.698458740408365879E-16, 1.000000000000000000, 0.000000000000000000 ) ) ;
#6403=EDGE_CURVE ( 'NONE', #11673, #25136, #4739, .T. ) ;
#6405=ORIENTED_EDGE ( 'NONE', *, *, #9301, .T. ) ;
#6406=DIRECTION ( 'NONE',  ( 1.110223024625156540E-16, 2.995891024602366092E-32, 1.000000000000000000 ) ) ;
#6407=EDGE_CURVE ( 'NONE', #1746, #22518, #29849, .T. ) ;
#6410=EDGE_CURVE ( 'NONE', #12130, #8557, #18475, .T. ) ;
#6411=DIRECTION ( 'NONE',  ( -0.9510565162951536422, -2.566386769018988323E-16, 0.3090169943749475623 ) ) ;
#6412=ORIENTED_EDGE ( 'NONE', *, *, #9858, .F. ) ;
#6416=ORIENTED_EDGE ( 'NONE', *, *, #27182, .F. ) ;
#6418=DIRECTION ( 'NONE',  ( 0.3090169943749472292, 8.338696094057992503E-17, -0.9510565162951536422 ) ) ;
#6419=VECTOR ( 'NONE', #21595, 1000.000000000000000 ) ;
#6420=AXIS2_PLACEMENT_3D ( 'NONE', #15016, #24345, #3443 ) ;
#6422=EDGE_LOOP ( 'NONE', ( #29806, #28571, #24361, #4126 ) ) ;
#6423=DIRECTION ( 'NONE',  ( -1.110223024625156540E-16, 0.000000000000000000, -1.000000000000000000 ) ) ;
#6424=CARTESIAN_POINT ( 'NONE',  ( 158.6922820468853104, -1.999999999999974465, 2.247092850131519715 ) ) ;
#6426=LINE ( 'NONE', #24898, #4862 ) ;
#6428=DIRECTION ( 'NONE',  ( 2.908569913943825554E-16, -1.000000000000000000, 0.000000000000000000 ) ) ;
#6429=VERTEX_POINT ( 'NONE', #29991 ) ;
#6434=ORIENTED_EDGE ( 'NONE', *, *, #25521, .F. ) ;
#6436=ADVANCED_FACE ( 'NONE', ( #2476 ), #13741, .T. ) ;
#6440=EDGE_CURVE ( 'NONE', #6518, #29309, #30141, .T. ) ;
#6441=ORIENTED_EDGE ( 'NONE', *, *, #12071, .F. ) ;
#6442=CARTESIAN_POINT ( 'NONE',  ( 132.0152310637605808, -1.999999999999981348, -6.958068083716893781 ) ) ;
#6443=ADVANCED_FACE ( 'NONE', ( #27830 ), #8855, .T. ) ;
#6449=DIRECTION ( 'NONE',  ( -2.698458740408365879E-16, 1.000000000000000000, 0.000000000000000000 ) ) ;
#6453=VERTEX_POINT ( 'NONE', #28130 ) ;
#6454=VECTOR ( 'NONE', #1885, 1000.000000000000000 ) ;
#6455=ORIENTED_EDGE ( 'NONE', *, *, #19996, .T. ) ;
#6456=CARTESIAN_POINT ( 'NONE',  ( 164.7287565553229740, -9.999999999999998224, -33.82050807568879947 ) ) ;
#6458=DIRECTION ( 'NONE',  ( -1.000000000000000000, -2.908569913943825554E-16, 0.000000000000000000 ) ) ;
#6459=VECTOR ( 'NONE', #10980, 1000.000000000000000 ) ;
#6460=DIRECTION ( 'NONE',  ( 0.3090169943749472292, 8.338696094057992503E-17, -0.9510565162951536422 ) ) ;
#6464=ORIENTED_EDGE ( 'NONE', *, *, #13008, .T. ) ;
#6465=CARTESIAN_POINT ( 'NONE',  ( 130.7287565553229172, -4.999999999999983125, -28.21440484423857242 ) ) ;
#6466=EDGE_LOOP ( 'NONE', ( #26352, #21118, #5879, #6910, #26741 ) ) ;
#6468=EDGE_CURVE ( 'NONE', #26900, #10926, #1875, .T. ) ;
#6469=AXIS2_PLACEMENT_3D ( 'NONE', #17359, #12631, #898 ) ;
#6470=FACE_OUTER_BOUND ( 'NONE', #1254, .T. ) ;
#6473=CARTESIAN_POINT ( 'NONE',  ( 26.10647222977721071, -5.000000000000010658, -80.34745979530829629 ) ) ;
#6474=EDGE_CURVE ( 'NONE', #7790, #25049, #20907, .T. ) ;
#6476=EDGE_LOOP ( 'NONE', ( #7891, #624, #7449, #1224 ) ) ;
#6477=VERTEX_POINT ( 'NONE', #15874 ) ;
#6478=LINE ( 'NONE', #20643, #23726 ) ;
#6479=EDGE_CURVE ( 'NONE', #17865, #7141, #9307, .T. ) ;
#6482=LINE ( 'NONE', #4336, #6903 ) ;
#6486=ORIENTED_EDGE ( 'NONE', *, *, #8617, .F. ) ;
#6487=DIRECTION ( 'NONE',  ( -0.9510565162951536422, -2.566386769018988816E-16, -0.3090169943749472292 ) ) ;
#6490=ORIENTED_EDGE ( 'NONE', *, *, #10410, .F. ) ;
#6492=CARTESIAN_POINT ( 'NONE',  ( 166.1922820468853672, -9.999999999999998224, -22.25671179336496053 ) ) ;
#6494=FACE_OUTER_BOUND ( 'NONE', #7878, .T. ) ;
#6495=VERTEX_POINT ( 'NONE', #8185 ) ;
#6496=EDGE_CURVE ( 'NONE', #10227, #10342, #24381, .T. ) ;
#6497=CARTESIAN_POINT ( 'NONE',  ( 157.0152310637604955, -1.999999999999974465, -6.958068083716895558 ) ) ;
#6498=LINE ( 'NONE', #15939, #9156 ) ;
#6499=DIRECTION ( 'NONE',  ( 0.9510565162951536422, 2.566386769018988816E-16, 0.3090169943749472292 ) ) ;
#6500=CARTESIAN_POINT ( 'NONE',  ( 149.5152310637604955, -10.00000000000000178, -4.391296821672111328 ) ) ;
#6504=CARTESIAN_POINT ( 'NONE',  ( 154.5152310637605808, -1.999999999999974021, -28.60870317832789667 ) ) ;
#6506=CARTESIAN_POINT ( 'NONE',  ( 15.93055805288878801, -5.000000000000013323, 49.02921625739047329 ) ) ;
#6507=CARTESIAN_POINT ( 'NONE',  ( 132.0152310637605524, -10.00000000000000711, -0.06116980274991495881 ) ) ;
#6510=ORIENTED_EDGE ( 'NONE', *, *, #5320, .F. ) ;
#6511=ORIENTED_EDGE ( 'NONE', *, *, #29568, .F. ) ;
#6512=DIRECTION ( 'NONE',  ( 0.9510565162951536422, 2.566386769018988816E-16, 0.3090169943749472292 ) ) ;
#6513=EDGE_CURVE ( 'NONE', #3997, #486, #2620, .T. ) ;
#6516=CARTESIAN_POINT ( 'NONE',  ( 159.5152310637604955, -1.999999999999973577, -11.28819510263909542 ) ) ;
#6517=LINE ( 'NONE', #15807, #22976 ) ;
#6518=VERTEX_POINT ( 'NONE', #884 ) ;
#6519=PLANE ( 'NONE',  #24895 ) ;
#6520=VECTOR ( 'NONE', #28347, 1000.000000000000000 ) ;
#6521=ORIENTED_EDGE ( 'NONE', *, *, #2826, .T. ) ;
#6526=CARTESIAN_POINT ( 'NONE',  ( 137.2287565553230309, -10.00000000000000533, -29.49038105676660138 ) ) ;
#6528=VERTEX_POINT ( 'NONE', #29147 ) ;
#6529=DIRECTION ( 'NONE',  ( -0.5877852522924731371, 0.000000000000000000, 0.8090169943749474513 ) ) ;
#6530=EDGE_CURVE ( 'NONE', #4371, #12000, #10470, .T. ) ;
#6532=VERTEX_POINT ( 'NONE', #22233 ) ;
#6533=DIRECTION ( 'NONE',  ( 0.9510565162951536422, 2.566386769018988816E-16, 0.3090169943749472292 ) ) ;
#6534=DIRECTION ( 'NONE',  ( -0.5877852522924731371, -1.586114251531760235E-16, 0.8090169943749474513 ) ) ;
#6536=ORIENTED_EDGE ( 'NONE', *, *, #4198, .T. ) ;
#6537=DIRECTION ( 'NONE',  ( 0.5877852522924731371, 1.586114251531760728E-16, 0.8090169943749474513 ) ) ;
#6539=VERTEX_POINT ( 'NONE', #17054 ) ;
#6541=ORIENTED_EDGE ( 'NONE', *, *, #27650, .T. ) ;
#6543=CARTESIAN_POINT ( 'NONE',  ( 162.0152310637605240, -1.999999999999972244, -24.27857615940569502 ) ) ;
#6545=CARTESIAN_POINT ( 'NONE',  ( 172.7287565553229456, -9.999999999999971578, 3.500000000000003109 ) ) ;
#6546=EDGE_LOOP ( 'NONE', ( #11198, #11163, #24453, #18438 ) ) ;
#6547=ORIENTED_EDGE ( 'NONE', *, *, #29831, .F. ) ;
#6548=CARTESIAN_POINT ( 'NONE',  ( 156.1922820468853388, -10.00000000000000178, -4.936203717676158398 ) ) ;
#6549=CARTESIAN_POINT ( 'NONE',  ( 139.5152310637605524, -1.999999999999979128, -4.391296821672111328 ) ) ;
#6550=LINE ( 'NONE', #17683, #13533 ) ;
#6551=ORIENTED_EDGE ( 'NONE', *, *, #17179, .T. ) ;
#6552=DIRECTION ( 'NONE',  ( -0.9510565162951536422, -2.566386769018988816E-16, -0.3090169943749472292 ) ) ;
#6553=VERTEX_POINT ( 'NONE', #21784 ) ;
#6555=VERTEX_POINT ( 'NONE', #19488 ) ;
#6558=VERTEX_POINT ( 'NONE', #10172 ) ;
#6560=CARTESIAN_POINT ( 'NONE',  ( 136.1922820468854241, -1.999999999999980460, -10.74328820663507322 ) ) ;
#6561=VECTOR ( 'NONE', #6045, 1000.000000000000000 ) ;
#6563=CARTESIAN_POINT ( 'NONE',  ( 163.6922820468853388, -1.999999999999972689, -17.92658477444275889 ) ) ;
#6565=ORIENTED_EDGE ( 'NONE', *, *, #24880, .T. ) ;
#6567=EDGE_CURVE ( 'NONE', #5949, #13402, #19333, .T. ) ;
#6568=DIRECTION ( 'NONE',  ( 0.5877852522924731371, 1.586114251531760728E-16, 0.8090169943749474513 ) ) ;
#6570=ADVANCED_FACE ( 'NONE', ( #24085 ), #3186, .T. ) ;
#6571=EDGE_CURVE ( 'NONE', #24722, #28182, #17202, .T. ) ;
#6575=LINE ( 'NONE', #25192, #25334 ) ;
#6576=ORIENTED_EDGE ( 'NONE', *, *, #13069, .T. ) ;
#6577=ORIENTED_EDGE ( 'NONE', *, *, #27289, .T. ) ;
#6578=CARTESIAN_POINT ( 'NONE',  ( 164.7287565553229172, -1.999999999999971800, -16.50000000000000355 ) ) ;
#6582=VERTEX_POINT ( 'NONE', #7893 ) ;
#6583=CARTESIAN_POINT ( 'NONE',  ( 171.1922820468853672, -1.999999999999970024, -30.91696583120936026 ) ) ;
#6585=DIRECTION ( 'NONE',  ( -1.110223024625156540E-16, 0.000000000000000000, -1.000000000000000000 ) ) ;
#6587=ORIENTED_EDGE ( 'NONE', *, *, #22792, .F. ) ;
#6588=PLANE ( 'NONE',  #21268 ) ;
#6589=ORIENTED_EDGE ( 'NONE', *, *, #30190, .T. ) ;
#6593=CARTESIAN_POINT ( 'NONE',  ( 137.0152310637605808, -4.999999999999980460, -1.521174642513229767E-14 ) ) ;
#6594=CARTESIAN_POINT ( 'NONE',  ( 130.7287565553229456, -4.999999999999983125, 3.500000000000003109 ) ) ;
#6598=VECTOR ( 'NONE', #26753, 1000.000000000000000 ) ;
#6599=ORIENTED_EDGE ( 'NONE', *, *, #3403, .T. ) ;
#6600=LINE ( 'NONE', #4163, #29443 ) ;
#6601=EDGE_CURVE ( 'NONE', #29946, #5949, #5612, .T. ) ;
#6603=EDGE_CURVE ( 'NONE', #27886, #15011, #17344, .T. ) ;
#6605=DIRECTION ( 'NONE',  ( -2.698458740408365879E-16, 1.000000000000000000, 0.000000000000000000 ) ) ;
#6606=DIRECTION ( 'NONE',  ( 0.9510565162951536422, 2.566386769018988816E-16, 0.3090169943749472292 ) ) ;
#6609=DIRECTION ( 'NONE',  ( -2.698458740408365879E-16, 1.000000000000000000, 0.000000000000000000 ) ) ;
#6611=ORIENTED_EDGE ( 'NONE', *, *, #28665, .T. ) ;
#6612=VECTOR ( 'NONE', #13067, 1000.000000000000000 ) ;
#6616=CARTESIAN_POINT ( 'NONE',  ( 129.5152310637605524, -1.999999999999982236, -13.05155085951650840 ) ) ;
#6617=DIRECTION ( 'NONE',  ( 0.5877852522924731371, 1.586114251531760728E-16, 0.8090169943749474513 ) ) ;
#6618=ORIENTED_EDGE ( 'NONE', *, *, #23106, .F. ) ;
#6620=ORIENTED_EDGE ( 'NONE', *, *, #27483, .F. ) ;
#6621=ORIENTED_EDGE ( 'NONE', *, *, #23772, .T. ) ;
#6622=CARTESIAN_POINT ( 'NONE',  ( 132.0152310637605524, -10.00000000000000711, -34.70218595412750773 ) ) ;
#6626=DIRECTION ( 'NONE',  ( -0.8090169943749474513, -2.183098979609982436E-16, 0.5877852522924731371 ) ) ;
#6630=ORIENTED_EDGE ( 'NONE', *, *, #10380, .T. ) ;
#6631=CARTESIAN_POINT ( 'NONE',  ( 164.5152310637605240, -9.999999999999996447, -28.60870317832789667 ) ) ;
#6634=VECTOR ( 'NONE', #20235, 1000.000000000000000 ) ;
#6635=VERTEX_POINT ( 'NONE', #3334 ) ;
#6636=ORIENTED_EDGE ( 'NONE', *, *, #11341, .F. ) ;
#6637=CARTESIAN_POINT ( 'NONE',  ( 154.5152310637605524, -4.999999999999976019, -1.715463671822631846E-14 ) ) ;
#6639=EDGE_CURVE ( 'NONE', #22085, #4384, #26689, .T. ) ;
#6640=EDGE_CURVE ( 'NONE', #6979, #26011, #3476, .T. ) ;
#6641=VECTOR ( 'NONE', #15152, 1000.000000000000000 ) ;
#6642=EDGE_CURVE ( 'NONE', #26171, #23545, #19780, .T. ) ;
#6643=DIRECTION ( 'NONE',  ( 0.3090169943749475623, 8.338696094058001131E-17, 0.9510565162951536422 ) ) ;
#6645=DIRECTION ( 'NONE',  ( -0.5877852522924731371, -1.586114251531760235E-16, 0.8090169943749474513 ) ) ;
#6646=LINE ( 'NONE', #8619, #17443 ) ;
#6647=FACE_OUTER_BOUND ( 'NONE', #15415, .T. ) ;
#6648=LINE ( 'NONE', #27741, #914 ) ;
#6652=VERTEX_POINT ( 'NONE', #15200 ) ;
#6656=DIRECTION ( 'NONE',  ( 0.3090169943749475623, 8.338696094058001131E-17, 0.9510565162951536422 ) ) ;
#6657=DIRECTION ( 'NONE',  ( -0.9510565162951536422, -2.566386769018988816E-16, -0.3090169943749472292 ) ) ;
#6659=PLANE ( 'NONE',  #8277 ) ;
#6661=CARTESIAN_POINT ( 'NONE',  ( 177.2287565553229172, -9.999999999999994671, -29.49038105676660493 ) ) ;
#6663=EDGE_LOOP ( 'NONE', ( #29489, #16083, #23607, #19984 ) ) ;
#6664=VECTOR ( 'NONE', #4629, 1000.000000000000000 ) ;
#6665=DIRECTION ( 'NONE',  ( -1.110223024625156540E-16, 0.000000000000000000, -1.000000000000000000 ) ) ;
#6666=CARTESIAN_POINT ( 'NONE',  ( 133.7287565553229172, -4.000000000000003553, -41.50000000000000000 ) ) ;
#6668=AXIS2_PLACEMENT_3D ( 'NONE', #10878, #27268, #22646 ) ;
#6669=CARTESIAN_POINT ( 'NONE',  ( 172.7287565553229456, -9.999999999999980460, -41.50000000000000711 ) ) ;
#6671=ORIENTED_EDGE ( 'NONE', *, *, #3644, .F. ) ;
#6676=CARTESIAN_POINT ( 'NONE',  ( 163.6922820468853956, -4.999999999999973355, -32.39392330124607611 ) ) ;
#6679=AXIS2_PLACEMENT_3D ( 'NONE', #30039, #11054, #2070 ) ;
#6680=VERTEX_POINT ( 'NONE', #10019 ) ;
#6681=ADVANCED_FACE ( 'NONE', ( #27154 ), #20682, .T. ) ;
#6682=PLANE ( 'NONE',  #29452 ) ;
#6683=EDGE_CURVE ( 'NONE', #22665, #25015, #10928, .T. ) ;
#6685=ORIENTED_EDGE ( 'NONE', *, *, #19856, .T. ) ;
#6686=VECTOR ( 'NONE', #6411, 999.9999999999998863 ) ;
#6687=VERTEX_POINT ( 'NONE', #24688 ) ;
#6689=CARTESIAN_POINT ( 'NONE',  ( 169.5152310637604387, -1.999999999999971356, -2.627941064794695691 ) ) ;
#6690=CARTESIAN_POINT ( 'NONE',  ( 131.1922820468854241, -4.999999999999982236, -28.06379628232387446 ) ) ;
#6691=ORIENTED_EDGE ( 'NONE', *, *, #7497, .F. ) ;
#6693=VECTOR ( 'NONE', #1285, 1000.000000000000000 ) ;
#6695=EDGE_LOOP ( 'NONE', ( #15231, #3066, #5326, #4700 ) ) ;
#6699=CARTESIAN_POINT ( 'NONE',  ( 92.15659011758447150, -4.999999999999992006, 66.95568195638367115 ) ) ;
#6700=DIRECTION ( 'NONE',  ( 1.000000000000000000, 2.698458740408365879E-16, -1.110223024625156540E-16 ) ) ;
#6701=ORIENTED_EDGE ( 'NONE', *, *, #23422, .T. ) ;
#6702=CARTESIAN_POINT ( 'NONE',  ( 136.1922820468854241, -10.00000000000000533, -4.936203717676158398 ) ) ;
#6703=VECTOR ( 'NONE', #29069, 1000.000000000000000 ) ;
#6705=EDGE_LOOP ( 'NONE', ( #24685, #11756, #9320, #13185 ) ) ;
#6707=DIRECTION ( 'NONE',  ( -2.698458740408365879E-16, 1.000000000000000000, 0.000000000000000000 ) ) ;
#6708=ORIENTED_EDGE ( 'NONE', *, *, #6954, .F. ) ;
#6710=EDGE_CURVE ( 'NONE', #21232, #25023, #3929, .T. ) ;
#6715=DIRECTION ( 'NONE',  ( -2.698458740408365879E-16, 1.000000000000000000, 0.000000000000000000 ) ) ;
#6716=CARTESIAN_POINT ( 'NONE',  ( 169.7287565553229740, -9.999999999999996447, -33.82050807568879947 ) ) ;
#6719=CARTESIAN_POINT ( 'NONE',  ( 171.1922820468853672, -4.999999999999971578, -30.91696583120936026 ) ) ;
#6720=CARTESIAN_POINT ( 'NONE',  ( 169.5152310637604387, -1.999999999999970912, -13.05155085951651195 ) ) ;
#6721=VECTOR ( 'NONE', #10362, 1000.000000000000000 ) ;
#6724=LINE ( 'NONE', #2307, #23382 ) ;
#6727=ORIENTED_EDGE ( 'NONE', *, *, #4737, .F. ) ;
#6733=VERTEX_POINT ( 'NONE', #6666 ) ;
#6736=PLANE ( 'NONE',  #17105 ) ;
#6738=ORIENTED_EDGE ( 'NONE', *, *, #15367, .T. ) ;
#6746=EDGE_CURVE ( 'NONE', #22297, #7033, #24840, .T. ) ;
#6747=VECTOR ( 'NONE', #24822, 1000.000000000000000 ) ;
#6748=CARTESIAN_POINT ( 'NONE',  ( 133.6922820468854241, -10.00000000000000711, 2.247092850131519715 ) ) ;
#6749=DIRECTION ( 'NONE',  ( 0.3090169943749472292, 8.338696094057992503E-17, -0.9510565162951536422 ) ) ;
#6752=VECTOR ( 'NONE', #14000, 1000.000000000000000 ) ;
#6754=ORIENTED_EDGE ( 'NONE', *, *, #23993, .T. ) ;
#6755=CARTESIAN_POINT ( 'NONE',  ( 20.21908482906315996, -5.000000000000012434, -62.22794451515765957 ) ) ;
#6757=CARTESIAN_POINT ( 'NONE',  ( 169.5152310637604671, -1.999999999999970912, -11.28819510263909542 ) ) ;
#6763=EDGE_LOOP ( 'NONE', ( #30100, #6098, #18821, #24033 ) ) ;
#6764=VECTOR ( 'NONE', #8294, 1000.000000000000000 ) ;
#6769=DIRECTION ( 'NONE',  ( 1.110223024625156540E-16, 2.995891024602366092E-32, 1.000000000000000000 ) ) ;
#6774=VERTEX_POINT ( 'NONE', #20236 ) ;
#6775=DIRECTION ( 'NONE',  ( 0.5877852522924731371, 1.586114251531760728E-16, -0.8090169943749474513 ) ) ;
#6777=ORIENTED_EDGE ( 'NONE', *, *, #6567, .F. ) ;
#6778=EDGE_CURVE ( 'NONE', #9083, #14185, #20538, .T. ) ;
#6779=AXIS2_PLACEMENT_3D ( 'NONE', #2750, #12187, #13055 ) ;
#6781=DIRECTION ( 'NONE',  ( 0.5877852522924731371, 1.586114251531760728E-16, 0.8090169943749474513 ) ) ;
#6782=ORIENTED_EDGE ( 'NONE', *, *, #17366, .F. ) ;
#6783=EDGE_CURVE ( 'NONE', #13070, #5527, #22551, .T. ) ;
#6785=EDGE_CURVE ( 'NONE', #3713, #22665, #4374, .T. ) ;
#6787=ORIENTED_EDGE ( 'NONE', *, *, #9162, .T. ) ;
#6788=LINE ( 'NONE', #28026, #19320 ) ;
#6792=ORIENTED_EDGE ( 'NONE', *, *, #13566, .T. ) ;
#6793=CARTESIAN_POINT ( 'NONE',  ( 143.6922820468854525, -10.00000000000000355, -17.92658477444275889 ) ) ;
#6794=VECTOR ( 'NONE', #20005, 1000.000000000000000 ) ;
#6795=DIRECTION ( 'NONE',  ( 0.5877852522924731371, 1.586114251531760728E-16, -0.8090169943749474513 ) ) ;
#6797=ORIENTED_EDGE ( 'NONE', *, *, #11613, .F. ) ;
#6799=DIRECTION ( 'NONE',  ( 1.000000000000000000, 2.168404344971006896E-16, 0.000000000000000000 ) ) ;
#6800=LINE ( 'NONE', #9057, #3828 ) ;
#6801=CARTESIAN_POINT ( 'NONE',  ( 144.5152310637605808, -10.00000000000000355, -11.28819510263909542 ) ) ;
#6802=CARTESIAN_POINT ( 'NONE',  ( 172.0152310637604671, -9.999999999999994671, -15.61832212156129707 ) ) ;
#6807=DIRECTION ( 'NONE',  ( -0.9510565162951536422, 0.000000000000000000, -0.3090169943749472292 ) ) ;
#6812=ORIENTED_EDGE ( 'NONE', *, *, #17074, .T. ) ;
#6813=DIRECTION ( 'NONE',  ( 0.9510565162951536422, 2.566386769018988816E-16, 0.3090169943749472292 ) ) ;
#6815=ORIENTED_EDGE ( 'NONE', *, *, #16699, .F. ) ;
#6816=AXIS2_PLACEMENT_3D ( 'NONE', #15988, #18436, #23163 ) ;
#6817=DIRECTION ( 'NONE',  ( -0.9510565162951536422, -2.566386769018988816E-16, -0.3090169943749472292 ) ) ;
#6818=DIRECTION ( 'NONE',  ( -0.5877852522924731371, -1.586114251531760235E-16, 0.8090169943749474513 ) ) ;
#6820=LINE ( 'NONE', #27466, #29334 ) ;
#6821=EDGE_CURVE ( 'NONE', #7982, #7358, #13372, .T. ) ;
#6825=EDGE_LOOP ( 'NONE', ( #7150, #20706, #4882, #3677, #23875 ) ) ;
#6826=EDGE_CURVE ( 'NONE', #27678, #25209, #17941, .T. ) ;
#6833=ORIENTED_EDGE ( 'NONE', *, *, #22246, .T. ) ;
#6834=CARTESIAN_POINT ( 'NONE',  ( 167.0152310637604955, -9.999999999999996447, -15.61832212156129707 ) ) ;
#6838=VERTEX_POINT ( 'NONE', #9079 ) ;
#6841=CARTESIAN_POINT ( 'NONE',  ( 148.6922820468853672, -10.00000000000000355, -0.6060766987539614181 ) ) ;
#6842=VECTOR ( 'NONE', #14730, 1000.000000000000000 ) ;
#6843=LINE ( 'NONE', #25589, #3419 ) ;
#6846=ORIENTED_EDGE ( 'NONE', *, *, #26970, .T. ) ;
#6847=CARTESIAN_POINT ( 'NONE',  ( 76.63953071969194752, -4.999999999999996447, 55.68187839422949281 ) ) ;
#6848=LINE ( 'NONE', #13984, #12853 ) ;
#6851=CARTESIAN_POINT ( 'NONE',  ( 153.6922820468854525, -4.999999999999975131, -32.39392330124607611 ) ) ;
#6853=VERTEX_POINT ( 'NONE', #17794 ) ;
#6855=PLANE ( 'NONE',  #1257 ) ;
#6856=EDGE_CURVE ( 'NONE', #29309, #10540, #27757, .T. ) ;
#6859=ADVANCED_FACE ( 'NONE', ( #22696 ), #13072, .T. ) ;
#6861=VERTEX_POINT ( 'NONE', #11235 ) ;
#6862=EDGE_CURVE ( 'NONE', #10393, #25794, #29777, .T. ) ;
#6864=AXIS2_PLACEMENT_3D ( 'NONE', #17071, #14615, #15065 ) ;
#6868=CARTESIAN_POINT ( 'NONE',  ( 137.0152310637605808, -1.999999999999979572, -17.38167787843870826 ) ) ;
#6869=CARTESIAN_POINT ( 'NONE',  ( 172.0152310637604103, -1.999999999999970912, 1.702185954127501066 ) ) ;
#6870=DIRECTION ( 'NONE',  ( 0.9510565162951535312, 2.566386769018988816E-16, -0.3090169943749475623 ) ) ;
#6872=CARTESIAN_POINT ( 'NONE',  ( 130.7287565553229456, -4.999999999999983125, 3.500000000000003109 ) ) ;
#6873=VECTOR ( 'NONE', #13549, 1000.000000000000000 ) ;
#6875=DIRECTION ( 'NONE',  ( -2.698458740408365879E-16, 1.000000000000000000, 0.000000000000000000 ) ) ;
#6877=FACE_OUTER_BOUND ( 'NONE', #6271, .T. ) ;
#6878=DIRECTION ( 'NONE',  ( 0.5877852522924731371, 1.586114251531760728E-16, 0.8090169943749474513 ) ) ;
#6879=EDGE_CURVE ( 'NONE', #10809, #23695, #6517, .T. ) ;
#6883=CARTESIAN_POINT ( 'NONE',  ( 143.6922820468854525, -1.999999999999978684, -32.39392330124607611 ) ) ;
#6884=ORIENTED_EDGE ( 'NONE', *, *, #18246, .T. ) ;
#6885=ORIENTED_EDGE ( 'NONE', *, *, #14907, .F. ) ;
#6890=VERTEX_POINT ( 'NONE', #1499 ) ;
#6891=VERTEX_POINT ( 'NONE', #16257 ) ;
#6892=EDGE_LOOP ( 'NONE', ( #7849, #29201, #1624, #4134, #13677 ) ) ;
#6895=LINE ( 'NONE', #27531, #25872 ) ;
#6896=CARTESIAN_POINT ( 'NONE',  ( 162.2287565553229740, -1.999999999999971800, -29.49038105676660493 ) ) ;
#6897=EDGE_LOOP ( 'NONE', ( #21228, #15480, #10400, #2353 ) ) ;
#6898=CARTESIAN_POINT ( 'NONE',  ( 153.6922820468854525, -1.999999999999974465, -35.24709285013155835 ) ) ;
#6903=VECTOR ( 'NONE', #1461, 1000.000000000000000 ) ;
#6910=ORIENTED_EDGE ( 'NONE', *, *, #23626, .T. ) ;
#6911=DIRECTION ( 'NONE',  ( -2.698458740408365879E-16, 1.000000000000000000, 0.000000000000000000 ) ) ;
#6912=ADVANCED_FACE ( 'NONE', ( #4522 ), #6970, .T. ) ;
#6913=CARTESIAN_POINT ( 'NONE',  ( 5.430258561686096108, -5.000000000000015987, 16.71261737790626256 ) ) ;
#6914=FACE_OUTER_BOUND ( 'NONE', #11035, .T. ) ;
#6915=EDGE_CURVE ( 'NONE', #25136, #18177, #13810, .T. ) ;
#6916=DIRECTION ( 'NONE',  ( -2.698458740408365879E-16, 1.000000000000000000, 0.000000000000000000 ) ) ;
#6918=DIRECTION ( 'NONE',  ( 2.908569913943826047E-16, -1.000000000000000000, 6.826925868028107924E-18 ) ) ;
#6919=ORIENTED_EDGE ( 'NONE', *, *, #19274, .F. ) ;
#6920=DIRECTION ( 'NONE',  ( -2.698458740408365879E-16, 1.000000000000000000, 0.000000000000000000 ) ) ;
#6923=AXIS2_PLACEMENT_3D ( 'NONE', #1136, #14837, #24174 ) ;
#6925=LINE ( 'NONE', #11630, #38 ) ;
#6926=DIRECTION ( 'NONE',  ( -2.698458740408365879E-16, 1.000000000000000000, 0.000000000000000000 ) ) ;
#6928=EDGE_LOOP ( 'NONE', ( #13375, #29027, #7026, #15865, #23302 ) ) ;
#6929=ORIENTED_EDGE ( 'NONE', *, *, #7533, .T. ) ;
#6934=ORIENTED_EDGE ( 'NONE', *, *, #28151, .T. ) ;
#6935=CARTESIAN_POINT ( 'NONE',  ( 172.2287565553229456, -9.999999999999994671, -29.49038105676660493 ) ) ;
#6936=VECTOR ( 'NONE', #17837, 1000.000000000000000 ) ;
#6938=ORIENTED_EDGE ( 'NONE', *, *, #13349, .T. ) ;
#6939=CARTESIAN_POINT ( 'NONE',  ( 153.6922820468854241, -10.00000000000000000, -23.73366926340167637 ) ) ;
#6943=EDGE_LOOP ( 'NONE', ( #28134, #12008, #8971, #8894 ) ) ;
#6946=CARTESIAN_POINT ( 'NONE',  ( 157.0152310637604387, -1.999999999999974909, -0.06116980274991495881 ) ) ;
#6947=EDGE_CURVE ( 'NONE', #19572, #20829, #30217, .T. ) ;
#6948=EDGE_CURVE ( 'NONE', #2774, #7135, #9227, .T. ) ;
#6949=DIRECTION ( 'NONE',  ( -0.5877852522924731371, -1.586114251531760728E-16, -0.8090169943749474513 ) ) ;
#6950=VERTEX_POINT ( 'NONE', #2248 ) ;
#6952=PLANE ( 'NONE',  #8482 ) ;
#6953=VECTOR ( 'NONE', #19425, 1000.000000000000000 ) ;
#6954=EDGE_CURVE ( 'NONE', #10786, #2363, #26043, .T. ) ;
#6960=CARTESIAN_POINT ( 'NONE',  ( 119.3579561578551562, -4.999999999999985789, -86.71863120448111317 ) ) ;
#6961=LINE ( 'NONE', #16249, #19551 ) ;
#6962=DIRECTION ( 'NONE',  ( -1.000000000000000000, -2.698458740408365879E-16, 0.000000000000000000 ) ) ;
#6963=DIRECTION ( 'NONE',  ( -2.698458740408365879E-16, 1.000000000000000000, 0.000000000000000000 ) ) ;
#6964=ORIENTED_EDGE ( 'NONE', *, *, #19238, .F. ) ;
#6965=DIRECTION ( 'NONE',  ( 0.5877852522924731371, 1.586114251531760728E-16, -0.8090169943749474513 ) ) ;
#6969=PLANE ( 'NONE',  #13456 ) ;
#6970=PLANE ( 'NONE',  #567 ) ;
#6972=ORIENTED_EDGE ( 'NONE', *, *, #26601, .T. ) ;
#6977=VECTOR ( 'NONE', #28676, 1000.000000000000000 ) ;
#6979=VERTEX_POINT ( 'NONE', #16723 ) ;
#6980=DIRECTION ( 'NONE',  ( 0.9510565162951536422, 0.000000000000000000, -0.3090169943749475623 ) ) ;
#6981=DIRECTION ( 'NONE',  ( -2.698458740408365879E-16, 1.000000000000000000, 0.000000000000000000 ) ) ;
#6983=VERTEX_POINT ( 'NONE', #27911 ) ;
#6984=ADVANCED_FACE ( 'NONE', ( #7267 ), #23290, .T. ) ;
#6985=PLANE ( 'NONE',  #4614 ) ;
#6986=EDGE_CURVE ( 'NONE', #23467, #19109, #14192, .T. ) ;
#6987=EDGE_CURVE ( 'NONE', #17600, #4081, #14411, .T. ) ;
#6991=ORIENTED_EDGE ( 'NONE', *, *, #28381, .T. ) ;
#6992=AXIS2_PLACEMENT_3D ( 'NONE', #28193, #23890, #7248 ) ;
#6993=CARTESIAN_POINT ( 'NONE',  ( 162.0152310637605524, -1.999999999999971800, -32.93883019725009120 ) ) ;
#6996=CARTESIAN_POINT ( 'NONE',  ( 159.7287565553230024, -1.999999999999972244, -33.82050807568879947 ) ) ;
#6997=FACE_OUTER_BOUND ( 'NONE', #22827, .T. ) ;
#7000=DIRECTION ( 'NONE',  ( -0.9510565162951536422, -2.566386769018988816E-16, -0.3090169943749472292 ) ) ;
#7002=EDGE_LOOP ( 'NONE', ( #6247, #22653, #10221, #1072 ) ) ;
#7009=CARTESIAN_POINT ( 'NONE',  ( 143.6922820468853956, -10.00000000000000533, -0.6060766987539614181 ) ) ;
#7010=CARTESIAN_POINT ( 'NONE',  ( 158.6922820468854241, -9.999999999999998224, -35.24709285013155835 ) ) ;
#7011=LINE ( 'NONE', #23331, #9363 ) ;
#7013=AXIS2_PLACEMENT_3D ( 'NONE', #25012, #4097, #29799 ) ;
#7014=LINE ( 'NONE', #16614, #2779 ) ;
#7015=LINE ( 'NONE', #27958, #25479 ) ;
#7017=EDGE_CURVE ( 'NONE', #29240, #8141, #254, .T. ) ;
#7018=EDGE_CURVE ( 'NONE', #29468, #23116, #20991, .T. ) ;
#7019=DIRECTION ( 'NONE',  ( -0.5877852522924731371, 0.000000000000000000, 0.8090169943749474513 ) ) ;
#7020=CARTESIAN_POINT ( 'NONE',  ( 132.2287565553230024, -1.999999999999981348, -3.509618943233403510 ) ) ;
#7021=EDGE_CURVE ( 'NONE', #13222, #6861, #2692, .T. ) ;
#7022=EDGE_CURVE ( 'NONE', #25081, #10203, #9531, .T. ) ;
#7026=ORIENTED_EDGE ( 'NONE', *, *, #5327, .T. ) ;
#7028=VERTEX_POINT ( 'NONE', #14260 ) ;
#7029=DIRECTION ( 'NONE',  ( -1.110223024625156540E-16, 0.000000000000000000, -1.000000000000000000 ) ) ;
#7032=LINE ( 'NONE', #13432, #24858 ) ;
#7033=VERTEX_POINT ( 'NONE', #98 ) ;
#7039=LINE ( 'NONE', #21067, #10271 ) ;
#7040=FACE_OUTER_BOUND ( 'NONE', #924, .T. ) ;
#7041=VERTEX_POINT ( 'NONE', #16111 ) ;
#7042=LINE ( 'NONE', #14034, #24226 ) ;
#7043=ORIENTED_EDGE ( 'NONE', *, *, #5815, .F. ) ;
#7045=EDGE_LOOP ( 'NONE', ( #6541, #15446, #22071, #14491 ) ) ;
#7048=ORIENTED_EDGE ( 'NONE', *, *, #18941, .F. ) ;
#7049=FACE_OUTER_BOUND ( 'NONE', #23783, .T. ) ;
#7055=ORIENTED_EDGE ( 'NONE', *, *, #12445, .F. ) ;
#7056=FACE_BOUND ( 'NONE', #24704, .T. ) ;
#7058=EDGE_CURVE ( 'NONE', #23288, #26251, #28056, .T. ) ;
#7059=ADVANCED_FACE ( 'NONE', ( #16414 ), #25735, .T. ) ;
#7060=CARTESIAN_POINT ( 'NONE',  ( 137.2287565553230309, -1.999999999999979572, -29.49038105676660138 ) ) ;
#7061=LINE ( 'NONE', #21543, #18958 ) ;
#7062=FACE_OUTER_BOUND ( 'NONE', #11556, .T. ) ;
#7064=LINE ( 'NONE', #2352, #25078 ) ;
#7065=ORIENTED_EDGE ( 'NONE', *, *, #13610, .F. ) ;
#7066=DIRECTION ( 'NONE',  ( -0.5877852522924731371, -1.586114251531760235E-16, 0.8090169943749474513 ) ) ;
#7067=ORIENTED_EDGE ( 'NONE', *, *, #1804, .T. ) ;
#7069=ORIENTED_EDGE ( 'NONE', *, *, #15291, .F. ) ;
#7071=CARTESIAN_POINT ( 'NONE',  ( 133.6922820468854241, -10.00000000000000711, -35.24709285013155835 ) ) ;
#7072=DIRECTION ( 'NONE',  ( 0.5877852522924731371, 1.586114251531760728E-16, -0.8090169943749474513 ) ) ;
#7074=ORIENTED_EDGE ( 'NONE', *, *, #8524, .T. ) ;
#7075=CARTESIAN_POINT ( 'NONE',  ( 23.08382991343894020, -5.000000000000011546, -71.04472329954472798 ) ) ;
#7078=DIRECTION ( 'NONE',  ( 0.9510565162951536422, 0.000000000000000000, -0.3090169943749475623 ) ) ;
#7079=VECTOR ( 'NONE', #4585, 1000.000000000000000 ) ;
#7080=ADVANCED_FACE ( 'NONE', ( #24057 ), #19600, .T. ) ;
#7081=CARTESIAN_POINT ( 'NONE',  ( 163.6922820468853956, -1.999999999999971800, -35.24709285013155835 ) ) ;
#7083=VERTEX_POINT ( 'NONE', #19747 ) ;
#7084=DIRECTION ( 'NONE',  ( -2.698458740408365879E-16, 1.000000000000000000, 0.000000000000000000 ) ) ;
#7085=EDGE_CURVE ( 'NONE', #10807, #1890, #5276, .T. ) ;
#7088=ORIENTED_EDGE ( 'NONE', *, *, #13757, .T. ) ;
#7089=DIRECTION ( 'NONE',  ( -2.698458740408365879E-16, 1.000000000000000000, 0.000000000000000000 ) ) ;
#7091=ORIENTED_EDGE ( 'NONE', *, *, #15854, .F. ) ;
#7092=CARTESIAN_POINT ( 'NONE',  ( 156.1922820468853672, -4.999999999999976019, -13.59645775552055902 ) ) ;
#7093=PLANE ( 'NONE',  #9269 ) ;
#7094=FACE_OUTER_BOUND ( 'NONE', #27794, .T. ) ;
#7095=VECTOR ( 'NONE', #5721, 1000.000000000000000 ) ;
#7100=ORIENTED_EDGE ( 'NONE', *, *, #23136, .F. ) ;
#7102=DIRECTION ( 'NONE',  ( 0.3090169943749472292, 8.338696094057992503E-17, -0.9510565162951536422 ) ) ;
#7105=ORIENTED_EDGE ( 'NONE', *, *, #11828, .T. ) ;
#7106=CARTESIAN_POINT ( 'NONE',  ( 131.1922820468854241, -1.999999999999982236, -30.91696583120935671 ) ) ;
#7110=CARTESIAN_POINT ( 'NONE',  ( 109.9631552159402617, -4.999999999999987566, -79.89290877803512103 ) ) ;
#7113=VERTEX_POINT ( 'NONE', #26348 ) ;
#7115=ORIENTED_EDGE ( 'NONE', *, *, #231, .T. ) ;
#7117=EDGE_CURVE ( 'NONE', #19168, #29985, #23912, .T. ) ;
#7120=VECTOR ( 'NONE', #6775, 1000.000000000000000 ) ;
#7121=EDGE_CURVE ( 'NONE', #11338, #28260, #8006, .T. ) ;
#7123=VECTOR ( 'NONE', #5210, 1000.000000000000000 ) ;
#7125=VERTEX_POINT ( 'NONE', #12580 ) ;
#7126=EDGE_LOOP ( 'NONE', ( #20196, #1673, #5235, #3818, #9597 ) ) ;
#7129=ORIENTED_EDGE ( 'NONE', *, *, #11864, .T. ) ;
#7130=ORIENTED_EDGE ( 'NONE', *, *, #18694, .T. ) ;
#7131=CARTESIAN_POINT ( 'NONE',  ( 163.6922820468853388, -1.999999999999972244, -15.07341522555727664 ) ) ;
#7135=VERTEX_POINT ( 'NONE', #5428 ) ;
#7141=VERTEX_POINT ( 'NONE', #12430 ) ;
#7142=CARTESIAN_POINT ( 'NONE',  ( 152.0152310637605808, -1.999999999999974909, -24.27857615940569502 ) ) ;
#7143=ORIENTED_EDGE ( 'NONE', *, *, #1135, .T. ) ;
#7144=LINE ( 'NONE', #25463, #15374 ) ;
#7146=ORIENTED_EDGE ( 'NONE', *, *, #779, .T. ) ;
#7147=ORIENTED_EDGE ( 'NONE', *, *, #8524, .F. ) ;
#7148=ORIENTED_EDGE ( 'NONE', *, *, #27556, .F. ) ;
#7150=ORIENTED_EDGE ( 'NONE', *, *, #29044, .T. ) ;
#7152=VERTEX_POINT ( 'NONE', #10140 ) ;
#7153=ADVANCED_FACE ( 'NONE', ( #17170 ), #15165, .T. ) ;
#7155=ADVANCED_FACE ( 'NONE', ( #24501 ), #10437, .T. ) ;
#7156=ORIENTED_EDGE ( 'NONE', *, *, #15125, .F. ) ;
#7157=EDGE_CURVE ( 'NONE', #16501, #14857, #14563, .T. ) ;
#7159=VECTOR ( 'NONE', #4341, 1000.000000000000000 ) ;
#7160=LINE ( 'NONE', #21181, #26746 ) ;
#7161=DIRECTION ( 'NONE',  ( -0.9510565162951536422, -2.566386769018988816E-16, -0.3090169943749472292 ) ) ;
#7166=STYLED_ITEM ( 'NONE', ( #2299 ), #21992 ) ;
#7167=VERTEX_POINT ( 'NONE', #3590 ) ;
#7168=CARTESIAN_POINT ( 'NONE',  ( 157.0152310637605524, -4.999999999999975131, -1.743219247438260759E-14 ) ) ;
#7169=LINE ( 'NONE', #11569, #4048 ) ;
#7171=CARTESIAN_POINT ( 'NONE',  ( 152.0152310637605808, -4.999999999999976907, -1.687708096207003248E-14 ) ) ;
#7172=LINE ( 'NONE', #14167, #16766 ) ;
#7174=CARTESIAN_POINT ( 'NONE',  ( 141.1922820468854525, -1.999999999999978684, -22.25671179336495697 ) ) ;
#7176=ORIENTED_EDGE ( 'NONE', *, *, #2644, .T. ) ;
#7178=EDGE_LOOP ( 'NONE', ( #5553, #17019, #2064, #5245 ) ) ;
#7179=PLANE ( 'NONE',  #11938 ) ;
#7182=CARTESIAN_POINT ( 'NONE',  ( 132.2287565553230024, -1.999999999999981348, -20.83012701892220164 ) ) ;
#7183=ORIENTED_EDGE ( 'NONE', *, *, #24181, .F. ) ;
#7184=AXIS2_PLACEMENT_3D ( 'NONE', #23322, #2436, #21031 ) ;
#7186=CARTESIAN_POINT ( 'NONE',  ( 15.44827550661201876, -5.000000000000013323, -47.54490320444753593 ) ) ;
#7190=ORIENTED_EDGE ( 'NONE', *, *, #3033, .F. ) ;
#7194=EDGE_LOOP ( 'NONE', ( #29370, #3220, #22730, #21377, #18320 ) ) ;
#7199=DIRECTION ( 'NONE',  ( 0.3090169943749475623, 8.338696094058001131E-17, 0.9510565162951536422 ) ) ;
#7200=EDGE_CURVE ( 'NONE', #25128, #23660, #12881, .T. ) ;
#7201=EDGE_CURVE ( 'NONE', #5593, #29734, #3305, .T. ) ;
#7202=EDGE_CURVE ( 'NONE', #983, #17128, #5733, .T. ) ;
#7207=VECTOR ( 'NONE', #10207, 999.9999999999998863 ) ;
#7209=DIRECTION ( 'NONE',  ( -0.5877852522924731371, 0.000000000000000000, 0.8090169943749474513 ) ) ;
#7211=ORIENTED_EDGE ( 'NONE', *, *, #18721, .T. ) ;
#7213=VECTOR ( 'NONE', #19545, 1000.000000000000000 ) ;
#7214=DIRECTION ( 'NONE',  ( -0.5877852522924731371, -1.586114251531760235E-16, 0.8090169943749474513 ) ) ;
#7215=DIRECTION ( 'NONE',  ( 1.000000000000000000, 2.698458740408365879E-16, -1.110223024625156540E-16 ) ) ;
#7217=CARTESIAN_POINT ( 'NONE',  ( 139.7287565553230309, -1.999999999999978684, -25.16025403784439973 ) ) ;
#7218=ORIENTED_EDGE ( 'NONE', *, *, #4327, .F. ) ;
#7219=LINE ( 'NONE', #23542, #15381 ) ;
#7220=ORIENTED_EDGE ( 'NONE', *, *, #14443, .T. ) ;
#7226=DIRECTION ( 'NONE',  ( 0.000000000000000000, -0.000000000000000000, 1.000000000000000000 ) ) ;
#7229=CARTESIAN_POINT ( 'NONE',  ( 138.6922820468854525, -1.999999999999979572, -17.92658477444275533 ) ) ;
#7231=VERTEX_POINT ( 'NONE', #10596 ) ;
#7234=DIRECTION ( 'NONE',  ( -0.9510565162951536422, -2.566386769018988323E-16, 0.3090169943749475623 ) ) ;
#7236=DIRECTION ( 'NONE',  ( -0.8090169943749474513, -2.183098979609982436E-16, 0.5877852522924731371 ) ) ;
#7238=ADVANCED_FACE ( 'NONE', ( #26198 ), #3007, .T. ) ;
#7240=EDGE_CURVE ( 'NONE', #10075, #16811, #4186, .T. ) ;
#7244=EDGE_LOOP ( 'NONE', ( #6040, #6141, #1950, #14525, #22457 ) ) ;
#7245=VERTEX_POINT ( 'NONE', #1759 ) ;
#7246=CARTESIAN_POINT ( 'NONE',  ( 154.7287565553229456, -1.999999999999974909, -7.839745962155603820 ) ) ;
#7247=VECTOR ( 'NONE', #7923, 1000.000000000000000 ) ;
#7248=DIRECTION ( 'NONE',  ( 0.5877852522924731371, 0.000000000000000000, 0.8090169943749474513 ) ) ;
#7250=AXIS2_PLACEMENT_3D ( 'NONE', #28650, #1294, #5872 ) ;
#7251=CARTESIAN_POINT ( 'NONE',  ( 139.7287565553230309, -10.00000000000000533, -7.839745962155603820 ) ) ;
#7257=ADVANCED_FACE ( 'NONE', ( #27116 ), #25096, .T. ) ;
#7260=FACE_OUTER_BOUND ( 'NONE', #22754, .T. ) ;
#7261=LINE ( 'NONE', #16560, #6349 ) ;
#7263=DIRECTION ( 'NONE',  ( -2.698458740408365879E-16, 1.000000000000000000, 0.000000000000000000 ) ) ;
#7265=VERTEX_POINT ( 'NONE', #11048 ) ;
#7266=DIRECTION ( 'NONE',  ( -6.938893903907227392E-16, 0.000000000000000000, -1.000000000000000000 ) ) ;
#7267=FACE_OUTER_BOUND ( 'NONE', #14179, .T. ) ;
#7271=ORIENTED_EDGE ( 'NONE', *, *, #23516, .T. ) ;
#7273=AXIS2_PLACEMENT_3D ( 'NONE', #13315, #6458, #45 ) ;
#7276=VECTOR ( 'NONE', #19878, 1000.000000000000000 ) ;
#7279=EDGE_LOOP ( 'NONE', ( #23506, #14766, #26885, #7091 ) ) ;
#7281=CARTESIAN_POINT ( 'NONE',  ( 159.7287565553229456, -1.999999999999973133, -16.50000000000000355 ) ) ;
#7282=ORIENTED_EDGE ( 'NONE', *, *, #15931, .F. ) ;
#7283=CARTESIAN_POINT ( 'NONE',  ( 173.6922820468853388, -9.999999999999994671, -23.73366926340167637 ) ) ;
#7285=ADVANCED_FACE ( 'NONE', ( #4040 ), #17612, .T. ) ;
#7288=ADVANCED_FACE ( 'NONE', ( #22812 ), #2063, .T. ) ;
#7290=PLANE ( 'NONE',  #20997 ) ;
#7291=CARTESIAN_POINT ( 'NONE',  ( 114.0813507336719255, -4.999999999999986677, -82.88495296030824022 ) ) ;
#7293=CARTESIAN_POINT ( 'NONE',  ( 153.6922820468854241, -1.999999999999975353, -32.39392330124607611 ) ) ;
#7295=ORIENTED_EDGE ( 'NONE', *, *, #7370, .F. ) ;
#7297=ORIENTED_EDGE ( 'NONE', *, *, #6265, .T. ) ;
#7299=DIRECTION ( 'NONE',  ( 1.000000000000000000, 2.698458740408365879E-16, -1.110223024625156540E-16 ) ) ;
#7300=CARTESIAN_POINT ( 'NONE',  ( 175.7287565553229456, -4.999999999999970690, -4.785595155761523500 ) ) ;
#7301=EDGE_LOOP ( 'NONE', ( #10063, #5825, #25193, #17553, #18197, #8967 ) ) ;
#7307=DIRECTION ( 'NONE',  ( -0.5877852522924731371, -1.586114251531760235E-16, 0.8090169943749474513 ) ) ;
#7308=LINE ( 'NONE', #2737, #2067 ) ;
#7313=DIRECTION ( 'NONE',  ( -0.5877852522924731371, -1.586114251531760728E-16, -0.8090169943749474513 ) ) ;
#7314=DIRECTION ( 'NONE',  ( -2.698458740408366372E-16, 1.000000000000000000, 0.000000000000000000 ) ) ;
#7315=CARTESIAN_POINT ( 'NONE',  ( 175.7287565553229456, -4.999999999999970690, -10.89389676854971967 ) ) ;
#7316=LINE ( 'NONE', #1, #11716 ) ;
#7317=LINE ( 'NONE', #4719, #1670 ) ;
#7321=EDGE_CURVE ( 'NONE', #11139, #29174, #6482, .T. ) ;
#7322=FACE_OUTER_BOUND ( 'NONE', #5935, .T. ) ;
#7323=CARTESIAN_POINT ( 'NONE',  ( 167.0152310637604955, -1.999999999999970912, -26.04193191628311155 ) ) ;
#7324=ORIENTED_EDGE ( 'NONE', *, *, #5043, .T. ) ;
#7328=VERTEX_POINT ( 'NONE', #20059 ) ;
#7329=CARTESIAN_POINT ( 'NONE',  ( 177.2287565553228887, -9.999999999999994671, -20.83012701892220520 ) ) ;
#7330=ADVANCED_FACE ( 'NONE', ( #29271 ), #29433, .T. ) ;
#7333=FACE_BOUND ( 'NONE', #8697, .T. ) ;
#7335=AXIS2_PLACEMENT_3D ( 'NONE', #14968, #7963, #24016 ) ;
#7338=LINE ( 'NONE', #16637, #23297 ) ;
#7340=CARTESIAN_POINT ( 'NONE',  ( 138.6922820468854241, -1.999999999999979572, -15.07341522555727309 ) ) ;
#7341=VERTEX_POINT ( 'NONE', #8898 ) ;
#7342=PLANE ( 'NONE',  #4712 ) ;
#7343=ORIENTED_EDGE ( 'NONE', *, *, #27360, .T. ) ;
#7345=VERTEX_POINT ( 'NONE', #22514 ) ;
#7349=ORIENTED_EDGE ( 'NONE', *, *, #62, .F. ) ;
#7350=DIRECTION ( 'NONE',  ( 0.5877852522924731371, 0.000000000000000000, 0.8090169943749474513 ) ) ;
#7351=DIRECTION ( 'NONE',  ( -0.8090169943749474513, -2.183098979609982436E-16, 0.5877852522924731371 ) ) ;
#7352=AXIS2_PLACEMENT_3D ( 'NONE', #24691, #21628, #10472 ) ;
#7355=AXIS2_PLACEMENT_3D ( 'NONE', #29384, #26919, #5981 ) ;
#7358=VERTEX_POINT ( 'NONE', #18214 ) ;
#7359=FACE_BOUND ( 'NONE', #22663, .T. ) ;
#7360=AXIS2_PLACEMENT_3D ( 'NONE', #24100, #3203, #21805 ) ;
#7361=DIRECTION ( 'NONE',  ( -1.110223024625156540E-16, 0.000000000000000000, -1.000000000000000000 ) ) ;
#7363=DIRECTION ( 'NONE',  ( -2.698458740408365879E-16, 1.000000000000000000, 0.000000000000000000 ) ) ;
#7364=EDGE_CURVE ( 'NONE', #19492, #29780, #13040, .T. ) ;
#7367=EDGE_CURVE ( 'NONE', #18794, #27442, #20202, .T. ) ;
#7370=EDGE_CURVE ( 'NONE', #5507, #13972, #27427, .T. ) ;
#7373=CARTESIAN_POINT ( 'NONE',  ( 172.2287565553229740, -4.999999999999970690, -29.49038105676660138 ) ) ;
#7374=EDGE_LOOP ( 'NONE', ( #21615, #12842, #2058, #7766, #17510 ) ) ;
#7377=VERTEX_POINT ( 'NONE', #13924 ) ;
#7381=CARTESIAN_POINT ( 'NONE',  ( 171.1922820468853388, -4.999999999999971578, -22.25671179336496053 ) ) ;
#7383=VERTEX_POINT ( 'NONE', #25694 ) ;
#7384=CARTESIAN_POINT ( 'NONE',  ( 132.0152310637605808, -1.999999999999981348, -15.61832212156129351 ) ) ;
#7386=ORIENTED_EDGE ( 'NONE', *, *, #26607, .T. ) ;
#7389=FACE_OUTER_BOUND ( 'NONE', #25598, .T. ) ;
#7393=LINE ( 'NONE', #3125, #8128 ) ;
#7397=FACE_OUTER_BOUND ( 'NONE', #19366, .T. ) ;
#7398=ORIENTED_EDGE ( 'NONE', *, *, #26644, .F. ) ;
#7399=EDGE_CURVE ( 'NONE', #24599, #17207, #23256, .T. ) ;
#7400=LINE ( 'NONE', #16697, #8390 ) ;
#7401=VECTOR ( 'NONE', #16248, 1000.000000000000000 ) ;
#7402=CARTESIAN_POINT ( 'NONE',  ( 131.1922820468854241, -4.999999999999983125, -4.936203717676158398 ) ) ;
#7404=FACE_OUTER_BOUND ( 'NONE', #29379, .T. ) ;
#7405=EDGE_CURVE ( 'NONE', #7041, #13256, #368, .T. ) ;
#7406=DIRECTION ( 'NONE',  ( 0.9510565162951536422, 2.566386769018988816E-16, 0.3090169943749472292 ) ) ;
#7409=ADVANCED_FACE ( 'NONE', ( #11485 ), #23558, .T. ) ;
#7413=EDGE_LOOP ( 'NONE', ( #15394, #416, #26312, #21551, #27796 ) ) ;
#7415=LINE ( 'NONE', #5268, #12124 ) ;
#7416=LINE ( 'NONE', #16403, #17118 ) ;
#7419=EDGE_LOOP ( 'NONE', ( #23951, #20869, #23705, #11223, #18022 ) ) ;
#7420=CARTESIAN_POINT ( 'NONE',  ( 143.6922820468854241, -10.00000000000000355, -9.266330736598359152 ) ) ;
#7422=CARTESIAN_POINT ( 'NONE',  ( 139.5152310637605808, -1.999999999999978684, -13.05155085951651195 ) ) ;
#7423=DIRECTION ( 'NONE',  ( -0.9510565162951536422, -2.566386769018988816E-16, -0.3090169943749472292 ) ) ;
#7426=VERTEX_POINT ( 'NONE', #16071 ) ;
#7430=ORIENTED_EDGE ( 'NONE', *, *, #5489, .T. ) ;
#7432=ORIENTED_EDGE ( 'NONE', *, *, #16445, .F. ) ;
#7433=VECTOR ( 'NONE', #27364, 1000.000000000000000 ) ;
#7434=ORIENTED_EDGE ( 'NONE', *, *, #16179, .F. ) ;
#7436=LINE ( 'NONE', #14578, #5021 ) ;
#7437=DIRECTION ( 'NONE',  ( -0.9510565162951536422, 0.000000000000000000, -0.3090169943749472292 ) ) ;
#7438=CARTESIAN_POINT ( 'NONE',  ( 159.7287565553229172, -10.00000000000000000, -7.839745962155603820 ) ) ;
#7439=EDGE_CURVE ( 'NONE', #23755, #15731, #25399, .T. ) ;
#7440=CARTESIAN_POINT ( 'NONE',  ( 141.1922820468854241, -1.999999999999978684, -2.083034168790677043 ) ) ;
#7443=ORIENTED_EDGE ( 'NONE', *, *, #22242, .T. ) ;
#7444=DIRECTION ( 'NONE',  ( -0.5877852522924731371, 0.000000000000000000, 0.8090169943749474513 ) ) ;
#7445=DIRECTION ( 'NONE',  ( 0.3090169943749475623, 8.338696094058001131E-17, 0.9510565162951536422 ) ) ;
#7447=CARTESIAN_POINT ( 'NONE',  ( 116.0854136719178200, -4.999999999999985789, -84.34098991374325749 ) ) ;
#7448=DIRECTION ( 'NONE',  ( -0.9510565162951536422, -2.566386769018988323E-16, 0.3090169943749475623 ) ) ;
#7449=ORIENTED_EDGE ( 'NONE', *, *, #9684, .F. ) ;
#7452=VERTEX_POINT ( 'NONE', #2659 ) ;
#7454=PLANE ( 'NONE',  #19842 ) ;
#7455=ORIENTED_EDGE ( 'NONE', *, *, #24913, .T. ) ;
#7459=CARTESIAN_POINT ( 'NONE',  ( 24.19664217352669766, -5.000000000000010658, -74.46960727238361244 ) ) ;
#7460=CARTESIAN_POINT ( 'NONE',  ( 173.6922820468853672, -1.999999999999969358, -35.24709285013155835 ) ) ;
#7461=FACE_OUTER_BOUND ( 'NONE', #13404, .T. ) ;
#7462=ADVANCED_FACE ( 'NONE', ( #25857 ), #18079, .T. ) ;
#7463=CARTESIAN_POINT ( 'NONE',  ( 164.7287565553229172, -9.999999999999998224, -16.50000000000000355 ) ) ;
#7467=CARTESIAN_POINT ( 'NONE',  ( 163.6922820468853104, -4.999999999999973355, -6.413161187712876909 ) ) ;
#7469=VECTOR ( 'NONE', #6387, 1000.000000000000000 ) ;
#7471=CARTESIAN_POINT ( 'NONE',  ( 163.6922820468853672, -4.999999999999973355, -23.73366926340167637 ) ) ;
#7473=VERTEX_POINT ( 'NONE', #18974 ) ;
#7475=LINE ( 'NONE', #19359, #16364 ) ;
#7478=LINE ( 'NONE', #28276, #29795 ) ;
#7479=ORIENTED_EDGE ( 'NONE', *, *, #9275, .T. ) ;
#7481=CARTESIAN_POINT ( 'NONE',  ( 139.5152310637605808, -10.00000000000000533, -30.37205893520530964 ) ) ;
#7483=CARTESIAN_POINT ( 'NONE',  ( 137.0152310637605808, -10.00000000000000533, -17.38167787843870826 ) ) ;
#7486=VERTEX_POINT ( 'NONE', #23108 ) ;
#7488=ORIENTED_EDGE ( 'NONE', *, *, #22566, .T. ) ;
#7492=LINE ( 'NONE', #2932, #12549 ) ;
#7493=VECTOR ( 'NONE', #22528, 1000.000000000000000 ) ;
#7494=EDGE_LOOP ( 'NONE', ( #20241, #12259, #4263, #10973 ) ) ;
#7495=LINE ( 'NONE', #635, #23012 ) ;
#7497=EDGE_CURVE ( 'NONE', #16007, #18552, #18363, .T. ) ;
#7500=ADVANCED_FACE ( 'NONE', ( #28176 ), #4634, .T. ) ;
#7503=FACE_BOUND ( 'NONE', #25300, .T. ) ;
#7504=DIRECTION ( 'NONE',  ( -0.8090169943749474513, -2.183098979609982436E-16, 0.5877852522924731371 ) ) ;
#7505=CARTESIAN_POINT ( 'NONE',  ( 168.6922820468852819, -1.999999999999972244, -0.6060766987539614181 ) ) ;
#7507=CARTESIAN_POINT ( 'NONE',  ( 149.7287565553229740, -4.999999999999977796, -7.839745962155614478 ) ) ;
#7510=CARTESIAN_POINT ( 'NONE',  ( 132.0152310637605808, -10.00000000000000711, -15.61832212156129351 ) ) ;
#7512=EDGE_LOOP ( 'NONE', ( #26690, #21240, #11293, #26764, #8709 ) ) ;
#7516=FACE_OUTER_BOUND ( 'NONE', #19751, .T. ) ;
#7517=LINE ( 'NONE', #9488, #21794 ) ;
#7518=DIRECTION ( 'NONE',  ( -0.5877852522924731371, 0.000000000000000000, 0.8090169943749474513 ) ) ;
#7519=ORIENTED_EDGE ( 'NONE', *, *, #22279, .T. ) ;
#7525=DIRECTION ( 'NONE',  ( 0.3090169943749475623, 8.338696094058001131E-17, 0.9510565162951536422 ) ) ;
#7528=ORIENTED_EDGE ( 'NONE', *, *, #13557, .T. ) ;
#7529=DIRECTION ( 'NONE',  ( 0.000000000000000000, 0.000000000000000000, 1.000000000000000000 ) ) ;
#7531=EDGE_CURVE ( 'NONE', #6950, #23457, #5898, .T. ) ;
#7533=EDGE_CURVE ( 'NONE', #16634, #5625, #10453, .T. ) ;
#7535=EDGE_CURVE ( 'NONE', #19917, #27081, #19756, .T. ) ;
#7536=VECTOR ( 'NONE', #9551, 1000.000000000000000 ) ;
#7537=ORIENTED_EDGE ( 'NONE', *, *, #548, .T. ) ;
#7540=EDGE_LOOP ( 'NONE', ( #23721, #23587, #2764, #24605 ) ) ;
#7541=ORIENTED_EDGE ( 'NONE', *, *, #4465, .F. ) ;
#7543=CARTESIAN_POINT ( 'NONE',  ( 148.6922820468853956, -10.00000000000000178, -9.266330736598359152 ) ) ;
#7544=ORIENTED_EDGE ( 'NONE', *, *, #26020, .T. ) ;
#7547=DIRECTION ( 'NONE',  ( 0.9510565162951536422, 2.566386769018988816E-16, 0.3090169943749472292 ) ) ;
#7552=ORIENTED_EDGE ( 'NONE', *, *, #10343, .F. ) ;
#7554=PLANE ( 'NONE',  #29316 ) ;
#7557=LINE ( 'NONE', #3001, #27603 ) ;
#7559=ORIENTED_EDGE ( 'NONE', *, *, #14772, .F. ) ;
#7560=DIRECTION ( 'NONE',  ( -2.698458740408365879E-16, 1.000000000000000000, 0.000000000000000000 ) ) ;
#7566=ORIENTED_EDGE ( 'NONE', *, *, #9277, .F. ) ;
#7569=EDGE_CURVE ( 'NONE', #12418, #8151, #29282, .T. ) ;
#7571=EDGE_CURVE ( 'NONE', #17394, #11963, #17626, .T. ) ;
#7572=EDGE_CURVE ( 'NONE', #5536, #14016, #27438, .T. ) ;
#7576=EDGE_LOOP ( 'NONE', ( #26297, #12404, #9246, #17697 ) ) ;
#7577=DIRECTION ( 'NONE',  ( -0.5877852522924731371, 0.000000000000000000, 0.8090169943749474513 ) ) ;
#7579=CARTESIAN_POINT ( 'NONE',  ( 164.7287565553229172, -1.999999999999971800, -16.50000000000000355 ) ) ;
#7580=FACE_OUTER_BOUND ( 'NONE', #27334, .T. ) ;
#7581=VECTOR ( 'NONE', #9374, 1000.000000000000000 ) ;
#7584=VECTOR ( 'NONE', #1681, 1000.000000000000000 ) ;
#7585=PLANE ( 'NONE',  #27392 ) ;
#7586=CARTESIAN_POINT ( 'NONE',  ( 159.5152310637604387, -4.999999999999974243, -1.770974823053888411E-14 ) ) ;
#7590=ORIENTED_EDGE ( 'NONE', *, *, #15755, .F. ) ;
#7591=VECTOR ( 'NONE', #23857, 1000.000000000000000 ) ;
#7592=PLANE ( 'NONE',  #16355 ) ;
#7593=VECTOR ( 'NONE', #18842, 1000.000000000000000 ) ;
#7594=FACE_OUTER_BOUND ( 'NONE', #8691, .T. ) ;
#7595=ORIENTED_EDGE ( 'NONE', *, *, #2565, .F. ) ;
#7596=ORIENTED_EDGE ( 'NONE', *, *, #15085, .F. ) ;
#7599=EDGE_CURVE ( 'NONE', #27188, #13402, #29901, .T. ) ;
#7601=DIRECTION ( 'NONE',  ( -0.8090169943749474513, -2.183098979609982436E-16, 0.5877852522924731371 ) ) ;
#7602=CARTESIAN_POINT ( 'NONE',  ( 177.2287565553228319, -1.999999999999969358, -3.509618943233403510 ) ) ;
#7603=EDGE_CURVE ( 'NONE', #24131, #11059, #16237, .T. ) ;
#7605=EDGE_CURVE ( 'NONE', #27678, #14364, #8762, .T. ) ;
#7606=VECTOR ( 'NONE', #9226, 1000.000000000000000 ) ;
#7607=CARTESIAN_POINT ( 'NONE',  ( 174.5152310637603819, -4.999999999999970690, -4.391296821672111328 ) ) ;
#7608=CARTESIAN_POINT ( 'NONE',  ( 141.1922820468854525, -4.999999999999979572, -19.40354224447947473 ) ) ;
#7610=VECTOR ( 'NONE', #12878, 1000.000000000000000 ) ;
#7611=PLANE ( 'NONE',  #23433 ) ;
#7612=VECTOR ( 'NONE', #26956, 999.9999999999998863 ) ;
#7613=CARTESIAN_POINT ( 'NONE',  ( 175.7287565553229456, -4.999999999999970690, -10.89389676854972322 ) ) ;
#7617=ORIENTED_EDGE ( 'NONE', *, *, #14091, .T. ) ;
#7619=DIRECTION ( 'NONE',  ( 1.000000000000000000, 2.698458740408365879E-16, -1.110223024625156540E-16 ) ) ;
#7623=EDGE_CURVE ( 'NONE', #26798, #6983, #9052, .T. ) ;
#7624=ORIENTED_EDGE ( 'NONE', *, *, #14855, .T. ) ;
#7627=CIRCLE ( 'NONE', #21771, 8.000000000000007105 ) ;
#7629=DIRECTION ( 'NONE',  ( -0.5877852522924731371, -1.586114251531760728E-16, -0.8090169943749474513 ) ) ;
#7630=ORIENTED_EDGE ( 'NONE', *, *, #18418, .T. ) ;
#7631=CARTESIAN_POINT ( 'NONE',  ( 138.6922820468854241, -1.999999999999980016, -0.6060766987539614181 ) ) ;
#7632=EDGE_LOOP ( 'NONE', ( #28419, #17135, #19042, #10992, #21715 ) ) ;
#7634=ORIENTED_EDGE ( 'NONE', *, *, #3607, .F. ) ;
#7639=EDGE_LOOP ( 'NONE', ( #4819, #20533, #8842, #11972 ) ) ;
#7640=AXIS2_PLACEMENT_3D ( 'NONE', #9790, #13910, #26143 ) ;
#7641=DIRECTION ( 'NONE',  ( -0.8090169943749474513, -2.183098979609982436E-16, 0.5877852522924731371 ) ) ;
#7642=EDGE_LOOP ( 'NONE', ( #19937, #26511, #5293, #15205, #27545 ) ) ;
#7643=VERTEX_POINT ( 'NONE', #8910 ) ;
#7644=ADVANCED_FACE ( 'NONE', ( #11649 ), #18227, .T. ) ;
#7648=VECTOR ( 'NONE', #14695, 1000.000000000000000 ) ;
#7652=FACE_BOUND ( 'NONE', #15216, .T. ) ;
#7653=VECTOR ( 'NONE', #20342, 1000.000000000000000 ) ;
#7654=CARTESIAN_POINT ( 'NONE',  ( 168.6922820468853104, -1.999999999999971800, -6.413161187712876909 ) ) ;
#7656=CARTESIAN_POINT ( 'NONE',  ( 158.6922820468853672, -4.999999999999975131, -15.07341522555727664 ) ) ;
#7657=AXIS2_PLACEMENT_3D ( 'NONE', #27201, #24881, #18140 ) ;
#7658=FACE_OUTER_BOUND ( 'NONE', #20832, .T. ) ;
#7660=DIRECTION ( 'NONE',  ( -0.5877852522924731371, -1.586114251531760728E-16, -0.8090169943749474513 ) ) ;
#7661=ADVANCED_FACE ( 'NONE', ( #29753 ), #18078, .T. ) ;
#7665=EDGE_CURVE ( 'NONE', #29884, #8986, #1926, .T. ) ;
#7667=PLANE ( 'NONE',  #2510 ) ;
#7669=CARTESIAN_POINT ( 'NONE',  ( 162.2287565553229740, -4.999999999999973355, -29.49038105676660138 ) ) ;
#7670=ORIENTED_EDGE ( 'NONE', *, *, #30124, .F. ) ;
#7671=CARTESIAN_POINT ( 'NONE',  ( 177.2287565553228603, -9.999999999999994671, -12.16987298107780369 ) ) ;
#7676=ORIENTED_EDGE ( 'NONE', *, *, #17141, .T. ) ;
#7677=AXIS2_PLACEMENT_3D ( 'NONE', #4595, #13883, #21519 ) ;
#7678=DIRECTION ( 'NONE',  ( 0.3090169943749472292, 8.338696094057992503E-17, -0.9510565162951536422 ) ) ;
#7680=ORIENTED_EDGE ( 'NONE', *, *, #2177, .T. ) ;
#7681=CARTESIAN_POINT ( 'NONE',  ( 131.1922820468854241, -10.00000000000000888, -30.91696583120935671 ) ) ;
#7685=LINE ( 'NONE', #19275, #29935 ) ;
#7688=AXIS2_PLACEMENT_3D ( 'NONE', #25829, #4912, #14208 ) ;
#7689=CARTESIAN_POINT ( 'NONE',  ( 131.1922820468854241, -10.00000000000000888, -2.083034168790677043 ) ) ;
#7691=CARTESIAN_POINT ( 'NONE',  ( 176.1922820468853104, -9.999999999999994671, -19.40354224447947828 ) ) ;
#7692=LINE ( 'NONE', #17004, #24617 ) ;
#7693=VECTOR ( 'NONE', #18054, 1000.000000000000000 ) ;
#7697=EDGE_CURVE ( 'NONE', #11977, #23167, #27581, .T. ) ;
#7699=ORIENTED_EDGE ( 'NONE', *, *, #3171, .F. ) ;
#7701=AXIS2_PLACEMENT_3D ( 'NONE', #3704, #17577, #26934 ) ;
#7702=CARTESIAN_POINT ( 'NONE',  ( 156.1922820468854241, -10.00000000000000000, -28.06379628232387802 ) ) ;
#7703=LINE ( 'NONE', #1282, #22372 ) ;
#7704=DIRECTION ( 'NONE',  ( -2.698458740408366372E-16, 1.000000000000000000, 0.000000000000000000 ) ) ;
#7705=EDGE_CURVE ( 'NONE', #5343, #15277, #18376, .T. ) ;
#7706=FACE_OUTER_BOUND ( 'NONE', #18007, .T. ) ;
#7707=CARTESIAN_POINT ( 'NONE',  ( 175.7287565553229456, -4.999999999999969802, -19.55415080639413006 ) ) ;
#7710=ORIENTED_EDGE ( 'NONE', *, *, #10100, .F. ) ;
#7713=FACE_OUTER_BOUND ( 'NONE', #29899, .T. ) ;
#7721=VECTOR ( 'NONE', #12368, 1000.000000000000000 ) ;
#7722=ORIENTED_EDGE ( 'NONE', *, *, #411, .F. ) ;
#7723=CARTESIAN_POINT ( 'NONE',  ( 137.2287565553230309, -1.999999999999979572, -12.16987298107780013 ) ) ;
#7724=AXIS2_PLACEMENT_3D ( 'NONE', #20880, #2736, #25827 ) ;
#7725=EDGE_CURVE ( 'NONE', #19562, #2080, #25262, .T. ) ;
#7726=VECTOR ( 'NONE', #28716, 1000.000000000000000 ) ;
#7727=DIRECTION ( 'NONE',  ( -2.698458740408365879E-16, 1.000000000000000000, 0.000000000000000000 ) ) ;
#7728=CARTESIAN_POINT ( 'NONE',  ( 144.5152310637606092, -1.999999999999977129, -19.94844914048349693 ) ) ;
#7729=LINE ( 'NONE', #22075, #4592 ) ;
#7730=DIRECTION ( 'NONE',  ( -0.5877852522924731371, -1.586114251531760728E-16, -0.8090169943749474513 ) ) ;
#7735=CARTESIAN_POINT ( 'NONE',  ( 162.2287565553229740, -9.999999999999998224, -29.49038105676660493 ) ) ;
#7736=EDGE_CURVE ( 'NONE', #3555, #23467, #11211, .T. ) ;
#7739=PLANE ( 'NONE',  #16078 ) ;
#7740=ADVANCED_FACE ( 'NONE', ( #1774 ), #11060, .T. ) ;
#7741=DIRECTION ( 'NONE',  ( 0.9510565162951536422, 0.000000000000000000, -0.3090169943749475623 ) ) ;
#7742=ORIENTED_EDGE ( 'NONE', *, *, #26602, .T. ) ;
#7743=VECTOR ( 'NONE', #2989, 1000.000000000000000 ) ;
#7744=CARTESIAN_POINT ( 'NONE',  ( 130.7287565553229456, -10.00000000000000888, -10.89389676854976408 ) ) ;
#7745=DIRECTION ( 'NONE',  ( 1.110223024625156540E-16, 2.995891024602366092E-32, 1.000000000000000000 ) ) ;
#7746=DIRECTION ( 'NONE',  ( -2.698458740408365879E-16, 1.000000000000000000, 0.000000000000000000 ) ) ;
#7747=ORIENTED_EDGE ( 'NONE', *, *, #14093, .F. ) ;
#7748=VECTOR ( 'NONE', #23901, 1000.000000000000000 ) ;
#7751=VERTEX_POINT ( 'NONE', #26321 ) ;
#7754=CARTESIAN_POINT ( 'NONE',  ( 144.7287565553230309, -10.00000000000000355, -33.82050807568879947 ) ) ;
#7755=DIRECTION ( 'NONE',  ( 0.5877852522924731371, 1.586114251531760728E-16, -0.8090169943749474513 ) ) ;
#7756=CARTESIAN_POINT ( 'NONE',  ( 142.0152310637605524, -10.00000000000000533, 1.702185954127501066 ) ) ;
#7757=LINE ( 'NONE', #19647, #16731 ) ;
#7758=CARTESIAN_POINT ( 'NONE',  ( 164.7287565553228887, -1.999999999999972689, 0.8205080756887930260 ) ) ;
#7760=DIRECTION ( 'NONE',  ( -2.698458740408365879E-16, 1.000000000000000000, 0.000000000000000000 ) ) ;
#7762=CARTESIAN_POINT ( 'NONE',  ( 174.7287565553228603, -4.999999999999970690, -7.839745962155600267 ) ) ;
#7766=ORIENTED_EDGE ( 'NONE', *, *, #29045, .T. ) ;
#7768=EDGE_CURVE ( 'NONE', #19382, #18123, #9820, .T. ) ;
#7774=EDGE_CURVE ( 'NONE', #27148, #28906, #3132, .T. ) ;
#7775=ORIENTED_EDGE ( 'NONE', *, *, #27930, .F. ) ;
#7777=LINE ( 'NONE', #17088, #7247 ) ;
#7779=CARTESIAN_POINT ( 'NONE',  ( 174.7287565553229456, -4.999999999999969802, -25.16025403784439973 ) ) ;
#7780=ORIENTED_EDGE ( 'NONE', *, *, #14816, .F. ) ;
#7781=DIRECTION ( 'NONE',  ( -2.698458740408365879E-16, 1.000000000000000000, 0.000000000000000000 ) ) ;
#7782=ORIENTED_EDGE ( 'NONE', *, *, #24701, .T. ) ;
#7783=( GEOMETRIC_REPRESENTATION_CONTEXT ( 3 ) GLOBAL_UNCERTAINTY_ASSIGNED_CONTEXT ( ( #11622 ) ) GLOBAL_UNIT_ASSIGNED_CONTEXT ( ( #29747, #27726, #4342 ) ) REPRESENTATION_CONTEXT ( 'NONE', 'WORKASPACE' ) );
#7785=EDGE_LOOP ( 'NONE', ( #30150, #6671, #14835, #7282 ) ) ;
#7786=VECTOR ( 'NONE', #10957, 1000.000000000000000 ) ;
#7790=VERTEX_POINT ( 'NONE', #5249 ) ;
#7793=AXIS2_PLACEMENT_3D ( 'NONE', #15564, #21995, #8244 ) ;
#7794=AXIS2_PLACEMENT_3D ( 'NONE', #16881, #24219, #3605 ) ;
#7797=VERTEX_POINT ( 'NONE', #380 ) ;
#7800=ORIENTED_EDGE ( 'NONE', *, *, #16308, .T. ) ;
#7801=LINE ( 'NONE', #5518, #15405 ) ;
#7802=EDGE_CURVE ( 'NONE', #23532, #11745, #23416, .T. ) ;
#7804=CARTESIAN_POINT ( 'NONE',  ( 15.04976660853063741, -5.000000000000013323, -46.31841892940461491 ) ) ;
#7805=DIRECTION ( 'NONE',  ( 0.9510565162951535312, 2.566386769018988816E-16, -0.3090169943749475623 ) ) ;
#7806=CIRCLE ( 'NONE', #7335, 5.999999999999977796 ) ;
#7807=CARTESIAN_POINT ( 'NONE',  ( 172.0152310637604955, -1.999999999999969580, -24.27857615940569502 ) ) ;
#7812=LINE ( 'NONE', #19396, #28035 ) ;
#7814=ORIENTED_EDGE ( 'NONE', *, *, #23522, .T. ) ;
#7817=DIRECTION ( 'NONE',  ( -1.110223024625156540E-16, 0.000000000000000000, -1.000000000000000000 ) ) ;
#7819=DIRECTION ( 'NONE',  ( -0.9510565162951536422, -2.566386769018988816E-16, -0.3090169943749472292 ) ) ;
#7821=CARTESIAN_POINT ( 'NONE',  ( 137.0152310637606092, -10.00000000000000533, -6.958068083716895558 ) ) ;
#7824=VECTOR ( 'NONE', #8787, 1000.000000000000000 ) ;
#7825=ORIENTED_EDGE ( 'NONE', *, *, #10213, .F. ) ;
#7828=ORIENTED_EDGE ( 'NONE', *, *, #19070, .T. ) ;
#7829=CARTESIAN_POINT ( 'NONE',  ( 147.2287565553230024, -10.00000000000000355, -12.16987298107780369 ) ) ;
#7831=EDGE_LOOP ( 'NONE', ( #20505, #12348, #11044, #24446 ) ) ;
#7835=CARTESIAN_POINT ( 'NONE',  ( 147.0152310637605524, -1.999999999999977129, -6.958068083716895558 ) ) ;
#7836=ORIENTED_EDGE ( 'NONE', *, *, #4864, .T. ) ;
#7837=EDGE_CURVE ( 'NONE', #13174, #1647, #19279, .T. ) ;
#7838=CARTESIAN_POINT ( 'NONE',  ( 159.5152310637604671, -1.999999999999974021, -2.627941064794695691 ) ) ;
#7840=CARTESIAN_POINT ( 'NONE',  ( 94.69354921296734062, -4.999999999999992006, 68.79889063098933377 ) ) ;
#7841=FACE_OUTER_BOUND ( 'NONE', #19911, .T. ) ;
#7842=CARTESIAN_POINT ( 'NONE',  ( 131.1922820468854241, -10.00000000000000888, -13.59645775552055547 ) ) ;
#7843=VECTOR ( 'NONE', #27676, 1000.000000000000114 ) ;
#7844=DIRECTION ( 'NONE',  ( -0.8090169943749474513, -2.183098979609982436E-16, 0.5877852522924731371 ) ) ;
#7849=ORIENTED_EDGE ( 'NONE', *, *, #10581, .T. ) ;
#7851=FACE_OUTER_BOUND ( 'NONE', #8377, .T. ) ;
#7855=CARTESIAN_POINT ( 'NONE',  ( 173.6922820468853672, -1.999999999999969358, -35.24709285013155835 ) ) ;
#7857=EDGE_LOOP ( 'NONE', ( #9513, #21111, #18313, #5976 ) ) ;
#7858=DIRECTION ( 'NONE',  ( 6.938893903907227392E-16, -0.000000000000000000, 1.000000000000000000 ) ) ;
#7861=DIRECTION ( 'NONE',  ( -2.698458740408365879E-16, 1.000000000000000000, 0.000000000000000000 ) ) ;
#7864=ORIENTED_EDGE ( 'NONE', *, *, #22670, .T. ) ;
#7866=VECTOR ( 'NONE', #16716, 1000.000000000000000 ) ;
#7868=AXIS2_PLACEMENT_3D ( 'NONE', #14112, #2556, #28216 ) ;
#7870=EDGE_LOOP ( 'NONE', ( #20717, #19940, #386, #30 ) ) ;
#7871=EDGE_CURVE ( 'NONE', #29710, #11366, #28490, .T. ) ;
#7872=EDGE_CURVE ( 'NONE', #10756, #11518, #21267, .T. ) ;
#7874=EDGE_CURVE ( 'NONE', #20344, #21061, #26172, .T. ) ;
#7876=EDGE_CURVE ( 'NONE', #29420, #11271, #21427, .T. ) ;
#7877=LINE ( 'NONE', #21766, #25996 ) ;
#7878=EDGE_LOOP ( 'NONE', ( #10834, #9568, #19147, #28544 ) ) ;
#7879=ORIENTED_EDGE ( 'NONE', *, *, #22493, .F. ) ;
#7880=CARTESIAN_POINT ( 'NONE',  ( 90.15252717933853432, -4.999999999999992895, 65.49964500294863967 ) ) ;
#7881=CARTESIAN_POINT ( 'NONE',  ( 156.1922820468853672, -10.00000000000000000, -13.59645775552055902 ) ) ;
#7882=CARTESIAN_POINT ( 'NONE',  ( 174.7287565553229172, -9.999999999999994671, -25.16025403784440329 ) ) ;
#7883=LINE ( 'NONE', #1032, #14116 ) ;
#7886=LINE ( 'NONE', #28991, #28853 ) ;
#7887=DIRECTION ( 'NONE',  ( 0.5877852522924731371, 1.586114251531760728E-16, -0.8090169943749474513 ) ) ;
#7889=DIRECTION ( 'NONE',  ( 0.000000000000000000, 0.000000000000000000, -1.000000000000000000 ) ) ;
#7891=ORIENTED_EDGE ( 'NONE', *, *, #20653, .T. ) ;
#7892=CARTESIAN_POINT ( 'NONE',  ( 173.6922820468853672, -9.999999999999994671, -35.24709285013155835 ) ) ;
#7893=CARTESIAN_POINT ( 'NONE',  ( 139.5152310637605808, -4.999999999999980460, -2.627941064794695691 ) ) ;
#7895=FACE_OUTER_BOUND ( 'NONE', #18960, .T. ) ;
#7897=ORIENTED_EDGE ( 'NONE', *, *, #7871, .F. ) ;
#7898=ORIENTED_EDGE ( 'NONE', *, *, #22074, .F. ) ;
#7902=CARTESIAN_POINT ( 'NONE',  ( 152.0152310637604671, -10.00000000000000178, -17.38167787843870826 ) ) ;
#7903=LINE ( 'NONE', #5622, #23818 ) ;
#7904=DIRECTION ( 'NONE',  ( 0.9510565162951535312, 2.566386769018988816E-16, -0.3090169943749475623 ) ) ;
#7906=ORIENTED_EDGE ( 'NONE', *, *, #27177, .F. ) ;
#7908=LINE ( 'NONE', #14462, #10833 ) ;
#7909=CARTESIAN_POINT ( 'NONE',  ( 139.7287565553230309, -10.00000000000000533, -25.16025403784439973 ) ) ;
#7911=VECTOR ( 'NONE', #16309, 1000.000000000000000 ) ;
#7912=LINE ( 'NONE', #22254, #11224 ) ;
#7916=EDGE_LOOP ( 'NONE', ( #6326, #406, #13974, #29488, #22260, #3696 ) ) ;
#7921=FACE_BOUND ( 'NONE', #13384, .T. ) ;
#7922=ORIENTED_EDGE ( 'NONE', *, *, #24814, .F. ) ;
#7923=DIRECTION ( 'NONE',  ( -2.698458740408365879E-16, 1.000000000000000000, 0.000000000000000000 ) ) ;
#7925=DIRECTION ( 'NONE',  ( 1.000000000000000000, 2.698458740408365879E-16, -1.110223024625156540E-16 ) ) ;
#7926=ORIENTED_EDGE ( 'NONE', *, *, #22453, .F. ) ;
#7927=CARTESIAN_POINT ( 'NONE',  ( 171.1922820468853104, -9.999999999999996447, -10.74328820663507678 ) ) ;
#7928=ORIENTED_EDGE ( 'NONE', *, *, #15442, .T. ) ;
#7930=VERTEX_POINT ( 'NONE', #14693 ) ;
#7934=LINE ( 'NONE', #29041, #16981 ) ;
#7940=ADVANCED_FACE ( 'NONE', ( #24034 ), #21717, .T. ) ;
#7941=EDGE_CURVE ( 'NONE', #12834, #2206, #28795, .T. ) ;
#7945=EDGE_CURVE ( 'NONE', #24305, #6528, #25867, .T. ) ;
#7946=FACE_BOUND ( 'NONE', #11596, .T. ) ;
#7948=DIRECTION ( 'NONE',  ( 1.000000000000000000, 2.698458740408365879E-16, -1.110223024625156540E-16 ) ) ;
#7949=CARTESIAN_POINT ( 'NONE',  ( 17.43705417884378051, -5.000000000000013323, -53.66573458306050526 ) ) ;
#7951=DIRECTION ( 'NONE',  ( 0.5877852522924731371, 0.000000000000000000, 0.8090169943749474513 ) ) ;
#7953=PLANE ( 'NONE',  #9903 ) ;
#7955=ORIENTED_EDGE ( 'NONE', *, *, #16701, .F. ) ;
#7957=ORIENTED_EDGE ( 'NONE', *, *, #14402, .F. ) ;
#7961=CARTESIAN_POINT ( 'NONE',  ( 171.1922820468853104, -9.999999999999996447, -10.74328820663507678 ) ) ;
#7963=DIRECTION ( 'NONE',  ( -2.698458740408365879E-16, 1.000000000000000000, 0.000000000000000000 ) ) ;
#7965=ORIENTED_EDGE ( 'NONE', *, *, #4771, .T. ) ;
#7967=ORIENTED_EDGE ( 'NONE', *, *, #6013, .T. ) ;
#7974=PLANE ( 'NONE',  #1911 ) ;
#7975=DIRECTION ( 'NONE',  ( -0.5877852522924731371, -1.586114251531760728E-16, -0.8090169943749474513 ) ) ;
#7976=VECTOR ( 'NONE', #28685, 1000.000000000000000 ) ;
#7980=EDGE_CURVE ( 'NONE', #8557, #6680, #7400, .T. ) ;
#7981=ADVANCED_FACE ( 'NONE', ( #23725 ), #2827, .T. ) ;
#7982=VERTEX_POINT ( 'NONE', #14987 ) ;
#7983=CARTESIAN_POINT ( 'NONE',  ( 176.1922820468852819, -9.999999999999994671, -10.74328820663507678 ) ) ;
#7985=CARTESIAN_POINT ( 'NONE',  ( 169.5152310637604671, -9.999999999999996447, -21.71180489736091346 ) ) ;
#7986=DIRECTION ( 'NONE',  ( -0.7071067811865480168, 0.7071067811865470176, 0.000000000000000000 ) ) ;
#7987=DIRECTION ( 'NONE',  ( -0.9510565162951536422, 0.000000000000000000, -0.3090169943749472292 ) ) ;
#7992=EDGE_LOOP ( 'NONE', ( #13638, #4628, #7595, #24514 ) ) ;
#7993=CARTESIAN_POINT ( 'NONE',  ( 161.1922820468853388, -1.999999999999973577, -13.59645775552055902 ) ) ;
#7995=LINE ( 'NONE', #17014, #16526 ) ;
#7997=DIRECTION ( 'NONE',  ( 1.110223024625156540E-16, 2.995891024602366092E-32, 1.000000000000000000 ) ) ;
#7998=CARTESIAN_POINT ( 'NONE',  ( 137.0152310637605524, -4.999999999999980460, -0.06116980274991495881 ) ) ;
#8001=ORIENTED_EDGE ( 'NONE', *, *, #21041, .F. ) ;
#8002=CARTESIAN_POINT ( 'NONE',  ( 154.5152310637605240, -4.999999999999976019, -1.715463671822631530E-14 ) ) ;
#8004=EDGE_CURVE ( 'NONE', #22761, #2119, #15287, .T. ) ;
#8005=PLANE ( 'NONE',  #29615 ) ;
#8006=LINE ( 'NONE', #24202, #10787 ) ;
#8008=VECTOR ( 'NONE', #1935, 1000.000000000000000 ) ;
#8011=VERTEX_POINT ( 'NONE', #10571 ) ;
#8012=DIRECTION ( 'NONE',  ( -0.5877852522924731371, -1.586114251531760235E-16, 0.8090169943749474513 ) ) ;
#8016=EDGE_LOOP ( 'NONE', ( #15611, #15860, #6685, #17348, #3836, #17449, #8403, #22392, #11122, #8252, #1086, #21290, #25803, #22005, #9192, #808, #10050, #4346, #15757, #122, #1197, #28020, #6374, #13520, #7965, #13013, #18906, #22555, #18244, #14896, #15842, #7680, #29090, #28010, #1167, #544, #19403, #18129, #27669, #13287, #298, #21755, #16921, #21063 ) ) ;
#8018=DIRECTION ( 'NONE',  ( 0.9510565162951536422, 0.000000000000000000, -0.3090169943749475623 ) ) ;
#8021=CARTESIAN_POINT ( 'NONE',  ( 142.0152310637606092, -10.00000000000000355, -15.61832212156129707 ) ) ;
#8024=LINE ( 'NONE', #8174, #2452 ) ;
#8028=DIRECTION ( 'NONE',  ( 0.3090169943749475623, 8.338696094058001131E-17, 0.9510565162951536422 ) ) ;
#8030=CARTESIAN_POINT ( 'NONE',  ( 167.0152310637604387, -9.999999999999998224, -8.721423840594312082 ) ) ;
#8031=ORIENTED_EDGE ( 'NONE', *, *, #7599, .T. ) ;
#8032=DIRECTION ( 'NONE',  ( 0.9510565162951536422, 2.566386769018988816E-16, 0.3090169943749472292 ) ) ;
#8033=ADVANCED_FACE ( 'NONE', ( #6001 ), #24621, .T. ) ;
#8035=VERTEX_POINT ( 'NONE', #10721 ) ;
#8036=CARTESIAN_POINT ( 'NONE',  ( 144.5152310637606092, -4.999999999999978684, -19.94844914048349693 ) ) ;
#8038=EDGE_CURVE ( 'NONE', #29180, #10203, #13014, .T. ) ;
#8039=DIRECTION ( 'NONE',  ( -0.9510565162951536422, -2.566386769018988816E-16, -0.3090169943749472292 ) ) ;
#8041=VERTEX_POINT ( 'NONE', #21873 ) ;
#8045=CARTESIAN_POINT ( 'NONE',  ( 137.2287565553230309, -1.999999999999979572, -20.83012701892220164 ) ) ;
#8046=DIRECTION ( 'NONE',  ( 0.9510565162951535312, 2.566386769018988816E-16, -0.3090169943749475623 ) ) ;
#8047=AXIS2_PLACEMENT_3D ( 'NONE', #3988, #3838, #13130 ) ;
#8048=CARTESIAN_POINT ( 'NONE',  ( 174.7287565553228319, -9.999999999999996447, 0.8205080756887930260 ) ) ;
#8049=ORIENTED_EDGE ( 'NONE', *, *, #20921, .F. ) ;
#8050=ORIENTED_EDGE ( 'NONE', *, *, #4948, .T. ) ;
#8051=DIRECTION ( 'NONE',  ( -2.698458740408365879E-16, 1.000000000000000000, 0.000000000000000000 ) ) ;
#8052=LINE ( 'NONE', #22101, #17976 ) ;
#8056=ORIENTED_EDGE ( 'NONE', *, *, #18721, .F. ) ;
#8058=EDGE_LOOP ( 'NONE', ( #16856, #11635, #22345, #5630 ) ) ;
#8059=VECTOR ( 'NONE', #3686, 1000.000000000000000 ) ;
#8061=VECTOR ( 'NONE', #14100, 1000.000000000000000 ) ;
#8064=FACE_BOUND ( 'NONE', #15416, .T. ) ;
#8065=EDGE_CURVE ( 'NONE', #30101, #11857, #5855, .T. ) ;
#8066=ORIENTED_EDGE ( 'NONE', *, *, #23169, .F. ) ;
#8067=FACE_OUTER_BOUND ( 'NONE', #14591, .T. ) ;
#8070=CARTESIAN_POINT ( 'NONE',  ( 152.0152310637605808, -4.999999999999976019, -24.27857615940569502 ) ) ;
#8071=EDGE_CURVE ( 'NONE', #26570, #29971, #29242, .T. ) ;
#8072=ORIENTED_EDGE ( 'NONE', *, *, #7802, .F. ) ;
#8073=CARTESIAN_POINT ( 'NONE',  ( 169.5152310637605240, -1.999999999999970024, -28.60870317832789667 ) ) ;
#8074=VERTEX_POINT ( 'NONE', #17731 ) ;
#8077=ORIENTED_EDGE ( 'NONE', *, *, #6372, .T. ) ;
#8080=VECTOR ( 'NONE', #19332, 1000.000000000000000 ) ;
#8081=CARTESIAN_POINT ( 'NONE',  ( 98.03139517864238428, -4.999999999999991118, -71.22397767698338100 ) ) ;
#8085=VECTOR ( 'NONE', #6512, 1000.000000000000000 ) ;
#8087=CARTESIAN_POINT ( 'NONE',  ( 146.1922820468853956, -4.999999999999978684, -4.936203717676158398 ) ) ;
#8088=FACE_BOUND ( 'NONE', #22615, .T. ) ;
#8091=FACE_OUTER_BOUND ( 'NONE', #764, .T. ) ;
#8092=CARTESIAN_POINT ( 'NONE',  ( 173.6922820468853672, -4.999999999999969802, -32.39392330124607611 ) ) ;
#8095=AXIS2_PLACEMENT_3D ( 'NONE', #28513, #14111, #23443 ) ;
#8097=LINE ( 'NONE', #15112, #1694 ) ;
#8099=CARTESIAN_POINT ( 'NONE',  ( 159.5152310637604671, -10.00000000000000000, -2.627941064794695691 ) ) ;
#8100=EDGE_LOOP ( 'NONE', ( #10433, #9885, #5203, #23276 ) ) ;
#8104=EDGE_CURVE ( 'NONE', #17985, #22052, #27091, .T. ) ;
#8105=VECTOR ( 'NONE', #3881, 1000.000000000000000 ) ;
#8109=ADVANCED_FACE ( 'NONE', ( #12708 ), #26783, .T. ) ;
#8111=EDGE_LOOP ( 'NONE', ( #9253, #20031, #28862, #22428 ) ) ;
#8112=CARTESIAN_POINT ( 'NONE',  ( 138.6922820468854525, -10.00000000000000533, -6.413161187712876909 ) ) ;
#8114=ORIENTED_EDGE ( 'NONE', *, *, #24105, .F. ) ;
#8119=EDGE_LOOP ( 'NONE', ( #16741, #18322, #16776, #6025 ) ) ;
#8121=CARTESIAN_POINT ( 'NONE',  ( 139.7287565553230309, -1.999999999999978684, -16.50000000000000000 ) ) ;
#8123=FACE_OUTER_BOUND ( 'NONE', #16841, .T. ) ;
#8124=CARTESIAN_POINT ( 'NONE',  ( 163.6922820468853388, -9.999999999999998224, -15.07341522555727664 ) ) ;
#8128=VECTOR ( 'NONE', #4939, 1000.000000000000000 ) ;
#8129=VERTEX_POINT ( 'NONE', #10867 ) ;
#8131=VECTOR ( 'NONE', #17860, 1000.000000000000000 ) ;
#8132=CARTESIAN_POINT ( 'NONE',  ( 148.6922820468854241, -1.999999999999977129, -23.73366926340167637 ) ) ;
#8133=AXIS2_PLACEMENT_3D ( 'NONE', #5456, #14143, #5149 ) ;
#8135=CARTESIAN_POINT ( 'NONE',  ( 136.1922820468854241, -1.999999999999980016, -10.74328820663507322 ) ) ;
#8141=VERTEX_POINT ( 'NONE', #17589 ) ;
#8143=FACE_OUTER_BOUND ( 'NONE', #19526, .T. ) ;
#8144=DIRECTION ( 'NONE',  ( -2.698458740408365879E-16, 1.000000000000000000, 0.000000000000000000 ) ) ;
#8145=LINE ( 'NONE', #3583, #23924 ) ;
#8146=ADVANCED_FACE ( 'NONE', ( #29557 ), #29410, .T. ) ;
#8149=EDGE_CURVE ( 'NONE', #26798, #27886, #19579, .T. ) ;
#8151=VERTEX_POINT ( 'NONE', #15599 ) ;
#8152=CARTESIAN_POINT ( 'NONE',  ( 129.5152310637605524, -10.00000000000000888, -13.05155085951650840 ) ) ;
#8153=EDGE_CURVE ( 'NONE', #29449, #13920, #22941, .T. ) ;
#8155=VECTOR ( 'NONE', #24611, 1000.000000000000000 ) ;
#8156=DIRECTION ( 'NONE',  ( 1.000000000000000000, 2.698458740408365879E-16, -1.110223024625156540E-16 ) ) ;
#8157=CARTESIAN_POINT ( 'NONE',  ( 144.5152310637606092, -10.00000000000000178, -19.94844914048349693 ) ) ;
#8159=CARTESIAN_POINT ( 'NONE',  ( 166.1922820468853672, -1.999999999999971356, -30.91696583120936026 ) ) ;
#8166=VECTOR ( 'NONE', #12807, 1000.000000000000000 ) ;
#8168=EDGE_CURVE ( 'NONE', #12771, #18151, #4012, .T. ) ;
#8169=ORIENTED_EDGE ( 'NONE', *, *, #11209, .F. ) ;
#8170=VECTOR ( 'NONE', #19417, 1000.000000000000000 ) ;
#8172=DIRECTION ( 'NONE',  ( -2.698458740408365879E-16, 1.000000000000000000, 0.000000000000000000 ) ) ;
#8173=DIRECTION ( 'NONE',  ( -2.698458740408365879E-16, 1.000000000000000000, 0.000000000000000000 ) ) ;
#8174=CARTESIAN_POINT ( 'NONE',  ( 90.99818021113283351, -4.999999999999992895, 66.11404789448386055 ) ) ;
#8177=CARTESIAN_POINT ( 'NONE',  ( 161.1922820468853104, -4.999999999999973355, -2.083034168790677043 ) ) ;
#8180=DIRECTION ( 'NONE',  ( -2.698458740408365879E-16, 1.000000000000000000, 0.000000000000000000 ) ) ;
#8181=ORIENTED_EDGE ( 'NONE', *, *, #23456, .F. ) ;
#8182=DIRECTION ( 'NONE',  ( 0.9510565162951536422, 2.566386769018988816E-16, 0.3090169943749472292 ) ) ;
#8183=ORIENTED_EDGE ( 'NONE', *, *, #28413, .F. ) ;
#8184=CARTESIAN_POINT ( 'NONE',  ( 169.5152310637604955, -1.999999999999970468, -19.94844914048349693 ) ) ;
#8185=CARTESIAN_POINT ( 'NONE',  ( 142.0152310637605808, -1.999999999999978018, -34.70218595412750773 ) ) ;
#8186=ORIENTED_EDGE ( 'NONE', *, *, #12796, .T. ) ;
#8187=AXIS2_PLACEMENT_3D ( 'NONE', #12075, #7504, #24139 ) ;
#8188=DIRECTION ( 'NONE',  ( 0.9510565162951536422, 2.566386769018988816E-16, 0.3090169943749472292 ) ) ;
#8189=ORIENTED_EDGE ( 'NONE', *, *, #15408, .F. ) ;
#8191=EDGE_LOOP ( 'NONE', ( #6884, #5679, #11382, #14263 ) ) ;
#8196=DIRECTION ( 'NONE',  ( -2.698458740408365879E-16, 1.000000000000000000, 0.000000000000000000 ) ) ;
#8197=DIRECTION ( 'NONE',  ( -2.698458740408365879E-16, 1.000000000000000000, 0.000000000000000000 ) ) ;
#8198=LINE ( 'NONE', #5930, #15227 ) ;
#8199=ORIENTED_EDGE ( 'NONE', *, *, #6496, .T. ) ;
#8200=LINE ( 'NONE', #27476, #4531 ) ;
#8201=EDGE_CURVE ( 'NONE', #28125, #20055, #30159, .T. ) ;
#8202=DIRECTION ( 'NONE',  ( -0.5877852522924731371, -1.586114251531760728E-16, -0.8090169943749474513 ) ) ;
#8204=DIRECTION ( 'NONE',  ( -0.5877852522924731371, 0.000000000000000000, 0.8090169943749474513 ) ) ;
#8205=DIRECTION ( 'NONE',  ( -2.698458740408365879E-16, 1.000000000000000000, 0.000000000000000000 ) ) ;
#8207=ORIENTED_EDGE ( 'NONE', *, *, #22743, .F. ) ;
#8209=VECTOR ( 'NONE', #29634, 1000.000000000000000 ) ;
#8210=EDGE_LOOP ( 'NONE', ( #28858, #15511, #26210, #23590 ) ) ;
#8215=FACE_BOUND ( 'NONE', #10855, .T. ) ;
#8216=VECTOR ( 'NONE', #3344, 1000.000000000000000 ) ;
#8217=ORIENTED_EDGE ( 'NONE', *, *, #6826, .F. ) ;
#8218=VECTOR ( 'NONE', #11818, 1000.000000000000000 ) ;
#8219=EDGE_LOOP ( 'NONE', ( #28152, #19450, #21967, #27077 ) ) ;
#8220=DIRECTION ( 'NONE',  ( -0.5877852522924731371, 0.000000000000000000, 0.8090169943749474513 ) ) ;
#8222=LINE ( 'NONE', #12955, #6721 ) ;
#8224=DIRECTION ( 'NONE',  ( 0.3090169943749472292, 8.338696094057992503E-17, -0.9510565162951536422 ) ) ;
#8225=ORIENTED_EDGE ( 'NONE', *, *, #21094, .T. ) ;
#8227=ORIENTED_EDGE ( 'NONE', *, *, #8456, .F. ) ;
#8231=EDGE_LOOP ( 'NONE', ( #1418, #5947, #25909, #26495, #5041 ) ) ;
#8233=AXIS2_PLACEMENT_3D ( 'NONE', #4016, #9327, #11176 ) ;
#8235=EDGE_LOOP ( 'NONE', ( #6189, #25865, #26058, #24971, #5509, #13845 ) ) ;
#8236=VECTOR ( 'NONE', #1001, 1000.000000000000000 ) ;
#8237=DIRECTION ( 'NONE',  ( -0.5877852522924731371, 0.000000000000000000, 0.8090169943749474513 ) ) ;
#8239=FACE_BOUND ( 'NONE', #3954, .T. ) ;
#8240=EDGE_CURVE ( 'NONE', #6979, #134, #25071, .T. ) ;
#8241=ADVANCED_FACE ( 'NONE', ( #27698 ), #20478, .T. ) ;
#8242=EDGE_CURVE ( 'NONE', #13963, #29180, #18190, .T. ) ;
#8244=DIRECTION ( 'NONE',  ( -0.5877852522924731371, 0.000000000000000000, 0.8090169943749474513 ) ) ;
#8246=DIRECTION ( 'NONE',  ( 0.000000000000000000, -1.000000000000000000, 0.000000000000000000 ) ) ;
#8247=ORIENTED_EDGE ( 'NONE', *, *, #4090, .T. ) ;
#8250=ORIENTED_EDGE ( 'NONE', *, *, #15791, .F. ) ;
#8252=ORIENTED_EDGE ( 'NONE', *, *, #20668, .F. ) ;
#8253=CARTESIAN_POINT ( 'NONE',  ( 141.1922820468854241, -10.00000000000000533, -2.083034168790677043 ) ) ;
#8254=ORIENTED_EDGE ( 'NONE', *, *, #16529, .F. ) ;
#8256=FACE_OUTER_BOUND ( 'NONE', #19531, .T. ) ;
#8259=ORIENTED_EDGE ( 'NONE', *, *, #5599, .F. ) ;
#8260=LINE ( 'NONE', #12536, #25654 ) ;
#8261=VERTEX_POINT ( 'NONE', #11017 ) ;
#8265=ORIENTED_EDGE ( 'NONE', *, *, #11109, .T. ) ;
#8266=ORIENTED_EDGE ( 'NONE', *, *, #18637, .T. ) ;
#8269=VERTEX_POINT ( 'NONE', #16045 ) ;
#8270=LINE ( 'NONE', #5995, #4238 ) ;
#8271=EDGE_CURVE ( 'NONE', #11681, #15913, #29868, .T. ) ;
#8275=ORIENTED_EDGE ( 'NONE', *, *, #24701, .F. ) ;
#8277=AXIS2_PLACEMENT_3D ( 'NONE', #17789, #15951, #18243 ) ;
#8278=ADVANCED_FACE ( 'NONE', ( #27253 ), #2189, .T. ) ;
#8279=CARTESIAN_POINT ( 'NONE',  ( 142.0152310637605240, -4.999999999999979572, -1.576685793744486963E-14 ) ) ;
#8281=EDGE_CURVE ( 'NONE', #25250, #16634, #6600, .T. ) ;
#8282=AXIS2_PLACEMENT_3D ( 'NONE', #2269, #25306, #29942 ) ;
#8283=CARTESIAN_POINT ( 'NONE',  ( 174.5152310637604955, -9.999999999999994671, -28.60870317832789667 ) ) ;
#8284=EDGE_CURVE ( 'NONE', #28008, #29920, #4311, .T. ) ;
#8285=CARTESIAN_POINT ( 'NONE',  ( 146.1922820468854525, -1.999999999999977129, -22.25671179336496053 ) ) ;
#8287=CARTESIAN_POINT ( 'NONE',  ( 151.1922820468853672, -10.00000000000000178, -2.083034168790677043 ) ) ;
#8292=ORIENTED_EDGE ( 'NONE', *, *, #11151, .F. ) ;
#8293=DIRECTION ( 'NONE',  ( 0.3090169943749475623, 8.338696094058001131E-17, 0.9510565162951536422 ) ) ;
#8294=DIRECTION ( 'NONE',  ( -1.110223024625156540E-16, 0.000000000000000000, -1.000000000000000000 ) ) ;
#8295=CARTESIAN_POINT ( 'NONE',  ( 152.0152310637604671, -4.999999999999976907, -17.38167787843870826 ) ) ;
#8296=AXIS2_PLACEMENT_3D ( 'NONE', #17892, #22347, #17605 ) ;
#8297=CARTESIAN_POINT ( 'NONE',  ( 148.6922820468854525, -10.00000000000000178, -32.39392330124607611 ) ) ;
#8298=DIRECTION ( 'NONE',  ( 0.9510565162951536422, 2.566386769018988816E-16, 0.3090169943749472292 ) ) ;
#8301=VERTEX_POINT ( 'NONE', #11458 ) ;
#8302=LINE ( 'NONE', #17757, #27129 ) ;
#8304=VECTOR ( 'NONE', #25486, 1000.000000000000000 ) ;
#8305=CARTESIAN_POINT ( 'NONE',  ( 125.7287565553229740, -84.33034373659255323, 0.5000000000000143219 ) ) ;
#8307=ORIENTED_EDGE ( 'NONE', *, *, #7157, .F. ) ;
#8309=DIRECTION ( 'NONE',  ( 0.9510565162951535312, 2.566386769018988816E-16, -0.3090169943749475623 ) ) ;
#8311=ORIENTED_EDGE ( 'NONE', *, *, #16565, .T. ) ;
#8312=LINE ( 'NONE', #3451, #10535 ) ;
#8319=DIRECTION ( 'NONE',  ( 1.110223024625156540E-16, 2.995891024602366092E-32, 1.000000000000000000 ) ) ;
#8320=VECTOR ( 'NONE', #22087, 1000.000000000000000 ) ;
#8321=EDGE_CURVE ( 'NONE', #23103, #9904, #18495, .T. ) ;
#8324=LINE ( 'NONE', #25712, #27026 ) ;
#8325=EDGE_CURVE ( 'NONE', #24130, #13154, #1734, .T. ) ;
#8327=CARTESIAN_POINT ( 'NONE',  ( 152.2287565553230309, -1.999999999999974465, -29.49038105676660493 ) ) ;
#8328=DIRECTION ( 'NONE',  ( -1.110223024625156540E-16, 0.000000000000000000, -1.000000000000000000 ) ) ;
#8329=LINE ( 'NONE', #22533, #6561 ) ;
#8334=CARTESIAN_POINT ( 'NONE',  ( 144.5152310637605808, -10.00000000000000178, -21.71180489736091346 ) ) ;
#8339=DIRECTION ( 'NONE',  ( -0.5877852522924731371, 0.000000000000000000, 0.8090169943749474513 ) ) ;
#8343=VECTOR ( 'NONE', #1307, 1000.000000000000000 ) ;
#8345=CARTESIAN_POINT ( 'NONE',  ( 139.5152310637605808, -4.999999999999980460, -1.548930218128858680E-14 ) ) ;
#8347=EDGE_LOOP ( 'NONE', ( #5767, #24125, #26984, #59, #20659 ) ) ;
#8353=CARTESIAN_POINT ( 'NONE',  ( 177.2287565553229172, -1.999999999999968026, -29.49038105676660493 ) ) ;
#8355=CARTESIAN_POINT ( 'NONE',  ( 120.2036091896494980, -4.999999999999985789, -87.33303409601636247 ) ) ;
#8356=ORIENTED_EDGE ( 'NONE', *, *, #19860, .F. ) ;
#8357=EDGE_CURVE ( 'NONE', #22145, #6733, #16350, .T. ) ;
#8358=ORIENTED_EDGE ( 'NONE', *, *, #4154, .T. ) ;
#8359=CARTESIAN_POINT ( 'NONE',  ( 154.7287565553230309, -1.999999999999973577, -33.82050807568879947 ) ) ;
#8360=EDGE_CURVE ( 'NONE', #20122, #27640, #21538, .T. ) ;
#8362=CARTESIAN_POINT ( 'NONE',  ( 153.6922820468853672, -10.00000000000000178, -9.266330736598359152 ) ) ;
#8363=CARTESIAN_POINT ( 'NONE',  ( 159.7287565553229456, -10.00000000000000000, -16.50000000000000355 ) ) ;
#8366=ORIENTED_EDGE ( 'NONE', *, *, #7725, .T. ) ;
#8368=ORIENTED_EDGE ( 'NONE', *, *, #28876, .T. ) ;
#8371=FACE_BOUND ( 'NONE', #17114, .T. ) ;
#8372=ORIENTED_EDGE ( 'NONE', *, *, #23136, .T. ) ;
#8373=LINE ( 'NONE', #6094, #27624 ) ;
#8375=VECTOR ( 'NONE', #20623, 1000.000000000000000 ) ;
#8377=EDGE_LOOP ( 'NONE', ( #6621, #9394, #12062, #28286 ) ) ;
#8378=DIRECTION ( 'NONE',  ( -2.698458740408365879E-16, 1.000000000000000000, 0.000000000000000000 ) ) ;
#8381=ADVANCED_FACE ( 'NONE', ( #28153 ), #27998, .T. ) ;
#8382=EDGE_LOOP ( 'NONE', ( #27558, #23623, #20555, #18508 ) ) ;
#8386=DIRECTION ( 'NONE',  ( -1.110223024625156540E-16, 0.000000000000000000, -1.000000000000000000 ) ) ;
#8387=VERTEX_POINT ( 'NONE', #18651 ) ;
#8388=CARTESIAN_POINT ( 'NONE',  ( 129.5152310637605524, -10.00000000000000888, -30.37205893520530964 ) ) ;
#8390=VECTOR ( 'NONE', #14386, 1000.000000000000000 ) ;
#8392=DIRECTION ( 'NONE',  ( -2.908569913943825554E-16, 1.000000000000000000, -6.826925868028084042E-18 ) ) ;
#8394=EDGE_LOOP ( 'NONE', ( #13823, #24088, #27029, #9633 ) ) ;
#8395=DIRECTION ( 'NONE',  ( 1.000000000000000000, 2.908569913943825554E-16, -6.938893903907227392E-16 ) ) ;
#8398=ORIENTED_EDGE ( 'NONE', *, *, #26935, .T. ) ;
#8399=PLANE ( 'NONE',  #15360 ) ;
#8402=DIRECTION ( 'NONE',  ( 0.5877852522924731371, 1.586114251531760728E-16, -0.8090169943749474513 ) ) ;
#8403=ORIENTED_EDGE ( 'NONE', *, *, #14272, .T. ) ;
#8406=VECTOR ( 'NONE', #4428, 1000.000000000000000 ) ;
#8408=CARTESIAN_POINT ( 'NONE',  ( 131.1922820468854241, -10.00000000000000888, -30.91696583120935671 ) ) ;
#8409=CARTESIAN_POINT ( 'NONE',  ( 138.6922820468854525, -4.999999999999980460, -35.24709285013155835 ) ) ;
#8410=CARTESIAN_POINT ( 'NONE',  ( 163.6922820468853672, -9.999999999999998224, -23.73366926340167637 ) ) ;
#8413=EDGE_CURVE ( 'NONE', #12010, #10075, #9781, .T. ) ;
#8414=ADVANCED_FACE ( 'NONE', ( #16502 ), #23685, .T. ) ;
#8418=ADVANCED_FACE ( 'NONE', ( #16657, #24001, #3097, #9631, #12224, #12366, #16956, #21230, #7652, #26285, #2943, #18950, #11768, #14347, #14049, #21389, #5367, #14207, #2636, #343, #21086, #21679, #4758, #7056, #640, #9473, #28302, #9325, #23376, #7359, #5058, #12069, #495, #19095, #16802, #28450, #2499, #192, #7503, #26134, #23843, #9925, #19240, #5519, #14799, #7946, #6112, #1102, #8239, #15407, #29368, #15102, #21837, #17396, #10529, #22288, #21990, #12822, #10379, #3382, #24436, #5668, #1395, #10076, #24137, #19997, #3239, #19689, #15255, #12517, #19836, #943, #29051, #3674, #13123, #8088, #10228, #26744 ), #5966, .T. ) ;
#8419=ORIENTED_EDGE ( 'NONE', *, *, #18340, .F. ) ;
#8420=DIRECTION ( 'NONE',  ( 0.5877852522924731371, 1.586114251531760728E-16, 0.8090169943749474513 ) ) ;
#8421=VECTOR ( 'NONE', #18870, 1000.000000000000000 ) ;
#8422=EDGE_CURVE ( 'NONE', #30027, #11898, #26584, .T. ) ;
#8423=CARTESIAN_POINT ( 'NONE',  ( 157.2287565553229740, -4.999999999999975131, -20.83012701892221585 ) ) ;
#8428=ORIENTED_EDGE ( 'NONE', *, *, #12170, .F. ) ;
#8429=VERTEX_POINT ( 'NONE', #14948 ) ;
#8431=CARTESIAN_POINT ( 'NONE',  ( 152.0152310637605240, -10.00000000000000178, -6.958068083716895558 ) ) ;
#8432=CARTESIAN_POINT ( 'NONE',  ( 98.38891821480183353, -4.999999999999990230, 71.48373336749482121 ) ) ;
#8435=DIRECTION ( 'NONE',  ( -0.8090169943749474513, -2.183098979609982436E-16, -0.5877852522924731371 ) ) ;
#8436=CARTESIAN_POINT ( 'NONE',  ( 142.0152310637605808, -1.999999999999978462, -6.958068083716895558 ) ) ;
#8442=DIRECTION ( 'NONE',  ( -0.5877852522924731371, -1.586114251531760235E-16, 0.8090169943749474513 ) ) ;
#8443=CARTESIAN_POINT ( 'NONE',  ( 163.6922820468853672, -9.999999999999998224, -26.58683881228715862 ) ) ;
#8444=ORIENTED_EDGE ( 'NONE', *, *, #15367, .F. ) ;
#8446=PLANE ( 'NONE',  #8296 ) ;
#8447=CARTESIAN_POINT ( 'NONE',  ( 159.7287565553228887, -10.00000000000000000, 0.8205080756887930260 ) ) ;
#8449=DIRECTION ( 'NONE',  ( -2.698458740408365879E-16, 1.000000000000000000, 0.000000000000000000 ) ) ;
#8451=AXIS2_PLACEMENT_3D ( 'NONE', #20417, #18583, #2426 ) ;
#8452=EDGE_CURVE ( 'NONE', #14013, #21320, #10687, .T. ) ;
#8455=ADVANCED_FACE ( 'NONE', ( #24743 ), #17696, .T. ) ;
#8456=EDGE_CURVE ( 'NONE', #27422, #2121, #785, .T. ) ;
#8458=DIRECTION ( 'NONE',  ( -2.698458740408365879E-16, 1.000000000000000000, 0.000000000000000000 ) ) ;
#8461=ORIENTED_EDGE ( 'NONE', *, *, #11576, .F. ) ;
#8462=LINE ( 'NONE', #15319, #14904 ) ;
#8463=ORIENTED_EDGE ( 'NONE', *, *, #23522, .F. ) ;
#8464=ORIENTED_EDGE ( 'NONE', *, *, #13351, .F. ) ;
#8468=VECTOR ( 'NONE', #6534, 1000.000000000000000 ) ;
#8469=ORIENTED_EDGE ( 'NONE', *, *, #11209, .T. ) ;
#8471=LINE ( 'NONE', #17327, #4080 ) ;
#8472=ORIENTED_EDGE ( 'NONE', *, *, #14473, .F. ) ;
#8474=CARTESIAN_POINT ( 'NONE',  ( 148.6922820468854525, -1.999999999999975797, -32.39392330124607611 ) ) ;
#8475=LINE ( 'NONE', #17775, #26544 ) ;
#8476=CARTESIAN_POINT ( 'NONE',  ( 132.0152310637605524, -10.00000000000000711, -26.04193191628310800 ) ) ;
#8482=AXIS2_PLACEMENT_3D ( 'NONE', #4505, #14092, #30201 ) ;
#8483=LINE ( 'NONE', #20377, #3472 ) ;
#8484=PLANE ( 'NONE',  #22714 ) ;
#8487=DIRECTION ( 'NONE',  ( -0.9510565162951536422, -2.566386769018988816E-16, -0.3090169943749472292 ) ) ;
#8492=EDGE_CURVE ( 'NONE', #12774, #10367, #28759, .T. ) ;
#8494=DIRECTION ( 'NONE',  ( -2.698458740408365879E-16, 1.000000000000000000, 0.000000000000000000 ) ) ;
#8495=ADVANCED_FACE ( 'NONE', ( #17551 ), #6269, .T. ) ;
#8496=ORIENTED_EDGE ( 'NONE', *, *, #19774, .F. ) ;
#8502=LINE ( 'NONE', #13380, #29226 ) ;
#8503=DIRECTION ( 'NONE',  ( -0.8090169943749474513, -2.183098979609982436E-16, -0.5877852522924731371 ) ) ;
#8504=DIRECTION ( 'NONE',  ( 0.9510565162951535312, 2.566386769018988816E-16, -0.3090169943749475623 ) ) ;
#8505=VECTOR ( 'NONE', #22178, 1000.000000000000000 ) ;
#8507=ORIENTED_EDGE ( 'NONE', *, *, #10268, .T. ) ;
#8508=FACE_OUTER_BOUND ( 'NONE', #16650, .T. ) ;
#8509=ORIENTED_EDGE ( 'NONE', *, *, #1042, .T. ) ;
#8511=ORIENTED_EDGE ( 'NONE', *, *, #26826, .F. ) ;
#8514=ORIENTED_EDGE ( 'NONE', *, *, #18561, .F. ) ;
#8521=DIRECTION ( 'NONE',  ( 1.000000000000000000, 2.698458740408365879E-16, -1.110223024625156540E-16 ) ) ;
#8522=ORIENTED_EDGE ( 'NONE', *, *, #12371, .F. ) ;
#8523=LINE ( 'NONE', #15545, #22207 ) ;
#8524=EDGE_CURVE ( 'NONE', #9448, #23002, #18298, .T. ) ;
#8525=AXIS2_PLACEMENT_3D ( 'NONE', #10421, #27259, #5715 ) ;
#8527=DIRECTION ( 'NONE',  ( -0.5877852522924731371, 0.000000000000000000, 0.8090169943749474513 ) ) ;
#8528=CARTESIAN_POINT ( 'NONE',  ( 142.0152310637606092, -1.999999999999978018, -32.93883019725009120 ) ) ;
#8529=ORIENTED_EDGE ( 'NONE', *, *, #18596, .T. ) ;
#8530=EDGE_CURVE ( 'NONE', #22161, #19955, #27810, .T. ) ;
#8534=DIRECTION ( 'NONE',  ( 0.9510565162951536422, 2.566386769018988816E-16, 0.3090169943749472292 ) ) ;
#8535=ORIENTED_EDGE ( 'NONE', *, *, #29953, .T. ) ;
#8536=CARTESIAN_POINT ( 'NONE',  ( 154.5152310637604671, -1.999999999999975353, -4.391296821672111328 ) ) ;
#8538=FACE_OUTER_BOUND ( 'NONE', #8058, .T. ) ;
#8539=CARTESIAN_POINT ( 'NONE',  ( 132.0152310637605808, -10.00000000000000711, -32.93883019725009120 ) ) ;
#8540=VECTOR ( 'NONE', #8547, 1000.000000000000000 ) ;
#8543=DIRECTION ( 'NONE',  ( -6.938893903907227392E-16, 0.000000000000000000, -1.000000000000000000 ) ) ;
#8545=DIRECTION ( 'NONE',  ( 0.9510565162951536422, 2.566386769018988816E-16, 0.3090169943749472292 ) ) ;
#8547=DIRECTION ( 'NONE',  ( -0.5877852522924731371, -1.586114251531760235E-16, 0.8090169943749474513 ) ) ;
#8551=ORIENTED_EDGE ( 'NONE', *, *, #27038, .F. ) ;
#8553=AXIS2_PLACEMENT_3D ( 'NONE', #13262, #22580, #4258 ) ;
#8556=CARTESIAN_POINT ( 'NONE',  ( 143.6922820468854525, -1.999999999999978018, -17.92658477444275889 ) ) ;
#8557=VERTEX_POINT ( 'NONE', #11137 ) ;
#8558=CARTESIAN_POINT ( 'NONE',  ( 147.0152310637605524, -4.999999999999977796, -6.958068083716895558 ) ) ;
#8559=VERTEX_POINT ( 'NONE', #6720 ) ;
#8561=ORIENTED_EDGE ( 'NONE', *, *, #25875, .T. ) ;
#8562=VECTOR ( 'NONE', #21446, 1000.000000000000000 ) ;
#8565=EDGE_LOOP ( 'NONE', ( #9605, #29472, #19777, #4770 ) ) ;
#8566=CARTESIAN_POINT ( 'NONE',  ( 148.6922820468854525, -4.999999999999977796, -26.58683881228715862 ) ) ;
#8567=ORIENTED_EDGE ( 'NONE', *, *, #1969, .T. ) ;
#8568=CARTESIAN_POINT ( 'NONE',  ( 149.7287565553229740, -1.999999999999976241, -7.839745962155603820 ) ) ;
#8573=ORIENTED_EDGE ( 'NONE', *, *, #7202, .T. ) ;
#8574=CARTESIAN_POINT ( 'NONE',  ( 162.0152310637604103, -9.999999999999998224, -0.06116980274991495881 ) ) ;
#8577=DIRECTION ( 'NONE',  ( -0.8090169943749474513, -2.183098979609982436E-16, -0.5877852522924731371 ) ) ;
#8578=EDGE_CURVE ( 'NONE', #3931, #30101, #22748, .T. ) ;
#8580=DIRECTION ( 'NONE',  ( 0.3090169943749472292, 8.338696094057992503E-17, -0.9510565162951536422 ) ) ;
#8581=VECTOR ( 'NONE', #23251, 1000.000000000000000 ) ;
#8582=EDGE_CURVE ( 'NONE', #24297, #18704, #20287, .T. ) ;
#8587=CARTESIAN_POINT ( 'NONE',  ( 157.0152310637604387, -10.00000000000000000, -0.06116980274991495881 ) ) ;
#8589=LINE ( 'NONE', #8443, #8105 ) ;
#8590=ORIENTED_EDGE ( 'NONE', *, *, #10381, .T. ) ;
#8592=DIRECTION ( 'NONE',  ( 1.000000000000000000, 2.698458740408365879E-16, -1.110223024625156540E-16 ) ) ;
#8594=DIRECTION ( 'NONE',  ( 0.5877852522924731371, 1.586114251531760728E-16, -0.8090169943749474513 ) ) ;
#8597=ORIENTED_EDGE ( 'NONE', *, *, #27871, .T. ) ;
#8598=CARTESIAN_POINT ( 'NONE',  ( 5.749818843786239420, -5.000000000000015987, 17.69612279726095139 ) ) ;
#8604=DIRECTION ( 'NONE',  ( 1.000000000000000000, 2.698458740408365879E-16, -1.110223024625156540E-16 ) ) ;
#8606=ORIENTED_EDGE ( 'NONE', *, *, #26706, .T. ) ;
#8608=SHAPE_REPRESENTATION_RELATIONSHIP ( 'NONE' , 'NONE' ,  #16744, #13457 ) ;
#8610=VECTOR ( 'NONE', #2171, 1000.000000000000000 ) ;
#8613=ORIENTED_EDGE ( 'NONE', *, *, #17786, .T. ) ;
#8616=DIRECTION ( 'NONE',  ( -2.698458740408365879E-16, 1.000000000000000000, 0.000000000000000000 ) ) ;
#8617=EDGE_CURVE ( 'NONE', #21141, #5593, #16010, .T. ) ;
#8619=CARTESIAN_POINT ( 'NONE',  ( 102.5724172122712474, -4.999999999999989342, -74.52322330502413195 ) ) ;
#8621=DIRECTION ( 'NONE',  ( 0.9510565162951535312, 2.566386769018988816E-16, -0.3090169943749475623 ) ) ;
#8623=EDGE_CURVE ( 'NONE', #14471, #12367, #16163, .T. ) ;
#8629=VECTOR ( 'NONE', #17614, 1000.000000000000000 ) ;
#8634=DIRECTION ( 'NONE',  ( 0.5877852522924731371, 1.586114251531760728E-16, -0.8090169943749474513 ) ) ;
#8635=CARTESIAN_POINT ( 'NONE',  ( 147.0152310637605808, -10.00000000000000178, -34.70218595412750773 ) ) ;
#8637=VERTEX_POINT ( 'NONE', #17841 ) ;
#8638=CARTESIAN_POINT ( 'NONE',  ( 139.7287565553230024, -1.999999999999979128, 0.8205080756887930260 ) ) ;
#8640=LINE ( 'NONE', #10929, #9774 ) ;
#8641=ORIENTED_EDGE ( 'NONE', *, *, #27, .T. ) ;
#8647=DIRECTION ( 'NONE',  ( 0.9510565162951536422, 2.566386769018988816E-16, 0.3090169943749472292 ) ) ;
#8648=DIRECTION ( 'NONE',  ( -2.698458740408365879E-16, 1.000000000000000000, 0.000000000000000000 ) ) ;
#8650=VECTOR ( 'NONE', #5660, 1000.000000000000000 ) ;
#8651=VERTEX_POINT ( 'NONE', #20731 ) ;
#8652=LINE ( 'NONE', #17960, #7469 ) ;
#8653=DIRECTION ( 'NONE',  ( -2.698458740408365879E-16, 1.000000000000000000, 0.000000000000000000 ) ) ;
#8654=ORIENTED_EDGE ( 'NONE', *, *, #11376, .F. ) ;
#8655=ADVANCED_FACE ( 'NONE', ( #24896 ), #10832, .T. ) ;
#8656=LINE ( 'NONE', #2381, #28837 ) ;
#8657=CARTESIAN_POINT ( 'NONE',  ( 142.2287565553230309, -10.00000000000000533, -12.16987298107780369 ) ) ;
#8658=ADVANCED_FACE ( 'NONE', ( #22449 ), #8981, .T. ) ;
#8659=ADVANCED_FACE ( 'NONE', ( #1696 ), #29835, .T. ) ;
#8660=EDGE_CURVE ( 'NONE', #20055, #10866, #8687, .T. ) ;
#8661=LINE ( 'NONE', #29802, #12664 ) ;
#8663=VERTEX_POINT ( 'NONE', #6424 ) ;
#8665=ORIENTED_EDGE ( 'NONE', *, *, #15201, .T. ) ;
#8666=VECTOR ( 'NONE', #22830, 1000.000000000000000 ) ;
#8668=CARTESIAN_POINT ( 'NONE',  ( 142.0152310637605808, -10.00000000000000355, -6.958068083716895558 ) ) ;
#8670=PLANE ( 'NONE',  #8756 ) ;
#8672=VECTOR ( 'NONE', #9422, 1000.000000000000000 ) ;
#8673=CARTESIAN_POINT ( 'NONE',  ( 2.698458740408370316E-15, -10.00000000000001776, 0.000000000000000000 ) ) ;
#8677=EDGE_LOOP ( 'NONE', ( #22271, #227, #796, #13634 ) ) ;
#8683=CARTESIAN_POINT ( 'NONE',  ( 132.2287565553230024, -4.999999999999982236, -3.509618943233400401 ) ) ;
#8685=VECTOR ( 'NONE', #26112, 1000.000000000000000 ) ;
#8687=LINE ( 'NONE', #27370, #26449 ) ;
#8691=EDGE_LOOP ( 'NONE', ( #6325, #27663, #8464, #20415 ) ) ;
#8692=EDGE_CURVE ( 'NONE', #26883, #13495, #4129, .T. ) ;
#8693=EDGE_CURVE ( 'NONE', #21590, #30106, #7015, .T. ) ;
#8694=LINE ( 'NONE', #3833, #26842 ) ;
#8697=EDGE_LOOP ( 'NONE', ( #4899, #29824, #12951, #177, #1206 ) ) ;
#8698=DIRECTION ( 'NONE',  ( -2.698458740408365879E-16, 1.000000000000000000, 0.000000000000000000 ) ) ;
#8701=CARTESIAN_POINT ( 'NONE',  ( 159.5152310637604671, -9.999999999999998224, -13.05155085951651195 ) ) ;
#8702=VERTEX_POINT ( 'NONE', #11727 ) ;
#8703=LINE ( 'NONE', #10702, #29380 ) ;
#8706=CARTESIAN_POINT ( 'NONE',  ( 154.5152310637605240, -4.999999999999976019, -21.71180489736091346 ) ) ;
#8708=LINE ( 'NONE', #8410, #8131 ) ;
#8709=ORIENTED_EDGE ( 'NONE', *, *, #234, .T. ) ;
#8711=VECTOR ( 'NONE', #15520, 1000.000000000000000 ) ;
#8714=VERTEX_POINT ( 'NONE', #5171 ) ;
#8715=VERTEX_POINT ( 'NONE', #2901 ) ;
#8716=LINE ( 'NONE', #17866, #890 ) ;
#8721=ORIENTED_EDGE ( 'NONE', *, *, #1806, .T. ) ;
#8722=ORIENTED_EDGE ( 'NONE', *, *, #24223, .T. ) ;
#8723=DIRECTION ( 'NONE',  ( 1.000000000000000000, 2.698458740408365879E-16, -1.110223024625156540E-16 ) ) ;
#8724=ADVANCED_FACE ( 'NONE', ( #9283 ), #18754, .T. ) ;
#8726=AXIS2_PLACEMENT_3D ( 'NONE', #25673, #19099, #12370 ) ;
#8727=CARTESIAN_POINT ( 'NONE',  ( 133.7287565553229172, -4.999999999999982236, -36.50000000000000711 ) ) ;
#8733=CARTESIAN_POINT ( 'NONE',  ( 147.0152310637605524, -10.00000000000000178, -17.38167787843871182 ) ) ;
#8734=ORIENTED_EDGE ( 'NONE', *, *, #26052, .F. ) ;
#8735=LINE ( 'NONE', #15462, #22934 ) ;
#8736=EDGE_LOOP ( 'NONE', ( #4589, #27826, #11695, #7069 ) ) ;
#8737=DIRECTION ( 'NONE',  ( 0.9510565162951536422, 2.566386769018988816E-16, 0.3090169943749472292 ) ) ;
#8739=DIRECTION ( 'NONE',  ( -1.000000000000000000, 0.000000000000000000, 1.779203565104417375E-16 ) ) ;
#8740=LINE ( 'NONE', #18511, #6305 ) ;
#8742=EDGE_LOOP ( 'NONE', ( #12322, #1350, #5746, #28860 ) ) ;
#8743=ORIENTED_EDGE ( 'NONE', *, *, #23877, .T. ) ;
#8744=CARTESIAN_POINT ( 'NONE',  ( 172.7287565553229456, -3.999999999999989786, 0.5000000000000029976 ) ) ;
#8747=DIRECTION ( 'NONE',  ( 0.3090169943749472292, 8.338696094057992503E-17, -0.9510565162951536422 ) ) ;
#8749=LINE ( 'NONE', #18365, #19367 ) ;
#8754=EDGE_CURVE ( 'NONE', #7452, #19213, #18608, .T. ) ;
#8755=EDGE_LOOP ( 'NONE', ( #16212, #2049, #13370, #22909, #14929 ) ) ;
#8756=AXIS2_PLACEMENT_3D ( 'NONE', #4256, #22879, #27787 ) ;
#8759=VECTOR ( 'NONE', #23307, 1000.000000000000000 ) ;
#8760=ORIENTED_EDGE ( 'NONE', *, *, #15591, .F. ) ;
#8761=ORIENTED_EDGE ( 'NONE', *, *, #19856, .F. ) ;
#8762=LINE ( 'NONE', #15783, #20480 ) ;
#8763=CARTESIAN_POINT ( 'NONE',  ( 159.7287565553229172, -1.999999999999973577, -7.839745962155603820 ) ) ;
#8764=ORIENTED_EDGE ( 'NONE', *, *, #23303, .F. ) ;
#8765=CARTESIAN_POINT ( 'NONE',  ( 144.7287565553230309, -1.999999999999977129, -25.16025403784439973 ) ) ;
#8768=CARTESIAN_POINT ( 'NONE',  ( 169.7287565553229740, -1.999999999999969580, -33.82050807568879947 ) ) ;
#8769=FACE_OUTER_BOUND ( 'NONE', #25881, .T. ) ;
#8770=DIRECTION ( 'NONE',  ( -2.698458740408365879E-16, 1.000000000000000000, 0.000000000000000000 ) ) ;
#8774=ORIENTED_EDGE ( 'NONE', *, *, #4535, .F. ) ;
#8781=ORIENTED_EDGE ( 'NONE', *, *, #27860, .F. ) ;
#8782=CARTESIAN_POINT ( 'NONE',  ( 172.7287565553229456, -1.999999999999970468, 6.499999999999980460 ) ) ;
#8784=VERTEX_POINT ( 'NONE', #14163 ) ;
#8785=DIRECTION ( 'NONE',  ( 0.3090169943749472292, 8.338696094057992503E-17, -0.9510565162951536422 ) ) ;
#8786=DIRECTION ( 'NONE',  ( -0.9510565162951536422, -2.566386769018988323E-16, 0.3090169943749475623 ) ) ;
#8787=DIRECTION ( 'NONE',  ( -2.698458740408365879E-16, 1.000000000000000000, 0.000000000000000000 ) ) ;
#8788=ORIENTED_EDGE ( 'NONE', *, *, #6474, .F. ) ;
#8791=VECTOR ( 'NONE', #29778, 1000.000000000000000 ) ;
#8792=EDGE_CURVE ( 'NONE', #16514, #23037, #25937, .T. ) ;
#8793=ADVANCED_FACE ( 'NONE', ( #28555 ), #16459, .F. ) ;
#8796=ADVANCED_FACE ( 'NONE', ( #14463 ), #9587, .T. ) ;
#8798=LINE ( 'NONE', #27164, #8209 ) ;
#8799=EDGE_CURVE ( 'NONE', #20749, #11253, #18908, .T. ) ;
#8800=DIRECTION ( 'NONE',  ( -0.5877852522924731371, -1.586114251531760235E-16, 0.8090169943749474513 ) ) ;
#8802=VECTOR ( 'NONE', #14090, 1000.000000000000000 ) ;
#8803=ORIENTED_EDGE ( 'NONE', *, *, #9409, .F. ) ;
#8804=DIRECTION ( 'NONE',  ( -0.9510565162951536422, -2.566386769018988323E-16, 0.3090169943749475623 ) ) ;
#8808=LINE ( 'NONE', #18117, #9426 ) ;
#8809=VECTOR ( 'NONE', #18239, 1000.000000000000000 ) ;
#8810=DIRECTION ( 'NONE',  ( 0.000000000000000000, 0.000000000000000000, -1.000000000000000000 ) ) ;
#8812=ORIENTED_EDGE ( 'NONE', *, *, #4983, .F. ) ;
#8813=VECTOR ( 'NONE', #9195, 1000.000000000000000 ) ;
#8819=CARTESIAN_POINT ( 'NONE',  ( 162.0152310637604387, -4.999999999999974243, -1.798730398669517324E-14 ) ) ;
#8821=ORIENTED_EDGE ( 'NONE', *, *, #21387, .T. ) ;
#8822=DIRECTION ( 'NONE',  ( -2.908569913943825554E-16, 1.000000000000000000, -6.826925868028084042E-18 ) ) ;
#8824=CARTESIAN_POINT ( 'NONE',  ( 154.5152310637604955, -1.999999999999974909, -13.05155085951651195 ) ) ;
#8825=ORIENTED_EDGE ( 'NONE', *, *, #15753, .T. ) ;
#8826=FACE_OUTER_BOUND ( 'NONE', #23213, .T. ) ;
#8827=ORIENTED_EDGE ( 'NONE', *, *, #10448, .F. ) ;
#8829=EDGE_CURVE ( 'NONE', #15396, #23103, #25624, .T. ) ;
#8833=EDGE_CURVE ( 'NONE', #17684, #22172, #300, .T. ) ;
#8835=CARTESIAN_POINT ( 'NONE',  ( 174.5152310637604103, -4.999999999999970690, -13.05155085951651195 ) ) ;
#8836=EDGE_CURVE ( 'NONE', #24130, #11673, #14309, .T. ) ;
#8837=DIRECTION ( 'NONE',  ( 2.908569913943825554E-16, -1.000000000000000000, 0.000000000000000000 ) ) ;
#8838=VECTOR ( 'NONE', #24907, 1000.000000000000000 ) ;
#8842=ORIENTED_EDGE ( 'NONE', *, *, #12830, .F. ) ;
#8846=EDGE_LOOP ( 'NONE', ( #11736, #610, #16645, #7825 ) ) ;
#8847=LINE ( 'NONE', #4286, #10962 ) ;
#8853=DIRECTION ( 'NONE',  ( 0.3090169943749472292, 8.338696094057992503E-17, -0.9510565162951536422 ) ) ;
#8855=PLANE ( 'NONE',  #22951 ) ;
#8856=PLANE ( 'NONE',  #1353 ) ;
#8857=ORIENTED_EDGE ( 'NONE', *, *, #14909, .T. ) ;
#8858=CARTESIAN_POINT ( 'NONE',  ( 149.5152310637604955, -4.999999999999976907, -4.391296821672111328 ) ) ;
#8859=ORIENTED_EDGE ( 'NONE', *, *, #9202, .F. ) ;
#8863=VERTEX_POINT ( 'NONE', #7608 ) ;
#8866=ORIENTED_EDGE ( 'NONE', *, *, #14949, .T. ) ;
#8868=DIRECTION ( 'NONE',  ( -1.000000000000000000, -2.908569913943825554E-16, 0.000000000000000000 ) ) ;
#8870=ADVANCED_FACE ( 'NONE', ( #21345 ), #26244, .T. ) ;
#8871=LINE ( 'NONE', #6594, #24490 ) ;
#8876=EDGE_LOOP ( 'NONE', ( #22397, #23555, #24311, #15870 ) ) ;
#8878=CARTESIAN_POINT ( 'NONE',  ( 161.1922820468853104, -10.00000000000000000, -2.083034168790677043 ) ) ;
#8879=LINE ( 'NONE', #23089, #14086 ) ;
#8880=AXIS2_PLACEMENT_3D ( 'NONE', #27056, #12672, #5818 ) ;
#8884=CARTESIAN_POINT ( 'NONE',  ( 158.6922820468853388, -10.00000000000000000, -6.413161187712876909 ) ) ;
#8886=CARTESIAN_POINT ( 'NONE',  ( 163.6922820468852819, -1.999999999999972689, 2.247092850131518826 ) ) ;
#8887=VECTOR ( 'NONE', #13684, 1000.000000000000000 ) ;
#8889=CARTESIAN_POINT ( 'NONE',  ( 16.48213915071852398, -5.000000000000013323, -50.72680832159814912 ) ) ;
#8890=CARTESIAN_POINT ( 'NONE',  ( 164.5152310637604671, -4.999999999999973355, -21.71180489736091346 ) ) ;
#8891=ORIENTED_EDGE ( 'NONE', *, *, #7364, .T. ) ;
#8893=EDGE_LOOP ( 'NONE', ( #25261, #8181, #2512, #24168 ) ) ;
#8894=ORIENTED_EDGE ( 'NONE', *, *, #16999, .F. ) ;
#8895=DIRECTION ( 'NONE',  ( -0.5877852522924731371, 0.000000000000000000, 0.8090169943749474513 ) ) ;
#8898=CARTESIAN_POINT ( 'NONE',  ( 138.6922820468853956, -1.999999999999979572, 2.247092850131519715 ) ) ;
#8902=ORIENTED_EDGE ( 'NONE', *, *, #28323, .F. ) ;
#8904=CARTESIAN_POINT ( 'NONE',  ( 129.5152310637605808, -10.00000000000000888, -19.94844914048349338 ) ) ;
#8907=VECTOR ( 'NONE', #10340, 1000.000000000000000 ) ;
#8910=CARTESIAN_POINT ( 'NONE',  ( 139.5152310637606092, -1.999999999999978684, -19.94844914048349338 ) ) ;
#8912=FACE_OUTER_BOUND ( 'NONE', #16935, .T. ) ;
#8913=DIRECTION ( 'NONE',  ( 0.3090169943749475623, 8.338696094058001131E-17, 0.9510565162951536422 ) ) ;
#8916=DIRECTION ( 'NONE',  ( 0.9510565162951536422, 0.000000000000000000, -0.3090169943749475623 ) ) ;
#8919=EDGE_CURVE ( 'NONE', #18472, #13174, #7169, .T. ) ;
#8922=DIRECTION ( 'NONE',  ( -0.5877852522924731371, -1.586114251531760728E-16, -0.8090169943749474513 ) ) ;
#8924=CARTESIAN_POINT ( 'NONE',  ( 173.6922820468853388, -1.999999999999969358, -23.73366926340167637 ) ) ;
#8925=CARTESIAN_POINT ( 'NONE',  ( 138.6922820468854525, -4.999999999999980460, -17.92658477444275533 ) ) ;
#8927=DIRECTION ( 'NONE',  ( -0.9510565162951536422, -2.566386769018988816E-16, -0.3090169943749472292 ) ) ;
#8928=DIRECTION ( 'NONE',  ( 0.5877852522924731371, 0.000000000000000000, 0.8090169943749474513 ) ) ;
#8930=ORIENTED_EDGE ( 'NONE', *, *, #19998, .F. ) ;
#8931=LINE ( 'NONE', #18249, #16867 ) ;
#8932=CARTESIAN_POINT ( 'NONE',  ( 173.6922820468853672, -1.999999999999968914, -32.39392330124607611 ) ) ;
#8933=CARTESIAN_POINT ( 'NONE',  ( 132.2287565553230024, -10.00000000000000888, -20.83012701892220164 ) ) ;
#8934=AXIS2_PLACEMENT_3D ( 'NONE', #6195, #1474, #15487 ) ;
#8935=ORIENTED_EDGE ( 'NONE', *, *, #29954, .F. ) ;
#8936=EDGE_CURVE ( 'NONE', #117, #21069, #21802, .T. ) ;
#8946=LINE ( 'NONE', #18573, #6314 ) ;
#8947=EDGE_LOOP ( 'NONE', ( #15622, #1574, #18575, #29313 ) ) ;
#8948=PLANE ( 'NONE',  #25525 ) ;
#8949=VECTOR ( 'NONE', #28415, 1000.000000000000000 ) ;
#8950=CARTESIAN_POINT ( 'NONE',  ( 174.5152310637604387, -9.999999999999994671, -21.71180489736091346 ) ) ;
#8952=EDGE_CURVE ( 'NONE', #23002, #17166, #28710, .T. ) ;
#8953=ADVANCED_FACE ( 'NONE', ( #12477 ), #14759, .T. ) ;
#8956=EDGE_CURVE ( 'NONE', #12555, #4706, #3200, .T. ) ;
#8958=CARTESIAN_POINT ( 'NONE',  ( 166.1922820468853104, -9.999999999999998224, -4.936203717676158398 ) ) ;
#8960=CARTESIAN_POINT ( 'NONE',  ( 172.0152310637604671, -9.999999999999994671, -26.04193191628311155 ) ) ;
#8961=LINE ( 'NONE', #29378, #17389 ) ;
#8962=ORIENTED_EDGE ( 'NONE', *, *, #11617, .F. ) ;
#8963=ORIENTED_EDGE ( 'NONE', *, *, #24952, .T. ) ;
#8966=EDGE_LOOP ( 'NONE', ( #1841, #22925, #13547, #21030 ) ) ;
#8967=ORIENTED_EDGE ( 'NONE', *, *, #4950, .F. ) ;
#8968=CARTESIAN_POINT ( 'NONE',  ( 139.7287565553230309, -1.999999999999978684, -25.16025403784439973 ) ) ;
#8971=ORIENTED_EDGE ( 'NONE', *, *, #18557, .F. ) ;
#8977=FACE_OUTER_BOUND ( 'NONE', #1497, .T. ) ;
#8979=FILL_AREA_STYLE ('',( #23643 ) ) ;
#8980=EDGE_CURVE ( 'NONE', #21422, #29780, #26547, .T. ) ;
#8981=PLANE ( 'NONE',  #21076 ) ;
#8983=EDGE_CURVE ( 'NONE', #10906, #26227, #14613, .T. ) ;
#8985=PLANE ( 'NONE',  #26322 ) ;
#8986=VERTEX_POINT ( 'NONE', #1063 ) ;
#8987=EDGE_CURVE ( 'NONE', #11708, #2172, #29015, .T. ) ;
#8988=EDGE_CURVE ( 'NONE', #18123, #27662, #26397, .T. ) ;
#8989=CARTESIAN_POINT ( 'NONE',  ( 129.5152310637605808, -10.00000000000000888, -2.627941064794695691 ) ) ;
#8991=EDGE_CURVE ( 'NONE', #16958, #2560, #10035, .T. ) ;
#8994=LINE ( 'NONE', #18312, #23384 ) ;
#8995=ORIENTED_EDGE ( 'NONE', *, *, #28841, .T. ) ;
#8999=CARTESIAN_POINT ( 'NONE',  ( 134.7287565553230024, -10.00000000000000711, -7.839745962155602044 ) ) ;
#9000=FACE_OUTER_BOUND ( 'NONE', #5788, .T. ) ;
#9001=CARTESIAN_POINT ( 'NONE',  ( 137.2287565553230309, -10.00000000000000533, -12.16987298107780013 ) ) ;
#9002=VERTEX_POINT ( 'NONE', #10689 ) ;
#9004=VECTOR ( 'NONE', #14140, 1000.000000000000000 ) ;
#9014=DIRECTION ( 'NONE',  ( 0.9510565162951536422, 2.566386769018988816E-16, 0.3090169943749472292 ) ) ;
#9016=CARTESIAN_POINT ( 'NONE',  ( 119.7807826737523271, -4.999999999999985789, -87.02583265024875914 ) ) ;
#9018=ADVANCED_FACE ( 'NONE', ( #26749 ), #1399, .T. ) ;
#9019=PLANE ( 'NONE',  #18260 ) ;
#9020=VECTOR ( 'NONE', #28541, 1000.000000000000000 ) ;
#9021=EDGE_CURVE ( 'NONE', #16825, #17911, #22138, .T. ) ;
#9022=ADVANCED_FACE ( 'NONE', ( #8091 ), #22452, .T. ) ;
#9024=EDGE_CURVE ( 'NONE', #16967, #24164, #13125, .T. ) ;
#9026=DIRECTION ( 'NONE',  ( -0.8090169943749474513, -2.183098979609982436E-16, -0.5877852522924731371 ) ) ;
#9028=AXIS2_PLACEMENT_3D ( 'NONE', #29952, #27939, #11706 ) ;
#9032=CARTESIAN_POINT ( 'NONE',  ( 137.0152310637605808, -4.999999999999980460, -1.521174642513229767E-14 ) ) ;
#9033=DIRECTION ( 'NONE',  ( 0.5877852522924731371, 1.586114251531760728E-16, 0.8090169943749474513 ) ) ;
#9035=ORIENTED_EDGE ( 'NONE', *, *, #18168, .F. ) ;
#9036=VERTEX_POINT ( 'NONE', #26907 ) ;
#9039=CIRCLE ( 'NONE', #3711, 8.000000000000007105 ) ;
#9042=ORIENTED_EDGE ( 'NONE', *, *, #11288, .F. ) ;
#9043=CARTESIAN_POINT ( 'NONE',  ( 159.5152310637605240, -1.999999999999973133, -19.94844914048349693 ) ) ;
#9045=ORIENTED_EDGE ( 'NONE', *, *, #28003, .F. ) ;
#9046=DIRECTION ( 'NONE',  ( -0.9510565162951536422, 0.000000000000000000, -0.3090169943749472292 ) ) ;
#9050=ORIENTED_EDGE ( 'NONE', *, *, #10517, .T. ) ;
#9051=EDGE_CURVE ( 'NONE', #29151, #25751, #1104, .T. ) ;
#9052=LINE ( 'NONE', #11496, #3920 ) ;
#9053=VECTOR ( 'NONE', #6174, 1000.000000000000000 ) ;
#9054=AXIS2_PLACEMENT_3D ( 'NONE', #17450, #10739, #13026 ) ;
#9056=CARTESIAN_POINT ( 'NONE',  ( 158.6922820468853388, -1.999999999999974465, -6.413161187712876909 ) ) ;
#9057=CARTESIAN_POINT ( 'NONE',  ( 147.0152310637605808, -1.999999999999976241, -34.70218595412750773 ) ) ;
#9061=CARTESIAN_POINT ( 'NONE',  ( 142.0152310637605808, -10.00000000000000355, -26.04193191628310800 ) ) ;
#9062=EDGE_CURVE ( 'NONE', #18724, #24484, #6115, .T. ) ;
#9069=CARTESIAN_POINT ( 'NONE',  ( 152.2287565553229740, -1.999999999999975353, -12.16987298107780369 ) ) ;
#9072=LINE ( 'NONE', #27310, #13641 ) ;
#9073=EDGE_LOOP ( 'NONE', ( #21391, #11479, #27776, #18935 ) ) ;
#9074=CARTESIAN_POINT ( 'NONE',  ( 138.6922820468854241, -10.00000000000000533, -0.6060766987539614181 ) ) ;
#9077=VECTOR ( 'NONE', #17897, 999.9999999999998863 ) ;
#9078=CARTESIAN_POINT ( 'NONE',  ( 175.7287565553229456, -4.999999999999970690, 0.5000000000000029976 ) ) ;
#9079=CARTESIAN_POINT ( 'NONE',  ( 132.0152310637605524, -4.999999999999982236, -8.721423840594310306 ) ) ;
#9081=AXIS2_PLACEMENT_3D ( 'NONE', #505, #18505, #25528 ) ;
#9083=VERTEX_POINT ( 'NONE', #6272 ) ;
#9087=AXIS2_PLACEMENT_3D ( 'NONE', #17878, #26948, #3871 ) ;
#9092=EDGE_CURVE ( 'NONE', #19566, #26769, #6426, .T. ) ;
#9093=VECTOR ( 'NONE', #21570, 1000.000000000000000 ) ;
#9094=ORIENTED_EDGE ( 'NONE', *, *, #16523, .F. ) ;
#9095=DIRECTION ( 'NONE',  ( -2.698458740408365879E-16, 1.000000000000000000, 0.000000000000000000 ) ) ;
#9099=CARTESIAN_POINT ( 'NONE',  ( 164.5152310637604955, -1.999999999999971800, -19.94844914048349693 ) ) ;
#9103=ORIENTED_EDGE ( 'NONE', *, *, #20132, .T. ) ;
#9105=LINE ( 'NONE', #8958, #28968 ) ;
#9107=FACE_BOUND ( 'NONE', #24867, .T. ) ;
#9108=CARTESIAN_POINT ( 'NONE',  ( 167.0152310637604671, -1.999999999999971800, -6.958068083716895558 ) ) ;
#9109=ORIENTED_EDGE ( 'NONE', *, *, #11151, .T. ) ;
#9111=CIRCLE ( 'NONE', #385, 3.000000000000002665 ) ;
#9113=LINE ( 'NONE', #30254, #1820 ) ;
#9114=ORIENTED_EDGE ( 'NONE', *, *, #17624, .T. ) ;
#9116=ORIENTED_EDGE ( 'NONE', *, *, #6087, .F. ) ;
#9123=ORIENTED_EDGE ( 'NONE', *, *, #20963, .F. ) ;
#9124=DIRECTION ( 'NONE',  ( 1.000000000000000000, 2.698458740408365879E-16, -1.110223024625156540E-16 ) ) ;
#9125=ADVANCED_FACE ( 'NONE', ( #12675 ), #29203, .T. ) ;
#9126=EDGE_CURVE ( 'NONE', #26448, #12138, #8694, .T. ) ;
#9128=FACE_OUTER_BOUND ( 'NONE', #17182, .T. ) ;
#9129=DIRECTION ( 'NONE',  ( -0.8090169943749474513, -2.183098979609982436E-16, -0.5877852522924731371 ) ) ;
#9131=VECTOR ( 'NONE', #17480, 1000.000000000000000 ) ;
#9135=DIRECTION ( 'NONE',  ( -0.8090169943749474513, -2.183098979609982436E-16, 0.5877852522924731371 ) ) ;
#9136=AXIS2_PLACEMENT_3D ( 'NONE', #28143, #7199, #16495 ) ;
#9137=ORIENTED_EDGE ( 'NONE', *, *, #1415, .F. ) ;
#9138=VERTEX_POINT ( 'NONE', #3981 ) ;
#9139=CARTESIAN_POINT ( 'NONE',  ( 159.7287565553228887, -1.999999999999974021, 0.8205080756887930260 ) ) ;
#9144=ORIENTED_EDGE ( 'NONE', *, *, #18559, .T. ) ;
#9147=FACE_OUTER_BOUND ( 'NONE', #18368, .T. ) ;
#9148=FACE_OUTER_BOUND ( 'NONE', #3264, .T. ) ;
#9149=ORIENTED_EDGE ( 'NONE', *, *, #3108, .T. ) ;
#9150=EDGE_LOOP ( 'NONE', ( #29405, #24559, #9159, #28581, #27031 ) ) ;
#9152=ORIENTED_EDGE ( 'NONE', *, *, #6496, .F. ) ;
#9156=VECTOR ( 'NONE', #29456, 1000.000000000000000 ) ;
#9157=CARTESIAN_POINT ( 'NONE',  ( 130.7287565553229172, -4.999999999999982236, -19.55415080639417269 ) ) ;
#9158=DIRECTION ( 'NONE',  ( -0.9510565162951536422, 0.000000000000000000, -0.3090169943749472292 ) ) ;
#9159=ORIENTED_EDGE ( 'NONE', *, *, #27896, .T. ) ;
#9161=ADVANCED_FACE ( 'NONE', ( #20003 ), #3532, .T. ) ;
#9162=EDGE_CURVE ( 'NONE', #20741, #20699, #5969, .T. ) ;
#9165=EDGE_CURVE ( 'NONE', #14471, #19412, #10982, .T. ) ;
#9170=ORIENTED_EDGE ( 'NONE', *, *, #24836, .F. ) ;
#9174=LINE ( 'NONE', #18499, #245 ) ;
#9177=DIRECTION ( 'NONE',  ( -2.698458740408365879E-16, 1.000000000000000000, 0.000000000000000000 ) ) ;
#9178=ORIENTED_EDGE ( 'NONE', *, *, #30125, .F. ) ;
#9180=EDGE_LOOP ( 'NONE', ( #14048, #2657, #23018, #13556 ) ) ;
#9182=ORIENTED_EDGE ( 'NONE', *, *, #12071, .T. ) ;
#9188=AXIS2_PLACEMENT_3D ( 'NONE', #2301, #17590, #3869 ) ;
#9189=ORIENTED_EDGE ( 'NONE', *, *, #13179, .F. ) ;
#9190=DIRECTION ( 'NONE',  ( 1.110223024625156540E-16, 2.995891024602366092E-32, 1.000000000000000000 ) ) ;
#9192=ORIENTED_EDGE ( 'NONE', *, *, #19272, .T. ) ;
#9195=DIRECTION ( 'NONE',  ( -2.698458740408365879E-16, 1.000000000000000000, 0.000000000000000000 ) ) ;
#9196=PLANE ( 'NONE',  #26703 ) ;
#9198=ORIENTED_EDGE ( 'NONE', *, *, #26015, .F. ) ;
#9202=EDGE_CURVE ( 'NONE', #26513, #10566, #24587, .T. ) ;
#9205=ORIENTED_EDGE ( 'NONE', *, *, #27177, .T. ) ;
#9208=DIRECTION ( 'NONE',  ( -2.698458740408365879E-16, 1.000000000000000000, 0.000000000000000000 ) ) ;
#9210=LINE ( 'NONE', #25413, #30081 ) ;
#9211=CARTESIAN_POINT ( 'NONE',  ( 143.6922820468854241, -4.999999999999979572, -9.266330736598359152 ) ) ;
#9217=LINE ( 'NONE', #6960, #7401 ) ;
#9218=DIRECTION ( 'NONE',  ( -2.698458740408365879E-16, 1.000000000000000000, 0.000000000000000000 ) ) ;
#9219=LINE ( 'NONE', #11370, #4661 ) ;
#9222=LINE ( 'NONE', #6661, #11004 ) ;
#9224=ORIENTED_EDGE ( 'NONE', *, *, #21340, .T. ) ;
#9226=DIRECTION ( 'NONE',  ( -2.698458740408365879E-16, 1.000000000000000000, 0.000000000000000000 ) ) ;
#9227=LINE ( 'NONE', #12134, #13699 ) ;
#9229=VECTOR ( 'NONE', #27515, 1000.000000000000000 ) ;
#9235=EDGE_CURVE ( 'NONE', #27415, #4938, #22750, .T. ) ;
#9236=EDGE_CURVE ( 'NONE', #12198, #4960, #18157, .T. ) ;
#9237=DIRECTION ( 'NONE',  ( -2.908569913943825554E-16, 1.000000000000000000, -6.826925868028084042E-18 ) ) ;
#9240=VERTEX_POINT ( 'NONE', #20701 ) ;
#9241=ORIENTED_EDGE ( 'NONE', *, *, #776, .F. ) ;
#9242=DIRECTION ( 'NONE',  ( 0.3090169943749475623, 8.338696094058001131E-17, 0.9510565162951536422 ) ) ;
#9245=LINE ( 'NONE', #28529, #14571 ) ;
#9246=ORIENTED_EDGE ( 'NONE', *, *, #19448, .F. ) ;
#9247=ORIENTED_EDGE ( 'NONE', *, *, #19611, .T. ) ;
#9248=LINE ( 'NONE', #7131, #15797 ) ;
#9250=ORIENTED_EDGE ( 'NONE', *, *, #14575, .F. ) ;
#9253=ORIENTED_EDGE ( 'NONE', *, *, #28189, .T. ) ;
#9254=DIRECTION ( 'NONE',  ( 0.5877852522924731371, 1.586114251531760728E-16, -0.8090169943749474513 ) ) ;
#9255=DIRECTION ( 'NONE',  ( -0.8090169943749474513, -2.183098979609982436E-16, 0.5877852522924731371 ) ) ;
#9258=PLANE ( 'NONE',  #352 ) ;
#9259=AXIS2_PLACEMENT_3D ( 'NONE', #17604, #28652, #5421 ) ;
#9260=ORIENTED_EDGE ( 'NONE', *, *, #17743, .F. ) ;
#9262=DIRECTION ( 'NONE',  ( 0.3090169943749472292, 8.338696094057992503E-17, -0.9510565162951536422 ) ) ;
#9263=CARTESIAN_POINT ( 'NONE',  ( 141.1922820468854241, -4.999999999999980460, -2.083034168790677043 ) ) ;
#9265=ORIENTED_EDGE ( 'NONE', *, *, #11070, .F. ) ;
#9266=CARTESIAN_POINT ( 'NONE',  ( 148.6922820468853956, -4.999999999999977796, -6.413161187712876909 ) ) ;
#9269=AXIS2_PLACEMENT_3D ( 'NONE', #9361, #20405, #13249 ) ;
#9273=PLANE ( 'NONE',  #14045 ) ;
#9275=EDGE_CURVE ( 'NONE', #17847, #6680, #6843, .T. ) ;
#9276=LINE ( 'NONE', #599, #19592 ) ;
#9277=EDGE_CURVE ( 'NONE', #10473, #17748, #8661, .T. ) ;
#9280=ORIENTED_EDGE ( 'NONE', *, *, #15028, .F. ) ;
#9281=( LENGTH_UNIT ( ) NAMED_UNIT ( * ) SI_UNIT ( .MILLI., .METRE. ) );
#9282=AXIS2_PLACEMENT_3D ( 'NONE', #28247, #7299, #18741 ) ;
#9283=FACE_OUTER_BOUND ( 'NONE', #17971, .T. ) ;
#9285=VECTOR ( 'NONE', #6216, 1000.000000000000000 ) ;
#9286=CARTESIAN_POINT ( 'NONE',  ( 7.340088617936617155, -5.000000000000015987, 22.59046990083097484 ) ) ;
#9287=CARTESIAN_POINT ( 'NONE',  ( 173.6922820468852535, -9.999999999999996447, 2.247092850131519715 ) ) ;
#9290=COLOUR_RGB ( '', 0.40784314, 0.44705882, 0.49803922) ;
#9294=VERTEX_POINT ( 'NONE', #13697 ) ;
#9295=CARTESIAN_POINT ( 'NONE',  ( 134.5152310637605524, -10.00000000000000533, -30.37205893520530964 ) ) ;
#9300=ORIENTED_EDGE ( 'NONE', *, *, #5852, .F. ) ;
#9301=EDGE_CURVE ( 'NONE', #17531, #27161, #27926, .T. ) ;
#9302=ORIENTED_EDGE ( 'NONE', *, *, #1417, .F. ) ;
#9304=CARTESIAN_POINT ( 'NONE',  ( 129.5152310637605808, -10.00000000000000888, -28.60870317832789311 ) ) ;
#9307=LINE ( 'NONE', #8345, #27864 ) ;
#9308=DIRECTION ( 'NONE',  ( -2.698458740408365879E-16, 1.000000000000000000, 0.000000000000000000 ) ) ;
#9309=VERTEX_POINT ( 'NONE', #6690 ) ;
#9313=VECTOR ( 'NONE', #28048, 1000.000000000000000 ) ;
#9314=VECTOR ( 'NONE', #21742, 1000.000000000000000 ) ;
#9316=VECTOR ( 'NONE', #20799, 1000.000000000000000 ) ;
#9318=CARTESIAN_POINT ( 'NONE',  ( 152.0152310637604955, -1.999999999999976241, -15.61832212156129351 ) ) ;
#9319=DIRECTION ( 'NONE',  ( 6.938893903907227392E-16, -0.000000000000000000, 1.000000000000000000 ) ) ;
#9320=ORIENTED_EDGE ( 'NONE', *, *, #2413, .F. ) ;
#9325=FACE_BOUND ( 'NONE', #24721, .T. ) ;
#9327=DIRECTION ( 'NONE',  ( -0.8090169943749474513, -2.183098979609982436E-16, -0.5877852522924731371 ) ) ;
#9328=LINE ( 'NONE', #29873, #19719 ) ;
#9330=CARTESIAN_POINT ( 'NONE',  ( 159.7287565553230024, -9.999999999999998224, -33.82050807568879947 ) ) ;
#9332=ADVANCED_FACE ( 'NONE', ( #18427 ), #17965, .T. ) ;
#9336=EDGE_CURVE ( 'NONE', #722, #756, #29644, .T. ) ;
#9340=DIRECTION ( 'NONE',  ( -0.9510565162951536422, -2.566386769018988323E-16, 0.3090169943749475623 ) ) ;
#9341=EDGE_CURVE ( 'NONE', #11366, #6539, #16131, .T. ) ;
#9343=EDGE_LOOP ( 'NONE', ( #24837, #2687, #9549, #9114, #26888 ) ) ;
#9344=FACE_OUTER_BOUND ( 'NONE', #591, .T. ) ;
#9346=ORIENTED_EDGE ( 'NONE', *, *, #17248, .T. ) ;
#9349=PLANE ( 'NONE',  #17402 ) ;
#9350=VECTOR ( 'NONE', #1544, 999.9999999999998863 ) ;
#9352=ORIENTED_EDGE ( 'NONE', *, *, #6530, .T. ) ;
#9356=ORIENTED_EDGE ( 'NONE', *, *, #17873, .T. ) ;
#9358=VECTOR ( 'NONE', #15562, 1000.000000000000000 ) ;
#9359=DIRECTION ( 'NONE',  ( -0.5877852522924731371, -1.586114251531760235E-16, 0.8090169943749474513 ) ) ;
#9361=CARTESIAN_POINT ( 'NONE',  ( 162.0152310637604103, -9.999999999999998224, -0.06116980274991495881 ) ) ;
#9362=DIRECTION ( 'NONE',  ( 0.3090169943749472292, 8.338696094057992503E-17, -0.9510565162951536422 ) ) ;
#9363=VECTOR ( 'NONE', #23640, 999.9999999999998863 ) ;
#9367=EDGE_CURVE ( 'NONE', #10926, #13095, #20557, .T. ) ;
#9369=VERTEX_POINT ( 'NONE', #13543 ) ;
#9371=ADVANCED_FACE ( 'NONE', ( #2421 ), #11104, .T. ) ;
#9372=EDGE_CURVE ( 'NONE', #24060, #18723, #27481, .T. ) ;
#9373=LINE ( 'NONE', #25885, #3949 ) ;
#9374=DIRECTION ( 'NONE',  ( 0.5877852522924731371, 1.586114251531760728E-16, 0.8090169943749474513 ) ) ;
#9375=EDGE_CURVE ( 'NONE', #209, #13070, #30238, .T. ) ;
#9377=ORIENTED_EDGE ( 'NONE', *, *, #2071, .T. ) ;
#9378=ORIENTED_EDGE ( 'NONE', *, *, #19996, .F. ) ;
#9379=LINE ( 'NONE', #7106, #25158 ) ;
#9382=DIRECTION ( 'NONE',  ( -0.5877852522924731371, -1.586114251531760728E-16, -0.8090169943749474513 ) ) ;
#9383=DIRECTION ( 'NONE',  ( 0.000000000000000000, 0.000000000000000000, -1.000000000000000000 ) ) ;
#9388=VERTEX_POINT ( 'NONE', #25013 ) ;
#9394=ORIENTED_EDGE ( 'NONE', *, *, #16549, .F. ) ;
#9395=LINE ( 'NONE', #28834, #22575 ) ;
#9396=DIRECTION ( 'NONE',  ( -1.110223024625156540E-16, 0.000000000000000000, -1.000000000000000000 ) ) ;
#9397=EDGE_LOOP ( 'NONE', ( #9944, #6416, #13489, #16046 ) ) ;
#9399=DIRECTION ( 'NONE',  ( -0.5877852522924731371, -1.586114251531760235E-16, 0.8090169943749474513 ) ) ;
#9400=CARTESIAN_POINT ( 'NONE',  ( 133.6922820468854241, -1.999999999999981348, -17.92658477444275533 ) ) ;
#9403=EDGE_LOOP ( 'NONE', ( #18925, #14830, #12314, #18836 ) ) ;
#9404=EDGE_CURVE ( 'NONE', #28119, #8559, #27339, .T. ) ;
#9405=VECTOR ( 'NONE', #3134, 1000.000000000000000 ) ;
#9406=CARTESIAN_POINT ( 'NONE',  ( 146.1922820468854241, -10.00000000000000355, -10.74328820663507678 ) ) ;
#9409=EDGE_CURVE ( 'NONE', #12138, #29920, #22867, .T. ) ;
#9411=CARTESIAN_POINT ( 'NONE',  ( 102.8198706071908219, -4.999999999999989342, 74.70300872013253013 ) ) ;
#9412=EDGE_CURVE ( 'NONE', #4141, #28792, #1976, .T. ) ;
#9413=LINE ( 'NONE', #18738, #8059 ) ;
#9414=ORIENTED_EDGE ( 'NONE', *, *, #13525, .T. ) ;
#9415=DIRECTION ( 'NONE',  ( -0.9510565162951536422, 0.000000000000000000, -0.3090169943749472292 ) ) ;
#9416=CARTESIAN_POINT ( 'NONE',  ( 5.828767459767482784, -5.000000000000015987, 17.93910165294919423 ) ) ;
#9417=CARTESIAN_POINT ( 'NONE',  ( 169.7287565553228603, -9.999999999999998224, 0.8205080756887930260 ) ) ;
#9418=ORIENTED_EDGE ( 'NONE', *, *, #6299, .F. ) ;
#9422=DIRECTION ( 'NONE',  ( 0.5877852522924731371, 1.586114251531760728E-16, 0.8090169943749474513 ) ) ;
#9423=DIRECTION ( 'NONE',  ( -2.698458740408365879E-16, 1.000000000000000000, 0.000000000000000000 ) ) ;
#9424=CARTESIAN_POINT ( 'NONE',  ( 164.5152310637604671, -1.999999999999971800, -21.71180489736091346 ) ) ;
#9426=VECTOR ( 'NONE', #27777, 1000.000000000000000 ) ;
#9427=ORIENTED_EDGE ( 'NONE', *, *, #22591, .F. ) ;
#9428=LINE ( 'NONE', #20885, #27179 ) ;
#9430=CARTESIAN_POINT ( 'NONE',  ( 132.0152310637605808, -10.00000000000000711, -6.958068083716893781 ) ) ;
#9432=DIRECTION ( 'NONE',  ( -0.8090169943749474513, -2.183098979609982436E-16, -0.5877852522924731371 ) ) ;
#9433=LINE ( 'NONE', #12033, #24581 ) ;
#9437=ORIENTED_EDGE ( 'NONE', *, *, #29953, .F. ) ;
#9440=ADVANCED_FACE ( 'NONE', ( #7580 ), #21312, .T. ) ;
#9441=LINE ( 'NONE', #12337, #13422 ) ;
#9443=EDGE_CURVE ( 'NONE', #18076, #14, #421, .T. ) ;
#9446=EDGE_CURVE ( 'NONE', #506, #29222, #28385, .T. ) ;
#9447=ORIENTED_EDGE ( 'NONE', *, *, #6440, .T. ) ;
#9448=VERTEX_POINT ( 'NONE', #19321 ) ;
#9450=DIRECTION ( 'NONE',  ( -2.698458740408365879E-16, 1.000000000000000000, 0.000000000000000000 ) ) ;
#9451=VECTOR ( 'NONE', #3910, 1000.000000000000000 ) ;
#9453=CARTESIAN_POINT ( 'NONE',  ( 158.6922820468854241, -1.999999999999973133, -35.24709285013155835 ) ) ;
#9454=DIRECTION ( 'NONE',  ( 0.3090169943749472292, 8.338696094057992503E-17, -0.9510565162951536422 ) ) ;
#9457=ORIENTED_EDGE ( 'NONE', *, *, #13723, .F. ) ;
#9459=EDGE_LOOP ( 'NONE', ( #10365, #28747, #3260, #28190 ) ) ;
#9463=EDGE_LOOP ( 'NONE', ( #7479, #12848, #7043, #191 ) ) ;
#9464=DIRECTION ( 'NONE',  ( -0.9510565162951536422, -2.566386769018988323E-16, 0.3090169943749475623 ) ) ;
#9465=EDGE_LOOP ( 'NONE', ( #27291, #10968, #2837, #19161 ) ) ;
#9471=ORIENTED_EDGE ( 'NONE', *, *, #22631, .F. ) ;
#9472=EDGE_CURVE ( 'NONE', #12367, #14559, #16588, .T. ) ;
#9473=FACE_BOUND ( 'NONE', #26107, .T. ) ;
#9474=AXIS2_PLACEMENT_3D ( 'NONE', #13461, #6460, #25230 ) ;
#9475=ORIENTED_EDGE ( 'NONE', *, *, #29614, .T. ) ;
#9476=PLANE ( 'NONE',  #7688 ) ;
#9477=DIRECTION ( 'NONE',  ( -0.5877852522924731371, -1.586114251531760728E-16, -0.8090169943749474513 ) ) ;
#9478=FACE_OUTER_BOUND ( 'NONE', #17350, .T. ) ;
#9480=CARTESIAN_POINT ( 'NONE',  ( 141.1922820468854525, -1.999999999999978684, -13.59645775552055902 ) ) ;
#9481=ORIENTED_EDGE ( 'NONE', *, *, #12330, .F. ) ;
#9487=LINE ( 'NONE', #4480, #29319 ) ;
#9488=CARTESIAN_POINT ( 'NONE',  ( 168.6922820468852819, -9.999999999999998224, -0.6060766987539614181 ) ) ;
#9490=CARTESIAN_POINT ( 'NONE',  ( 133.7287565553229456, -1.999999999999980904, 6.499999999999978684 ) ) ;
#9492=ORIENTED_EDGE ( 'NONE', *, *, #19270, .T. ) ;
#9495=ORIENTED_EDGE ( 'NONE', *, *, #28451, .F. ) ;
#9496=VECTOR ( 'NONE', #19101, 1000.000000000000000 ) ;
#9497=FACE_OUTER_BOUND ( 'NONE', #4644, .T. ) ;
#9500=DIRECTION ( 'NONE',  ( -0.5877852522924731371, -1.586114251531760235E-16, 0.8090169943749474513 ) ) ;
#9504=ORIENTED_EDGE ( 'NONE', *, *, #23247, .F. ) ;
#9505=EDGE_CURVE ( 'NONE', #5460, #7125, #14135, .T. ) ;
#9506=CARTESIAN_POINT ( 'NONE',  ( 162.0152310637604955, -1.999999999999972689, -15.61832212156129707 ) ) ;
#9508=LINE ( 'NONE', #14387, #3598 ) ;
#9510=CARTESIAN_POINT ( 'NONE',  ( 157.2287565553229740, -1.999999999999973577, -20.83012701892220520 ) ) ;
#9512=LINE ( 'NONE', #16395, #12373 ) ;
#9513=ORIENTED_EDGE ( 'NONE', *, *, #446, .T. ) ;
#9514=AXIS2_PLACEMENT_3D ( 'NONE', #8334, #19931, #6050 ) ;
#9519=ORIENTED_EDGE ( 'NONE', *, *, #28738, .F. ) ;
#9520=CARTESIAN_POINT ( 'NONE',  ( 137.0152310637605808, -10.00000000000000533, -34.70218595412750773 ) ) ;
#9522=LINE ( 'NONE', #22989, #29869 ) ;
#9523=LINE ( 'NONE', #16404, #24652 ) ;
#9525=ORIENTED_EDGE ( 'NONE', *, *, #8038, .F. ) ;
#9526=CARTESIAN_POINT ( 'NONE',  ( 172.7287565553229456, -3.999999999999989786, 8.500000000000007105 ) ) ;
#9528=VECTOR ( 'NONE', #4514, 1000.000000000000000 ) ;
#9529=ORIENTED_EDGE ( 'NONE', *, *, #439, .F. ) ;
#9530=CARTESIAN_POINT ( 'NONE',  ( 13.06098793629887744, -5.000000000000014211, -40.19758755079165979 ) ) ;
#9531=LINE ( 'NONE', #9845, #27408 ) ;
#9532=VECTOR ( 'NONE', #8822, 1000.000000000000000 ) ;
#9541=ORIENTED_EDGE ( 'NONE', *, *, #178, .F. ) ;
#9543=ADVANCED_FACE ( 'NONE', ( #5139 ), #5449, .T. ) ;
#9544=EDGE_CURVE ( 'NONE', #25774, #26592, #2573, .T. ) ;
#9545=ORIENTED_EDGE ( 'NONE', *, *, #4318, .T. ) ;
#9546=ADVANCED_FACE ( 'NONE', ( #119 ), #4836, .T. ) ;
#9547=CARTESIAN_POINT ( 'NONE',  ( 152.0152310637604671, -1.999999999999976241, -0.06116980274991495881 ) ) ;
#9549=ORIENTED_EDGE ( 'NONE', *, *, #23991, .T. ) ;
#9550=ORIENTED_EDGE ( 'NONE', *, *, #10230, .T. ) ;
#9551=DIRECTION ( 'NONE',  ( -0.9510565162951536422, -2.566386769018988816E-16, -0.3090169943749472292 ) ) ;
#9555=AXIS2_PLACEMENT_3D ( 'NONE', #8112, #5387, #5837 ) ;
#9559=DIRECTION ( 'NONE',  ( -2.698458740408365879E-16, 1.000000000000000000, 0.000000000000000000 ) ) ;
#9560=DIRECTION ( 'NONE',  ( -0.5877852522924731371, -1.586114251531760728E-16, -0.8090169943749474513 ) ) ;
#9563=CARTESIAN_POINT ( 'NONE',  ( 142.0152310637605524, -10.00000000000000533, 1.702185954127501066 ) ) ;
#9567=ORIENTED_EDGE ( 'NONE', *, *, #23379, .T. ) ;
#9568=ORIENTED_EDGE ( 'NONE', *, *, #30190, .F. ) ;
#9569=CARTESIAN_POINT ( 'NONE',  ( 178.7287565553229172, -1.999999999999968914, 0.5000000000000029976 ) ) ;
#9570=ORIENTED_EDGE ( 'NONE', *, *, #21341, .F. ) ;
#9572=EDGE_CURVE ( 'NONE', #3020, #6774, #9862, .T. ) ;
#9575=VECTOR ( 'NONE', #8012, 1000.000000000000000 ) ;
#9577=DIRECTION ( 'NONE',  ( -0.5877852522924731371, -1.586114251531760728E-16, -0.8090169943749474513 ) ) ;
#9579=AXIS2_PLACEMENT_3D ( 'NONE', #12349, #8224, #17092 ) ;
#9581=EDGE_CURVE ( 'NONE', #23543, #24609, #11698, .T. ) ;
#9582=VECTOR ( 'NONE', #24082, 1000.000000000000000 ) ;
#9584=ADVANCED_FACE ( 'NONE', ( #14582 ), #23932, .T. ) ;
#9585=( NAMED_UNIT ( * ) PLANE_ANGLE_UNIT ( ) SI_UNIT ( $, .RADIAN. ) );
#9587=PLANE ( 'NONE',  #29928 ) ;
#9588=VECTOR ( 'NONE', #6605, 1000.000000000000000 ) ;
#9589=LINE ( 'NONE', #18909, #18460 ) ;
#9590=DIRECTION ( 'NONE',  ( -0.9510565162951536422, 0.000000000000000000, -0.3090169943749472292 ) ) ;
#9591=CARTESIAN_POINT ( 'NONE',  ( 129.5152310637605524, -10.00000000000000888, -21.71180489736090991 ) ) ;
#9593=CARTESIAN_POINT ( 'NONE',  ( 136.1922820468854241, -10.00000000000000533, -30.91696583120935671 ) ) ;
#9595=VERTEX_POINT ( 'NONE', #21157 ) ;
#9597=ORIENTED_EDGE ( 'NONE', *, *, #13188, .T. ) ;
#9602=LINE ( 'NONE', #165, #5353 ) ;
#9603=EDGE_LOOP ( 'NONE', ( #12610, #22341, #3262, #16109 ) ) ;
#9605=ORIENTED_EDGE ( 'NONE', *, *, #6342, .T. ) ;
#9606=AXIS2_PLACEMENT_3D ( 'NONE', #27283, #11486, #25400 ) ;
#9608=DIRECTION ( 'NONE',  ( 1.110223024625156540E-16, 2.995891024602366092E-32, 1.000000000000000000 ) ) ;
#9610=LINE ( 'NONE', #25958, #1369 ) ;
#9611=ORIENTED_EDGE ( 'NONE', *, *, #20200, .T. ) ;
#9612=DIRECTION ( 'NONE',  ( 1.000000000000000000, 2.698458740408365879E-16, -1.110223024625156540E-16 ) ) ;
#9616=ORIENTED_EDGE ( 'NONE', *, *, #12212, .T. ) ;
#9617=CIRCLE ( 'NONE', #13519, 8.000000000000003553 ) ;
#9621=FACE_OUTER_BOUND ( 'NONE', #19024, .T. ) ;
#9622=ORIENTED_EDGE ( 'NONE', *, *, #21169, .T. ) ;
#9627=AXIS2_PLACEMENT_3D ( 'NONE', #6097, #27040, #27353 ) ;
#9629=EDGE_CURVE ( 'NONE', #18781, #21937, #8024, .T. ) ;
#9630=ORIENTED_EDGE ( 'NONE', *, *, #5882, .F. ) ;
#9631=FACE_BOUND ( 'NONE', #21607, .T. ) ;
#9633=ORIENTED_EDGE ( 'NONE', *, *, #28618, .F. ) ;
#9634=FACE_OUTER_BOUND ( 'NONE', #2275, .T. ) ;
#9635=CARTESIAN_POINT ( 'NONE',  ( 144.7287565553230309, -4.999999999999978684, -16.50000000000000000 ) ) ;
#9636=LINE ( 'NONE', #18954, #28768 ) ;
#9637=LINE ( 'NONE', #12078, #13900 ) ;
#9639=DIRECTION ( 'NONE',  ( -2.698458740408365879E-16, 1.000000000000000000, 0.000000000000000000 ) ) ;
#9641=VERTEX_POINT ( 'NONE', #5598 ) ;
#9643=ORIENTED_EDGE ( 'NONE', *, *, #6407, .T. ) ;
#9646=LINE ( 'NONE', #9032, #10742 ) ;
#9649=ORIENTED_EDGE ( 'NONE', *, *, #22874, .F. ) ;
#9650=LINE ( 'NONE', #23707, #2295 ) ;
#9652=ORIENTED_EDGE ( 'NONE', *, *, #16870, .T. ) ;
#9656=PLANE ( 'NONE',  #3792 ) ;
#9659=ORIENTED_EDGE ( 'NONE', *, *, #10939, .F. ) ;
#9660=DIRECTION ( 'NONE',  ( 0.000000000000000000, -1.000000000000000000, 0.000000000000000000 ) ) ;
#9664=VERTEX_POINT ( 'NONE', #12905 ) ;
#9665=EDGE_CURVE ( 'NONE', #3010, #28897, #19929, .T. ) ;
#9667=DIRECTION ( 'NONE',  ( -0.8090169943749474513, -2.183098979609982436E-16, 0.5877852522924731371 ) ) ;
#9668=CARTESIAN_POINT ( 'NONE',  ( 159.7287565553229456, -10.00000000000000000, -16.50000000000000355 ) ) ;
#9669=CARTESIAN_POINT ( 'NONE',  ( 3.441479889454326813, -5.000000000000016875, 10.59178599929328435 ) ) ;
#9670=VECTOR ( 'NONE', #19431, 1000.000000000000000 ) ;
#9671=DIRECTION ( 'NONE',  ( 1.110223024625156540E-16, 2.995891024602366092E-32, 1.000000000000000000 ) ) ;
#9677=VECTOR ( 'NONE', #25418, 1000.000000000000000 ) ;
#9679=LINE ( 'NONE', #5112, #12741 ) ;
#9682=FACE_OUTER_BOUND ( 'NONE', #26728, .T. ) ;
#9684=EDGE_CURVE ( 'NONE', #8715, #15699, #12753, .T. ) ;
#9685=DIRECTION ( 'NONE',  ( 1.110223024625156540E-16, 2.995891024602366092E-32, 1.000000000000000000 ) ) ;
#9689=ORIENTED_EDGE ( 'NONE', *, *, #11078, .F. ) ;
#9691=ORIENTED_EDGE ( 'NONE', *, *, #17850, .T. ) ;
#9693=VECTOR ( 'NONE', #28456, 1000.000000000000000 ) ;
#9698=ORIENTED_EDGE ( 'NONE', *, *, #16448, .F. ) ;
#9700=ORIENTED_EDGE ( 'NONE', *, *, #3782, .T. ) ;
#9702=CARTESIAN_POINT ( 'NONE',  ( 144.7287565553229740, -10.00000000000000533, 0.8205080756887930260 ) ) ;
#9705=VECTOR ( 'NONE', #16781, 1000.000000000000000 ) ;
#9707=VERTEX_POINT ( 'NONE', #17486 ) ;
#9708=CARTESIAN_POINT ( 'NONE',  ( 142.2287565553230024, -1.999999999999978462, -3.509618943233403510 ) ) ;
#9711=CARTESIAN_POINT ( 'NONE',  ( 171.1922820468853388, -9.999999999999996447, -19.40354224447947828 ) ) ;
#9712=VECTOR ( 'NONE', #18423, 1000.000000000000000 ) ;
#9713=CARTESIAN_POINT ( 'NONE',  ( 152.2287565553230024, -4.999999999999976907, -20.83012701892220164 ) ) ;
#9714=EDGE_CURVE ( 'NONE', #10404, #28006, #29295, .T. ) ;
#9715=EDGE_CURVE ( 'NONE', #20837, #6555, #7883, .T. ) ;
#9716=ORIENTED_EDGE ( 'NONE', *, *, #13141, .T. ) ;
#9728=LINE ( 'NONE', #7459, #415 ) ;
#9731=CARTESIAN_POINT ( 'NONE',  ( 172.7287565553229740, -84.33034373659253902, -41.50000000000000711 ) ) ;
#9732=VECTOR ( 'NONE', #5913, 1000.000000000000000 ) ;
#9735=VECTOR ( 'NONE', #14726, 1000.000000000000000 ) ;
#9736=CARTESIAN_POINT ( 'NONE',  ( 138.6922820468854241, -4.999999999999979572, 2.247092850131519715 ) ) ;
#9738=CARTESIAN_POINT ( 'NONE',  ( 133.7287565553229456, -4.999999999999981348, 0.5000000000000029976 ) ) ;
#9743=LINE ( 'NONE', #9593, #19923 ) ;
#9749=DIRECTION ( 'NONE',  ( -2.698458740408365879E-16, 1.000000000000000000, 0.000000000000000000 ) ) ;
#9752=LINE ( 'NONE', #18923, #25830 ) ;
#9753=EDGE_LOOP ( 'NONE', ( #9936, #10521, #866, #13465 ) ) ;
#9755=EDGE_LOOP ( 'NONE', ( #20413, #14237, #6797, #12350 ) ) ;
#9758=EDGE_CURVE ( 'NONE', #18859, #27873, #18046, .T. ) ;
#9760=CARTESIAN_POINT ( 'NONE',  ( 154.5152310637605240, -1.999999999999974465, -21.71180489736091346 ) ) ;
#9761=EDGE_CURVE ( 'NONE', #4670, #7383, #29875, .T. ) ;
#9762=ORIENTED_EDGE ( 'NONE', *, *, #1346, .T. ) ;
#9764=PLANE ( 'NONE',  #18852 ) ;
#9765=VERTEX_POINT ( 'NONE', #30014 ) ;
#9767=ORIENTED_EDGE ( 'NONE', *, *, #23378, .F. ) ;
#9771=ORIENTED_EDGE ( 'NONE', *, *, #21304, .F. ) ;
#9772=FACE_OUTER_BOUND ( 'NONE', #26090, .T. ) ;
#9773=PLANE ( 'NONE',  #22534 ) ;
#9774=VECTOR ( 'NONE', #17943, 1000.000000000000000 ) ;
#9778=AXIS2_PLACEMENT_3D ( 'NONE', #24910, #4144, #13438 ) ;
#9780=VERTEX_POINT ( 'NONE', #27412 ) ;
#9781=LINE ( 'NONE', #25669, #12304 ) ;
#9783=LINE ( 'NONE', #26136, #10118 ) ;
#9785=CARTESIAN_POINT ( 'NONE',  ( 156.1922820468853956, -1.999999999999974021, -19.40354224447947828 ) ) ;
#9787=DIRECTION ( 'NONE',  ( 0.5877852522924731371, 0.000000000000000000, 0.8090169943749474513 ) ) ;
#9788=AXIS2_PLACEMENT_3D ( 'NONE', #12451, #21777, #877 ) ;
#9789=ORIENTED_EDGE ( 'NONE', *, *, #14273, .F. ) ;
#9790=CARTESIAN_POINT ( 'NONE',  ( 133.7287565553229172, -4.999999999999981348, -33.50000000000000000 ) ) ;
#9792=VECTOR ( 'NONE', #27465, 1000.000000000000000 ) ;
#9794=EDGE_LOOP ( 'NONE', ( #27437, #550, #22712, #4411 ) ) ;
#9796=EDGE_CURVE ( 'NONE', #2176, #26572, #23093, .T. ) ;
#9799=LINE ( 'NONE', #28469, #30156 ) ;
#9801=PLANE ( 'NONE',  #3441 ) ;
#9802=ORIENTED_EDGE ( 'NONE', *, *, #15030, .F. ) ;
#9803=DIRECTION ( 'NONE',  ( -0.9510565162951536422, -2.566386769018988816E-16, -0.3090169943749472292 ) ) ;
#9809=LINE ( 'NONE', #19121, #17875 ) ;
#9813=CARTESIAN_POINT ( 'NONE',  ( 133.6922820468854241, -1.999999999999980904, -23.73366926340167282 ) ) ;
#9818=EDGE_LOOP ( 'NONE', ( #27619, #11108, #26658, #9475, #19560 ) ) ;
#9819=ORIENTED_EDGE ( 'NONE', *, *, #28806, .F. ) ;
#9820=LINE ( 'NONE', #228, #16081 ) ;
#9824=DIRECTION ( 'NONE',  ( -2.698458740408366372E-16, 1.000000000000000000, 0.000000000000000000 ) ) ;
#9825=LINE ( 'NONE', #5412, #11912 ) ;
#9826=ORIENTED_EDGE ( 'NONE', *, *, #5718, .F. ) ;
#9831=EDGE_LOOP ( 'NONE', ( #8721, #9109, #863, #25083, #17060, #12203 ) ) ;
#9835=AXIS2_PLACEMENT_3D ( 'NONE', #11565, #21184, #14458 ) ;
#9837=CARTESIAN_POINT ( 'NONE',  ( 16.64003638268102137, -5.000000000000013323, -51.21276603297467034 ) ) ;
#9838=EDGE_CURVE ( 'NONE', #10764, #17796, #15458, .T. ) ;
#9840=VERTEX_POINT ( 'NONE', #25232 ) ;
#9841=PLANE ( 'NONE',  #21243 ) ;
#9842=EDGE_CURVE ( 'NONE', #26897, #4109, #24942, .T. ) ;
#9844=CARTESIAN_POINT ( 'NONE',  ( 167.0152310637604387, -1.999999999999971800, -8.721423840594312082 ) ) ;
#9845=CARTESIAN_POINT ( 'NONE',  ( 138.6922820468854525, -1.999999999999979128, -23.73366926340167282 ) ) ;
#9848=VERTEX_POINT ( 'NONE', #4168 ) ;
#9851=VECTOR ( 'NONE', #6911, 1000.000000000000000 ) ;
#9856=VERTEX_POINT ( 'NONE', #24787 ) ;
#9857=FACE_OUTER_BOUND ( 'NONE', #29013, .T. ) ;
#9858=EDGE_CURVE ( 'NONE', #10985, #28338, #13172, .T. ) ;
#9861=PLANE ( 'NONE',  #18238 ) ;
#9862=LINE ( 'NONE', #19174, #27833 ) ;
#9866=CARTESIAN_POINT ( 'NONE',  ( 11.47554319436263448, -5.000000000000014211, 35.31809036943338498 ) ) ;
#9867=LINE ( 'NONE', #19180, #26092 ) ;
#9870=DIRECTION ( 'NONE',  ( -0.5877852522924731371, -1.586114251531760728E-16, -0.8090169943749474513 ) ) ;
#9871=DIRECTION ( 'NONE',  ( 1.110223024625156540E-16, 2.995891024602366092E-32, 1.000000000000000000 ) ) ;
#9874=CARTESIAN_POINT ( 'NONE',  ( 174.5152310637604387, -4.999999999999970690, -21.71180489736091346 ) ) ;
#9875=VECTOR ( 'NONE', #8051, 1000.000000000000000 ) ;
#9876=EDGE_LOOP ( 'NONE', ( #3655, #11946, #6708, #17237 ) ) ;
#9877=VERTEX_POINT ( 'NONE', #5220 ) ;
#9881=PLANE ( 'NONE',  #15991 ) ;
#9882=CARTESIAN_POINT ( 'NONE',  ( 151.1922820468853672, -4.999999999999976907, -2.083034168790677043 ) ) ;
#9884=VECTOR ( 'NONE', #13284, 1000.000000000000000 ) ;
#9885=ORIENTED_EDGE ( 'NONE', *, *, #21642, .F. ) ;
#9886=CARTESIAN_POINT ( 'NONE',  ( 143.6922820468854525, -1.999999999999978462, -23.73366926340167282 ) ) ;
#9887=EDGE_CURVE ( 'NONE', #25944, #19638, #16357, .T. ) ;
#9888=CARTESIAN_POINT ( 'NONE',  ( 178.7287565553229172, -1.999999999999968914, 0.5000000000000029976 ) ) ;
#9889=CARTESIAN_POINT ( 'NONE',  ( 131.1922820468854241, -1.999999999999981792, -2.083034168790673490 ) ) ;
#9890=EDGE_CURVE ( 'NONE', #18400, #29149, #30169, .T. ) ;
#9891=CARTESIAN_POINT ( 'NONE',  ( 136.1922820468854241, -1.999999999999980460, -30.91696583120935671 ) ) ;
#9892=LINE ( 'NONE', #1068, #10417 ) ;
#9893=VECTOR ( 'NONE', #2864, 1000.000000000000000 ) ;
#9895=CARTESIAN_POINT ( 'NONE',  ( 88.14846424109262557, -4.999999999999993783, 64.04360804951359398 ) ) ;
#9897=VERTEX_POINT ( 'NONE', #14512 ) ;
#9899=CARTESIAN_POINT ( 'NONE',  ( 147.0152310637605808, -10.00000000000000178, -15.61832212156129707 ) ) ;
#9902=DIRECTION ( 'NONE',  ( 2.908569913943825554E-16, -1.000000000000000000, 0.000000000000000000 ) ) ;
#9903=AXIS2_PLACEMENT_3D ( 'NONE', #8668, #26444, #12525 ) ;
#9904=VERTEX_POINT ( 'NONE', #28162 ) ;
#9909=VERTEX_POINT ( 'NONE', #25679 ) ;
#9910=DIRECTION ( 'NONE',  ( -2.698458740408365879E-16, 1.000000000000000000, 0.000000000000000000 ) ) ;
#9911=EDGE_LOOP ( 'NONE', ( #21574, #15273, #7775, #25445 ) ) ;
#9918=ORIENTED_EDGE ( 'NONE', *, *, #16869, .F. ) ;
#9919=VECTOR ( 'NONE', #12112, 1000.000000000000000 ) ;
#9922=SHAPE_DEFINITION_REPRESENTATION ( #26667, #16744 ) ;
#9925=FACE_BOUND ( 'NONE', #27285, .T. ) ;
#9926=EDGE_CURVE ( 'NONE', #19638, #5499, #12080, .T. ) ;
#9927=ADVANCED_FACE ( 'NONE', ( #14356 ), #28005, .T. ) ;
#9928=ADVANCED_FACE ( 'NONE', ( #25989 ), #23541, .T. ) ;
#9930=CARTESIAN_POINT ( 'NONE',  ( 134.7287565553230024, -10.00000000000000711, 0.8205080756887930260 ) ) ;
#9931=FACE_OUTER_BOUND ( 'NONE', #16349, .T. ) ;
#9932=CARTESIAN_POINT ( 'NONE',  ( 147.0152310637605808, -1.999999999999976685, -15.61832212156129707 ) ) ;
#9933=AXIS2_PLACEMENT_3D ( 'NONE', #1211, #19203, #6237 ) ;
#9936=ORIENTED_EDGE ( 'NONE', *, *, #2530, .F. ) ;
#9937=CARTESIAN_POINT ( 'NONE',  ( 161.1922820468853388, -9.999999999999998224, -13.59645775552055902 ) ) ;
#9943=DIRECTION ( 'NONE',  ( -0.9510565162951536422, 0.000000000000000000, -0.3090169943749472292 ) ) ;
#9944=ORIENTED_EDGE ( 'NONE', *, *, #9446, .T. ) ;
#9945=LINE ( 'NONE', #7384, #19323 ) ;
#9950=DIRECTION ( 'NONE',  ( 1.000000000000000000, 2.698458740408365879E-16, -1.110223024625156540E-16 ) ) ;
#9952=ORIENTED_EDGE ( 'NONE', *, *, #11724, .T. ) ;
#9954=VERTEX_POINT ( 'NONE', #354 ) ;
#9957=VECTOR ( 'NONE', #82, 1000.000000000000000 ) ;
#9958=ORIENTED_EDGE ( 'NONE', *, *, #4537, .T. ) ;
#9959=DIRECTION ( 'NONE',  ( -0.9510565162951536422, -2.566386769018988816E-16, -0.3090169943749472292 ) ) ;
#9960=EDGE_LOOP ( 'NONE', ( #8935, #29397, #9144, #1743 ) ) ;
#9961=ORIENTED_EDGE ( 'NONE', *, *, #6783, .F. ) ;
#9962=CARTESIAN_POINT ( 'NONE',  ( 139.5152310637605808, -4.999999999999980460, -1.548930218128858680E-14 ) ) ;
#9963=EDGE_CURVE ( 'NONE', #25406, #17919, #21239, .T. ) ;
#9964=EDGE_CURVE ( 'NONE', #10203, #10847, #7064, .T. ) ;
#9965=EDGE_CURVE ( 'NONE', #2774, #3794, #25840, .T. ) ;
#9966=LINE ( 'NONE', #21723, #2631 ) ;
#9967=VERTEX_POINT ( 'NONE', #18957 ) ;
#9969=DIRECTION ( 'NONE',  ( 1.110223024625156540E-16, 2.995891024602366092E-32, 1.000000000000000000 ) ) ;
#9970=LINE ( 'NONE', #7842, #27762 ) ;
#9971=PLANE ( 'NONE',  #25561 ) ;
#9976=ORIENTED_EDGE ( 'NONE', *, *, #6403, .F. ) ;
#9977=DIRECTION ( 'NONE',  ( 0.9510565162951535312, 2.566386769018988816E-16, -0.3090169943749475623 ) ) ;
#9979=CARTESIAN_POINT ( 'NONE',  ( 176.1922820468853388, -9.999999999999994671, -30.91696583120936026 ) ) ;
#9980=VECTOR ( 'NONE', #1439, 1000.000000000000000 ) ;
#9984=PLANE ( 'NONE',  #4202 ) ;
#9986=FACE_OUTER_BOUND ( 'NONE', #12987, .T. ) ;
#9990=ORIENTED_EDGE ( 'NONE', *, *, #29711, .T. ) ;
#9992=ORIENTED_EDGE ( 'NONE', *, *, #27256, .T. ) ;
#9995=ORIENTED_EDGE ( 'NONE', *, *, #6785, .T. ) ;
#9996=ADVANCED_FACE ( 'NONE', ( #28312 ), #23236, .T. ) ;
#9998=EDGE_CURVE ( 'NONE', #14637, #2694, #28460, .T. ) ;
#9999=DIRECTION ( 'NONE',  ( 0.9510565162951536422, 2.566386769018988816E-16, 0.3090169943749472292 ) ) ;
#10000=ORIENTED_EDGE ( 'NONE', *, *, #5297, .F. ) ;
#10001=EDGE_LOOP ( 'NONE', ( #5306, #16696, #11411, #5001 ) ) ;
#10002=EDGE_CURVE ( 'NONE', #10566, #21077, #49, .T. ) ;
#10005=DIRECTION ( 'NONE',  ( -1.110223024625156540E-16, 0.000000000000000000, -1.000000000000000000 ) ) ;
#10006=CARTESIAN_POINT ( 'NONE',  ( 157.2287565553229456, -10.00000000000000000, -12.16987298107780369 ) ) ;
#10011=DIRECTION ( 'NONE',  ( -2.698458740408365879E-16, 1.000000000000000000, 0.000000000000000000 ) ) ;
#10012=CARTESIAN_POINT ( 'NONE',  ( 142.0152310637605240, -10.00000000000000533, -0.06116980274991495881 ) ) ;
#10015=FACE_OUTER_BOUND ( 'NONE', #6695, .T. ) ;
#10016=EDGE_LOOP ( 'NONE', ( #16225, #12808, #6389, #17265 ) ) ;
#10017=VECTOR ( 'NONE', #847, 999.9999999999998863 ) ;
#10018=DIRECTION ( 'NONE',  ( -0.8090169943749474513, -2.183098979609982436E-16, -0.5877852522924731371 ) ) ;
#10019=CARTESIAN_POINT ( 'NONE',  ( 134.5152310637605524, -1.999999999999980460, -21.71180489736090991 ) ) ;
#10020=DIRECTION ( 'NONE',  ( -2.698458740408365879E-16, 1.000000000000000000, 0.000000000000000000 ) ) ;
#10021=ORIENTED_EDGE ( 'NONE', *, *, #15715, .F. ) ;
#10022=ORIENTED_EDGE ( 'NONE', *, *, #20783, .F. ) ;
#10023=ORIENTED_EDGE ( 'NONE', *, *, #18692, .T. ) ;
#10028=PLANE ( 'NONE',  #4319 ) ;
#10029=LINE ( 'NONE', #28868, #19899 ) ;
#10030=DIRECTION ( 'NONE',  ( -0.5877852522924731371, -1.586114251531760728E-16, -0.8090169943749474513 ) ) ;
#10031=VECTOR ( 'NONE', #27115, 1000.000000000000000 ) ;
#10033=PLANE ( 'NONE',  #19633 ) ;
#10034=EDGE_CURVE ( 'NONE', #18517, #14794, #16667, .T. ) ;
#10035=LINE ( 'NONE', #24098, #14733 ) ;
#10038=DIRECTION ( 'NONE',  ( 0.9510565162951535312, 2.566386769018988816E-16, -0.3090169943749475623 ) ) ;
#10042=CARTESIAN_POINT ( 'NONE',  ( 164.7287565553228887, -1.999999999999972244, -7.839745962155603820 ) ) ;
#10044=ORIENTED_EDGE ( 'NONE', *, *, #29751, .T. ) ;
#10046=DIRECTION ( 'NONE',  ( -0.5877852522924731371, -1.586114251531760235E-16, 0.8090169943749474513 ) ) ;
#10050=ORIENTED_EDGE ( 'NONE', *, *, #22493, .T. ) ;
#10051=ORIENTED_EDGE ( 'NONE', *, *, #5742, .T. ) ;
#10055=AXIS2_PLACEMENT_3D ( 'NONE', #26468, #16836, #16987 ) ;
#10057=DIRECTION ( 'NONE',  ( -2.698458740408365879E-16, 1.000000000000000000, 0.000000000000000000 ) ) ;
#10058=ORIENTED_EDGE ( 'NONE', *, *, #29445, .F. ) ;
#10059=DIRECTION ( 'NONE',  ( -2.698458740408365879E-16, 1.000000000000000000, 0.000000000000000000 ) ) ;
#10060=ORIENTED_EDGE ( 'NONE', *, *, #2346, .F. ) ;
#10063=ORIENTED_EDGE ( 'NONE', *, *, #19345, .T. ) ;
#10068=VECTOR ( 'NONE', #15856, 1000.000000000000000 ) ;
#10069=CARTESIAN_POINT ( 'NONE',  ( 172.0152310637604387, -4.999999999999970690, -17.38167787843871182 ) ) ;
#10074=CARTESIAN_POINT ( 'NONE',  ( 133.7287565553229172, -1.999999999999980904, -39.49999999999997158 ) ) ;
#10075=VERTEX_POINT ( 'NONE', #2506 ) ;
#10076=FACE_BOUND ( 'NONE', #7374, .T. ) ;
#10077=VECTOR ( 'NONE', #23246, 1000.000000000000000 ) ;
#10078=LINE ( 'NONE', #23848, #30195 ) ;
#10079=DIRECTION ( 'NONE',  ( 0.5877852522924731371, 0.000000000000000000, 0.8090169943749474513 ) ) ;
#10081=VECTOR ( 'NONE', #9910, 1000.000000000000000 ) ;
#10085=ORIENTED_EDGE ( 'NONE', *, *, #15928, .T. ) ;
#10086=LINE ( 'NONE', #28604, #1266 ) ;
#10089=ORIENTED_EDGE ( 'NONE', *, *, #1757, .T. ) ;
#10093=CARTESIAN_POINT ( 'NONE',  ( 139.5152310637605808, -1.999999999999979128, -2.627941064794695691 ) ) ;
#10094=ORIENTED_EDGE ( 'NONE', *, *, #13854, .T. ) ;
#10095=CARTESIAN_POINT ( 'NONE',  ( 167.2287565553229456, -1.999999999999970912, -20.83012701892220520 ) ) ;
#10098=EDGE_CURVE ( 'NONE', #1963, #25081, #11774, .T. ) ;
#10099=VERTEX_POINT ( 'NONE', #1250 ) ;
#10100=EDGE_CURVE ( 'NONE', #6453, #10227, #7812, .T. ) ;
#10103=VERTEX_POINT ( 'NONE', #25020 ) ;
#10105=VECTOR ( 'NONE', #14728, 1000.000000000000000 ) ;
#10106=LINE ( 'NONE', #8121, #21333 ) ;
#10109=ORIENTED_EDGE ( 'NONE', *, *, #16518, .T. ) ;
#10110=DIRECTION ( 'NONE',  ( 0.9510565162951535312, 2.566386769018988816E-16, -0.3090169943749475623 ) ) ;
#10112=AXIS2_PLACEMENT_3D ( 'NONE', #16684, #7678, #23406 ) ;
#10114=ORIENTED_EDGE ( 'NONE', *, *, #28621, .T. ) ;
#10115=PLANE ( 'NONE',  #16708 ) ;
#10116=ORIENTED_EDGE ( 'NONE', *, *, #1075, .F. ) ;
#10117=DIRECTION ( 'NONE',  ( 0.5877852522924731371, 1.586114251531760728E-16, 0.8090169943749474513 ) ) ;
#10118=VECTOR ( 'NONE', #29054, 1000.000000000000000 ) ;
#10119=CARTESIAN_POINT ( 'NONE',  ( 147.0152310637606092, -1.999999999999976241, -24.27857615940569502 ) ) ;
#10120=CARTESIAN_POINT ( 'NONE',  ( 142.0152310637605808, -4.999999999999979572, -1.576685793744487594E-14 ) ) ;
#10121=LINE ( 'NONE', #7691, #28244 ) ;
#10122=CARTESIAN_POINT ( 'NONE',  ( 10.04317065217474436, -5.000000000000015099, 30.90970097723984722 ) ) ;
#10128=EDGE_LOOP ( 'NONE', ( #26608, #26061, #16980, #9437 ) ) ;
#10131=DIRECTION ( 'NONE',  ( -2.698458740408366372E-16, 1.000000000000000000, 0.000000000000000000 ) ) ;
#10132=CARTESIAN_POINT ( 'NONE',  ( 172.2287565553229172, -1.999999999999969580, -20.83012701892220520 ) ) ;
#10133=PLANE ( 'NONE',  #24447 ) ;
#10136=ORIENTED_EDGE ( 'NONE', *, *, #23014, .T. ) ;
#10137=FACE_OUTER_BOUND ( 'NONE', #15974, .T. ) ;
#10140=CARTESIAN_POINT ( 'NONE',  ( 169.7287565553229456, -4.999999999999971578, -16.50000000000000000 ) ) ;
#10143=EDGE_CURVE ( 'NONE', #3931, #10985, #8097, .T. ) ;
#10145=ORIENTED_EDGE ( 'NONE', *, *, #308, .F. ) ;
#10151=VECTOR ( 'NONE', #19676, 999.9999999999998863 ) ;
#10153=CARTESIAN_POINT ( 'NONE',  ( 176.1922820468853104, -9.999999999999994671, -22.25671179336496053 ) ) ;
#10154=VECTOR ( 'NONE', #11564, 1000.000000000000000 ) ;
#10155=VECTOR ( 'NONE', #13212, 1000.000000000000000 ) ;
#10157=ORIENTED_EDGE ( 'NONE', *, *, #15593, .F. ) ;
#10158=DIRECTION ( 'NONE',  ( -2.698458740408365879E-16, 1.000000000000000000, 0.000000000000000000 ) ) ;
#10159=DIRECTION ( 'NONE',  ( -0.8090169943749474513, -2.183098979609982436E-16, 0.5877852522924731371 ) ) ;
#10161=EDGE_CURVE ( 'NONE', #14150, #21061, #5378, .T. ) ;
#10164=CARTESIAN_POINT ( 'NONE',  ( 167.0152310637605240, -4.999999999999972466, -34.70218595412750773 ) ) ;
#10165=LINE ( 'NONE', #28536, #30044 ) ;
#10167=DIRECTION ( 'NONE',  ( 0.9510565162951535312, 2.566386769018988816E-16, -0.3090169943749475623 ) ) ;
#10168=CARTESIAN_POINT ( 'NONE',  ( 10.28378231829363898, -5.000000000000015099, 31.65022754090628254 ) ) ;
#10169=ORIENTED_EDGE ( 'NONE', *, *, #4643, .T. ) ;
#10170=AXIS2_PLACEMENT_3D ( 'NONE', #15004, #6016, #22344 ) ;
#10172=CARTESIAN_POINT ( 'NONE',  ( 172.2287565553228603, -1.999999999999970468, -3.509618943233403510 ) ) ;
#10173=ADVANCED_FACE ( 'NONE', ( #19697 ), #14661, .T. ) ;
#10175=CARTESIAN_POINT ( 'NONE',  ( 101.2386341848420699, -4.999999999999990230, 73.55417321246510198 ) ) ;
#10177=ADVANCED_FACE ( 'NONE', ( #26591 ), #21690, .T. ) ;
#10178=VECTOR ( 'NONE', #16618, 1000.000000000000000 ) ;
#10180=ADVANCED_FACE ( 'NONE', ( #21546 ), #7953, .T. ) ;
#10182=VECTOR ( 'NONE', #26776, 1000.000000000000000 ) ;
#10185=LINE ( 'NONE', #19496, #28754 ) ;
#10186=DIRECTION ( 'NONE',  ( -2.698458740408365879E-16, 1.000000000000000000, 0.000000000000000000 ) ) ;
#10187=FACE_OUTER_BOUND ( 'NONE', #5556, .T. ) ;
#10188=CARTESIAN_POINT ( 'NONE',  ( 147.0152310637606092, -4.999999999999976907, -24.27857615940569502 ) ) ;
#10198=EDGE_LOOP ( 'NONE', ( #3753, #19408, #3663, #725 ) ) ;
#10202=FACE_BOUND ( 'NONE', #20795, .T. ) ;
#10203=VERTEX_POINT ( 'NONE', #5525 ) ;
#10207=DIRECTION ( 'NONE',  ( -0.9510565162951536422, -2.566386769018988323E-16, 0.3090169943749475623 ) ) ;
#10208=VERTEX_POINT ( 'NONE', #26291 ) ;
#10209=ADVANCED_FACE ( 'NONE', ( #6400 ), #15691, .T. ) ;
#10210=CARTESIAN_POINT ( 'NONE',  ( 144.5152310637605240, -1.999999999999978018, -4.391296821672111328 ) ) ;
#10211=VERTEX_POINT ( 'NONE', #10388 ) ;
#10213=EDGE_CURVE ( 'NONE', #20918, #18221, #12831, .T. ) ;
#10215=ORIENTED_EDGE ( 'NONE', *, *, #2009, .T. ) ;
#10221=ORIENTED_EDGE ( 'NONE', *, *, #27973, .F. ) ;
#10222=VECTOR ( 'NONE', #26835, 1000.000000000000000 ) ;
#10223=LINE ( 'NONE', #29669, #27919 ) ;
#10227=VERTEX_POINT ( 'NONE', #16966 ) ;
#10228=FACE_BOUND ( 'NONE', #20948, .T. ) ;
#10230=EDGE_CURVE ( 'NONE', #10227, #12932, #3250, .T. ) ;
#10231=PLANE ( 'NONE',  #28225 ) ;
#10232=CARTESIAN_POINT ( 'NONE',  ( 129.5152310637605808, -1.999999999999982236, -28.60870317832789311 ) ) ;
#10234=FACE_OUTER_BOUND ( 'NONE', #27158, .T. ) ;
#10235=CARTESIAN_POINT ( 'NONE',  ( 137.2287565553230309, -1.999999999999979572, -3.509618943233403510 ) ) ;
#10239=ORIENTED_EDGE ( 'NONE', *, *, #25757, .T. ) ;
#10242=LINE ( 'NONE', #29537, #12696 ) ;
#10243=DIRECTION ( 'NONE',  ( -2.908569913943825554E-16, 1.000000000000000000, -0.000000000000000000 ) ) ;
#10244=CARTESIAN_POINT ( 'NONE',  ( 132.0152310637605524, -1.999999999999981348, -34.70218595412750773 ) ) ;
#10250=ORIENTED_EDGE ( 'NONE', *, *, #27396, .F. ) ;
#10252=VECTOR ( 'NONE', #1005, 1000.000000000000000 ) ;
#10255=CARTESIAN_POINT ( 'NONE',  ( 113.2356977018776263, -4.999999999999986677, -82.27055006877300514 ) ) ;
#10260=AXIS2_PLACEMENT_3D ( 'NONE', #5782, #5936, #24552 ) ;
#10264=DIRECTION ( 'NONE',  ( -0.5877852522924731371, 0.000000000000000000, 0.8090169943749474513 ) ) ;
#10265=DIRECTION ( 'NONE',  ( -1.000000000000000000, 0.000000000000000000, -0.000000000000000000 ) ) ;
#10267=ADVANCED_FACE ( 'NONE', ( #2278 ), #23313, .T. ) ;
#10268=EDGE_CURVE ( 'NONE', #21323, #16948, #30244, .T. ) ;
#10269=LINE ( 'NONE', #12264, #16373 ) ;
#10271=VECTOR ( 'NONE', #25807, 1000.000000000000000 ) ;
#10272=ADVANCED_FACE ( 'NONE', ( #27784 ), #11703, .T. ) ;
#10273=CARTESIAN_POINT ( 'NONE',  ( 149.5152310637605524, -10.00000000000000178, -21.71180489736091346 ) ) ;
#10274=ORIENTED_EDGE ( 'NONE', *, *, #8357, .F. ) ;
#10281=CARTESIAN_POINT ( 'NONE',  ( 180.7287565553229740, -84.33034373659253902, -33.50000000000000000 ) ) ;
#10282=CARTESIAN_POINT ( 'NONE',  ( 154.5152310637605240, -10.00000000000000000, -21.71180489736091346 ) ) ;
#10283=CARTESIAN_POINT ( 'NONE',  ( 164.5152310637604955, -9.999999999999996447, -30.37205893520531319 ) ) ;
#10284=CARTESIAN_POINT ( 'NONE',  ( 143.6922820468854241, -1.999999999999978462, -9.266330736598359152 ) ) ;
#10287=ORIENTED_EDGE ( 'NONE', *, *, #23243, .T. ) ;
#10288=ORIENTED_EDGE ( 'NONE', *, *, #11656, .F. ) ;
#10289=CARTESIAN_POINT ( 'NONE',  ( 168.6922820468853956, -9.999999999999996447, -35.24709285013155835 ) ) ;
#10292=DIRECTION ( 'NONE',  ( 0.9510565162951536422, 0.000000000000000000, -0.3090169943749475623 ) ) ;
#10294=LINE ( 'NONE', #22358, #4734 ) ;
#10298=VECTOR ( 'NONE', #26037, 1000.000000000000000 ) ;
#10299=AXIS2_PLACEMENT_3D ( 'NONE', #25390, #17893, #2203 ) ;
#10301=AXIS2_PLACEMENT_3D ( 'NONE', #4970, #560, #21143 ) ;
#10305=EDGE_LOOP ( 'NONE', ( #10023, #27467, #18763, #15744 ) ) ;
#10306=EDGE_CURVE ( 'NONE', #3603, #28443, #9105, .T. ) ;
#10307=ORIENTED_EDGE ( 'NONE', *, *, #18379, .T. ) ;
#10308=DIRECTION ( 'NONE',  ( 0.3090169943749475623, 8.338696094058001131E-17, 0.9510565162951536422 ) ) ;
#10310=CARTESIAN_POINT ( 'NONE',  ( 84.87592175515526094, -4.999999999999994671, 61.66596675877570988 ) ) ;
#10313=DIRECTION ( 'NONE',  ( -1.110223024625156540E-16, 0.000000000000000000, -1.000000000000000000 ) ) ;
#10316=CARTESIAN_POINT ( 'NONE',  ( 174.7287565553229456, -4.999999999999969802, -33.82050807568879947 ) ) ;
#10319=DIRECTION ( 'NONE',  ( 0.5877852522924731371, 0.000000000000000000, 0.8090169943749474513 ) ) ;
#10320=ORIENTED_EDGE ( 'NONE', *, *, #13610, .T. ) ;
#10321=LINE ( 'NONE', #5761, #281 ) ;
#10322=ORIENTED_EDGE ( 'NONE', *, *, #26256, .F. ) ;
#10323=ORIENTED_EDGE ( 'NONE', *, *, #27730, .F. ) ;
#10325=CARTESIAN_POINT ( 'NONE',  ( 167.2287565553229740, -9.999999999999996447, -29.49038105676660493 ) ) ;
#10326=VECTOR ( 'NONE', #13162, 1000.000000000000000 ) ;
#10327=DIRECTION ( 'NONE',  ( 1.000000000000000000, 2.698458740408365879E-16, -1.110223024625156540E-16 ) ) ;
#10328=ORIENTED_EDGE ( 'NONE', *, *, #29293, .T. ) ;
#10329=ORIENTED_EDGE ( 'NONE', *, *, #10522, .F. ) ;
#10333=CARTESIAN_POINT ( 'NONE',  ( 169.5152310637604671, -4.999999999999971578, -11.28819510263909542 ) ) ;
#10334=DIRECTION ( 'NONE',  ( -2.698458740408365879E-16, 1.000000000000000000, 0.000000000000000000 ) ) ;
#10335=VECTOR ( 'NONE', #6870, 1000.000000000000000 ) ;
#10336=CARTESIAN_POINT ( 'NONE',  ( 133.6922820468854241, -4.999999999999982236, -0.6060766987539614181 ) ) ;
#10337=ORIENTED_EDGE ( 'NONE', *, *, #26498, .F. ) ;
#10338=DIRECTION ( 'NONE',  ( 1.110223024625156540E-16, 2.995891024602366092E-32, 1.000000000000000000 ) ) ;
#10339=VERTEX_POINT ( 'NONE', #1831 ) ;
#10340=DIRECTION ( 'NONE',  ( -0.5877852522924731371, -1.586114251531760235E-16, 0.8090169943749474513 ) ) ;
#10341=CARTESIAN_POINT ( 'NONE',  ( 91.48631020676766923, -4.999999999999992895, -66.46869509550764121 ) ) ;
#10342=VERTEX_POINT ( 'NONE', #11400 ) ;
#10343=EDGE_CURVE ( 'NONE', #20011, #28465, #23161, .T. ) ;
#10344=CARTESIAN_POINT ( 'NONE',  ( 141.1922820468854525, -10.00000000000000533, -10.74328820663507678 ) ) ;
#10345=CARTESIAN_POINT ( 'NONE',  ( 168.6922820468853104, -4.999999999999972466, -9.266330736598359152 ) ) ;
#10346=EDGE_CURVE ( 'NONE', #15181, #19023, #4549, .T. ) ;
#10350=VERTEX_POINT ( 'NONE', #16282 ) ;
#10352=VERTEX_POINT ( 'NONE', #30096 ) ;
#10354=VECTOR ( 'NONE', #28409, 1000.000000000000000 ) ;
#10357=FACE_BOUND ( 'NONE', #21085, .T. ) ;
#10358=ORIENTED_EDGE ( 'NONE', *, *, #21166, .F. ) ;
#10359=ORIENTED_EDGE ( 'NONE', *, *, #23419, .T. ) ;
#10362=DIRECTION ( 'NONE',  ( -2.698458740408365879E-16, 1.000000000000000000, 0.000000000000000000 ) ) ;
#10364=DIRECTION ( 'NONE',  ( -2.698458740408365879E-16, 1.000000000000000000, 0.000000000000000000 ) ) ;
#10365=ORIENTED_EDGE ( 'NONE', *, *, #28976, .T. ) ;
#10367=VERTEX_POINT ( 'NONE', #6543 ) ;
#10370=VECTOR ( 'NONE', #23962, 1000.000000000000000 ) ;
#10371=LINE ( 'NONE', #8081, #30200 ) ;
#10372=ORIENTED_EDGE ( 'NONE', *, *, #16179, .T. ) ;
#10374=ADVANCED_FACE ( 'NONE', ( #28081 ), #25163, .T. ) ;
#10377=AXIS2_PLACEMENT_3D ( 'NONE', #28072, #13688, #9095 ) ;
#10378=DIRECTION ( 'NONE',  ( -1.110223024625156540E-16, 0.000000000000000000, -1.000000000000000000 ) ) ;
#10379=FACE_BOUND ( 'NONE', #7632, .T. ) ;
#10380=EDGE_CURVE ( 'NONE', #5681, #17796, #6848, .T. ) ;
#10381=EDGE_CURVE ( 'NONE', #20167, #6302, #21020, .T. ) ;
#10383=CARTESIAN_POINT ( 'NONE',  ( 164.5152310637604955, -9.999999999999998224, -19.94844914048349693 ) ) ;
#10384=CARTESIAN_POINT ( 'NONE',  ( 154.7287565553230309, -10.00000000000000000, -33.82050807568879947 ) ) ;
#10385=CARTESIAN_POINT ( 'NONE',  ( 80.75772623742359713, -4.999999999999995559, 58.67392257650259779 ) ) ;
#10388=CARTESIAN_POINT ( 'NONE',  ( 171.1922820468853388, -1.999999999999970912, -19.40354224447947828 ) ) ;
#10389=ORIENTED_EDGE ( 'NONE', *, *, #9544, .F. ) ;
#10390=CARTESIAN_POINT ( 'NONE',  ( 144.5152310637605808, -4.999999999999978684, -11.28819510263909542 ) ) ;
#10393=VERTEX_POINT ( 'NONE', #23028 ) ;
#10394=VECTOR ( 'NONE', #21580, 1000.000000000000000 ) ;
#10396=LINE ( 'NONE', #17715, #10763 ) ;
#10397=CARTESIAN_POINT ( 'NONE',  ( 164.5152310637604671, -1.999999999999972689, -2.627941064794695691 ) ) ;
#10398=ORIENTED_EDGE ( 'NONE', *, *, #28071, .T. ) ;
#10399=LINE ( 'NONE', #3116, #4685 ) ;
#10400=ORIENTED_EDGE ( 'NONE', *, *, #5511, .F. ) ;
#10404=VERTEX_POINT ( 'NONE', #13399 ) ;
#10405=VERTEX_POINT ( 'NONE', #22727 ) ;
#10406=DIRECTION ( 'NONE',  ( 0.9510565162951536422, 2.566386769018988816E-16, 0.3090169943749472292 ) ) ;
#10410=EDGE_CURVE ( 'NONE', #19213, #26420, #15832, .T. ) ;
#10414=VERTEX_POINT ( 'NONE', #2715 ) ;
#10415=ORIENTED_EDGE ( 'NONE', *, *, #28278, .T. ) ;
#10417=VECTOR ( 'NONE', #24403, 1000.000000000000000 ) ;
#10421=CARTESIAN_POINT ( 'NONE',  ( 138.6922820468854525, -10.00000000000000533, -26.58683881228715506 ) ) ;
#10425=ORIENTED_EDGE ( 'NONE', *, *, #29866, .T. ) ;
#10426=CARTESIAN_POINT ( 'NONE',  ( 177.2287565553228319, -1.999999999999969358, -3.509618943233403510 ) ) ;
#10427=DIRECTION ( 'NONE',  ( -2.698458740408365879E-16, 1.000000000000000000, 0.000000000000000000 ) ) ;
#10428=CARTESIAN_POINT ( 'NONE',  ( 159.5152310637605524, -1.999999999999972689, -28.60870317832789667 ) ) ;
#10429=FACE_OUTER_BOUND ( 'NONE', #11589, .T. ) ;
#10431=CARTESIAN_POINT ( 'NONE',  ( 147.0152310637606092, -1.999999999999976241, -32.93883019725009120 ) ) ;
#10433=ORIENTED_EDGE ( 'NONE', *, *, #8104, .T. ) ;
#10434=LINE ( 'NONE', #8002, #23187 ) ;
#10437=PLANE ( 'NONE',  #6420 ) ;
#10438=ORIENTED_EDGE ( 'NONE', *, *, #5852, .T. ) ;
#10440=AXIS2_PLACEMENT_3D ( 'NONE', #15332, #24517, #20370 ) ;
#10443=EDGE_LOOP ( 'NONE', ( #14361, #29033, #21426, #17011 ) ) ;
#10444=DIRECTION ( 'NONE',  ( -0.9510565162951536422, 0.000000000000000000, -0.3090169943749472292 ) ) ;
#10446=DIRECTION ( 'NONE',  ( 1.000000000000000000, 0.000000000000000000, 0.000000000000000000 ) ) ;
#10448=EDGE_CURVE ( 'NONE', #22172, #8011, #24079, .T. ) ;
#10452=VERTEX_POINT ( 'NONE', #5302 ) ;
#10453=LINE ( 'NONE', #24661, #29856 ) ;
#10454=ORIENTED_EDGE ( 'NONE', *, *, #25072, .T. ) ;
#10455=DIRECTION ( 'NONE',  ( -2.698458740408365879E-16, 1.000000000000000000, 0.000000000000000000 ) ) ;
#10456=ORIENTED_EDGE ( 'NONE', *, *, #3113, .F. ) ;
#10459=PLANE ( 'NONE',  #14328 ) ;
#10464=FACE_OUTER_BOUND ( 'NONE', #1219, .T. ) ;
#10467=FACE_OUTER_BOUND ( 'NONE', #1849, .T. ) ;
#10470=LINE ( 'NONE', #17646, #2990 ) ;
#10471=EDGE_LOOP ( 'NONE', ( #12730, #24869, #14196, #29894 ) ) ;
#10472=DIRECTION ( 'NONE',  ( -0.5877852522924731371, 0.000000000000000000, 0.8090169943749474513 ) ) ;
#10473=VERTEX_POINT ( 'NONE', #3028 ) ;
#10474=ORIENTED_EDGE ( 'NONE', *, *, #1761, .T. ) ;
#10477=EDGE_CURVE ( 'NONE', #25465, #21788, #16748, .T. ) ;
#10478=EDGE_CURVE ( 'NONE', #14190, #27415, #16593, .T. ) ;
#10480=EDGE_CURVE ( 'NONE', #7930, #563, #2873, .T. ) ;
#10482=LINE ( 'NONE', #19790, #13554 ) ;
#10484=AXIS2_PLACEMENT_3D ( 'NONE', #11146, #10986, #2159 ) ;
#10485=EDGE_CURVE ( 'NONE', #18105, #29393, #26220, .T. ) ;
#10486=DIRECTION ( 'NONE',  ( -0.9510565162951536422, 0.000000000000000000, -0.3090169943749472292 ) ) ;
#10487=ORIENTED_EDGE ( 'NONE', *, *, #20775, .F. ) ;
#10488=CARTESIAN_POINT ( 'NONE',  ( 173.6922820468853388, -9.999999999999994671, -23.73366926340167637 ) ) ;
#10489=AXIS2_PLACEMENT_3D ( 'NONE', #11228, #20530, #25276 ) ;
#10491=ORIENTED_EDGE ( 'NONE', *, *, #21791, .F. ) ;
#10492=DIRECTION ( 'NONE',  ( -2.698458740408365879E-16, 1.000000000000000000, 0.000000000000000000 ) ) ;
#10493=LINE ( 'NONE', #5175, #27529 ) ;
#10497=VECTOR ( 'NONE', #24294, 1000.000000000000000 ) ;
#10501=FACE_BOUND ( 'NONE', #4262, .T. ) ;
#10502=EDGE_CURVE ( 'NONE', #2770, #9840, #14587, .T. ) ;
#10503=ORIENTED_EDGE ( 'NONE', *, *, #12931, .T. ) ;
#10504=EDGE_LOOP ( 'NONE', ( #1122, #26852, #1280, #10556, #1426 ) ) ;
#10509=ORIENTED_EDGE ( 'NONE', *, *, #14268, .T. ) ;
#10511=ORIENTED_EDGE ( 'NONE', *, *, #12371, .T. ) ;
#10513=ORIENTED_EDGE ( 'NONE', *, *, #8833, .F. ) ;
#10517=EDGE_CURVE ( 'NONE', #506, #21151, #9867, .T. ) ;
#10518=VECTOR ( 'NONE', #6406, 1000.000000000000000 ) ;
#10519=CARTESIAN_POINT ( 'NONE',  ( 18.15135754085015662, -5.000000000000012434, -55.86413428085646160 ) ) ;
#10520=EDGE_CURVE ( 'NONE', #1114, #22451, #10165, .T. ) ;
#10521=ORIENTED_EDGE ( 'NONE', *, *, #20242, .F. ) ;
#10522=EDGE_CURVE ( 'NONE', #11518, #17686, #26374, .T. ) ;
#10523=EDGE_CURVE ( 'NONE', #29689, #12166, #25918, .T. ) ;
#10525=VECTOR ( 'NONE', #16107, 1000.000000000000000 ) ;
#10529=FACE_BOUND ( 'NONE', #14123, .T. ) ;
#10530=ORIENTED_EDGE ( 'NONE', *, *, #20329, .F. ) ;
#10532=DIRECTION ( 'NONE',  ( 0.5877852522924731371, 1.586114251531760728E-16, 0.8090169943749474513 ) ) ;
#10534=FACE_OUTER_BOUND ( 'NONE', #12403, .T. ) ;
#10535=VECTOR ( 'NONE', #24811, 1000.000000000000000 ) ;
#10538=ORIENTED_EDGE ( 'NONE', *, *, #19448, .T. ) ;
#10539=DIRECTION ( 'NONE',  ( 0.3090169943749472292, 8.338696094057992503E-17, -0.9510565162951536422 ) ) ;
#10540=VERTEX_POINT ( 'NONE', #12306 ) ;
#10543=ORIENTED_EDGE ( 'NONE', *, *, #28912, .F. ) ;
#10544=AXIS2_PLACEMENT_3D ( 'NONE', #6872, #2598, #18296 ) ;
#10547=LINE ( 'NONE', #17567, #6703 ) ;
#10548=EDGE_LOOP ( 'NONE', ( #12998, #12952, #25242, #27686, #29327 ) ) ;
#10549=VERTEX_POINT ( 'NONE', #12452 ) ;
#10553=ORIENTED_EDGE ( 'NONE', *, *, #10697, .F. ) ;
#10556=ORIENTED_EDGE ( 'NONE', *, *, #13107, .T. ) ;
#10557=EDGE_CURVE ( 'NONE', #19068, #14895, #21622, .T. ) ;
#10558=VERTEX_POINT ( 'NONE', #21778 ) ;
#10559=EDGE_CURVE ( 'NONE', #11271, #23695, #12158, .T. ) ;
#10560=CARTESIAN_POINT ( 'NONE',  ( 91.06348369087051253, -4.999999999999992895, -66.16149364974000946 ) ) ;
#10562=ADVANCED_FACE ( 'NONE', ( #25761 ), #28237, .T. ) ;
#10564=EDGE_CURVE ( 'NONE', #22699, #18794, #5146, .T. ) ;
#10566=VERTEX_POINT ( 'NONE', #14285 ) ;
#10569=VECTOR ( 'NONE', #27434, 1000.000000000000000 ) ;
#10570=ORIENTED_EDGE ( 'NONE', *, *, #28738, .T. ) ;
#10571=CARTESIAN_POINT ( 'NONE',  ( 159.5152310637604671, -4.999999999999974243, -2.627941064794695691 ) ) ;
#10574=VECTOR ( 'NONE', #22301, 1000.000000000000000 ) ;
#10575=CARTESIAN_POINT ( 'NONE',  ( 161.1922820468853388, -1.999999999999974021, -19.40354224447947473 ) ) ;
#10576=DIRECTION ( 'NONE',  ( -2.698458740408365879E-16, 1.000000000000000000, 0.000000000000000000 ) ) ;
#10577=CARTESIAN_POINT ( 'NONE',  ( 164.5152310637605240, -1.999999999999971356, -28.60870317832789667 ) ) ;
#10578=CARTESIAN_POINT ( 'NONE',  ( 151.1922820468854525, -10.00000000000000178, -28.06379628232387802 ) ) ;
#10581=EDGE_CURVE ( 'NONE', #10720, #27442, #23618, .T. ) ;
#10582=ORIENTED_EDGE ( 'NONE', *, *, #20369, .F. ) ;
#10584=CARTESIAN_POINT ( 'NONE',  ( 148.6922820468854525, -1.999999999999976241, -35.24709285013155835 ) ) ;
#10585=CARTESIAN_POINT ( 'NONE',  ( 147.0152310637606092, -10.00000000000000178, -24.27857615940569502 ) ) ;
#10588=DIRECTION ( 'NONE',  ( 0.3090169943749475623, 8.338696094058001131E-17, 0.9510565162951536422 ) ) ;
#10590=ORIENTED_EDGE ( 'NONE', *, *, #27038, .T. ) ;
#10594=AXIS2_PLACEMENT_3D ( 'NONE', #4042, #2369, #25542 ) ;
#10596=CARTESIAN_POINT ( 'NONE',  ( 168.6922820468853956, -1.999999999999970468, -35.24709285013155835 ) ) ;
#10598=CARTESIAN_POINT ( 'NONE',  ( 134.5152310637605808, -1.999999999999980460, -11.28819510263909187 ) ) ;
#10601=EDGE_CURVE ( 'NONE', #5840, #4938, #23779, .T. ) ;
#10602=DIRECTION ( 'NONE',  ( -1.000000000000000000, -2.891205793294689173E-16, 0.000000000000000000 ) ) ;
#10605=EDGE_CURVE ( 'NONE', #21255, #27873, #24526, .T. ) ;
#10610=VECTOR ( 'NONE', #10158, 1000.000000000000000 ) ;
#10611=DIRECTION ( 'NONE',  ( -2.698458740408365879E-16, 1.000000000000000000, 0.000000000000000000 ) ) ;
#10612=ORIENTED_EDGE ( 'NONE', *, *, #8693, .T. ) ;
#10613=LINE ( 'NONE', #17328, #27338 ) ;
#10614=VECTOR ( 'NONE', #10406, 1000.000000000000000 ) ;
#10615=PLANE ( 'NONE',  #27710 ) ;
#10616=LINE ( 'NONE', #20220, #23129 ) ;
#10622=PLANE ( 'NONE',  #9514 ) ;
#10625=DIRECTION ( 'NONE',  ( -2.698458740408365879E-16, 1.000000000000000000, 0.000000000000000000 ) ) ;
#10628=LINE ( 'NONE', #1188, #27674 ) ;
#10631=CARTESIAN_POINT ( 'NONE',  ( 22.04996626933243675, -5.000000000000011546, -67.86281818239412189 ) ) ;
#10632=DIRECTION ( 'NONE',  ( 0.5877852522924731371, 0.000000000000000000, 0.8090169943749474513 ) ) ;
#10633=VECTOR ( 'NONE', #28454, 1000.000000000000000 ) ;
#10634=LINE ( 'NONE', #26850, #14144 ) ;
#10635=ORIENTED_EDGE ( 'NONE', *, *, #21425, .F. ) ;
#10636=VERTEX_POINT ( 'NONE', #5758 ) ;
#10638=ORIENTED_EDGE ( 'NONE', *, *, #21482, .F. ) ;
#10639=VECTOR ( 'NONE', #26860, 1000.000000000000000 ) ;
#10642=LINE ( 'NONE', #6072, #21381 ) ;
#10643=CARTESIAN_POINT ( 'NONE',  ( 142.0152310637605240, -1.999999999999978684, -0.06116980274991495881 ) ) ;
#10646=ORIENTED_EDGE ( 'NONE', *, *, #30124, .T. ) ;
#10647=CARTESIAN_POINT ( 'NONE',  ( 152.0152310637605240, -10.00000000000000178, -6.958068083716895558 ) ) ;
#10648=EDGE_LOOP ( 'NONE', ( #22250, #16734, #1383, #3450 ) ) ;
#10649=DIRECTION ( 'NONE',  ( -0.9510565162951536422, 0.000000000000000000, -0.3090169943749472292 ) ) ;
#10650=DIRECTION ( 'NONE',  ( 1.110223024625156540E-16, 2.995891024602366092E-32, 1.000000000000000000 ) ) ;
#10653=EDGE_CURVE ( 'NONE', #28202, #16318, #26683, .T. ) ;
#10654=EDGE_CURVE ( 'NONE', #15239, #10099, #22081, .T. ) ;
#10656=VECTOR ( 'NONE', #5102, 1000.000000000000000 ) ;
#10657=ORIENTED_EDGE ( 'NONE', *, *, #4609, .T. ) ;
#10660=EDGE_LOOP ( 'NONE', ( #2164, #18627, #1270, #4368, #4968 ) ) ;
#10664=FACE_BOUND ( 'NONE', #3017, .T. ) ;
#10666=ORIENTED_EDGE ( 'NONE', *, *, #11412, .F. ) ;
#10669=FACE_OUTER_BOUND ( 'NONE', #17032, .T. ) ;
#10671=CARTESIAN_POINT ( 'NONE',  ( 164.7287565553229456, -1.999999999999971356, -25.16025403784440329 ) ) ;
#10672=ORIENTED_EDGE ( 'NONE', *, *, #17996, .T. ) ;
#10673=PLANE ( 'NONE',  #826 ) ;
#10674=ORIENTED_EDGE ( 'NONE', *, *, #11570, .F. ) ;
#10676=ORIENTED_EDGE ( 'NONE', *, *, #23422, .F. ) ;
#10679=CARTESIAN_POINT ( 'NONE',  ( 133.6922820468854241, -1.999999999999981348, -32.39392330124607611 ) ) ;
#10684=ORIENTED_EDGE ( 'NONE', *, *, #14542, .F. ) ;
#10686=DIRECTION ( 'NONE',  ( 0.9510565162951536422, 0.000000000000000000, -0.3090169943749475623 ) ) ;
#10687=LINE ( 'NONE', #24286, #22063 ) ;
#10688=ORIENTED_EDGE ( 'NONE', *, *, #3283, .T. ) ;
#10689=CARTESIAN_POINT ( 'NONE',  ( 169.7287565553228887, -1.999999999999970912, -7.839745962155603820 ) ) ;
#10690=ADVANCED_FACE ( 'NONE', ( #1335 ), #1641, .T. ) ;
#10692=PLANE ( 'NONE',  #23366 ) ;
#10693=ORIENTED_EDGE ( 'NONE', *, *, #20922, .F. ) ;
#10694=ADVANCED_FACE ( 'NONE', ( #24229 ), #29617, .T. ) ;
#10697=EDGE_CURVE ( 'NONE', #26624, #28890, #19934, .T. ) ;
#10699=AXIS2_PLACEMENT_3D ( 'NONE', #14620, #11579, #14014 ) ;
#10702=CARTESIAN_POINT ( 'NONE',  ( 142.0152310637605808, -1.999999999999978018, -34.70218595412750773 ) ) ;
#10703=VERTEX_POINT ( 'NONE', #28992 ) ;
#10706=CARTESIAN_POINT ( 'NONE',  ( 154.7287565553229456, -1.999999999999974909, -7.839745962155603820 ) ) ;
#10707=CARTESIAN_POINT ( 'NONE',  ( 20.14013621308192015, -5.000000000000012434, -61.98496565946941672 ) ) ;
#10708=ORIENTED_EDGE ( 'NONE', *, *, #27556, .T. ) ;
#10712=VERTEX_POINT ( 'NONE', #3770 ) ;
#10713=PLANE ( 'NONE',  #4267 ) ;
#10715=DIRECTION ( 'NONE',  ( -2.908569913943825554E-16, 1.000000000000000000, -0.000000000000000000 ) ) ;
#10720=VERTEX_POINT ( 'NONE', #3328 ) ;
#10721=CARTESIAN_POINT ( 'NONE',  ( 157.2287565553229456, -4.999999999999976019, -3.509618943233400401 ) ) ;
#10722=AXIS2_PLACEMENT_3D ( 'NONE', #29770, #22690, #1946 ) ;
#10723=VECTOR ( 'NONE', #19131, 1000.000000000000000 ) ;
#10724=CARTESIAN_POINT ( 'NONE',  ( 154.7287565553229172, -1.999999999999975353, 0.8205080756887930260 ) ) ;
#10725=VECTOR ( 'NONE', #12153, 1000.000000000000000 ) ;
#10726=CARTESIAN_POINT ( 'NONE',  ( 132.2287565553230024, -1.999999999999981348, -3.509618943233403510 ) ) ;
#10728=DIRECTION ( 'NONE',  ( 0.3090169943749472292, 8.338696094057992503E-17, -0.9510565162951536422 ) ) ;
#10729=ADVANCED_FACE ( 'NONE', ( #10464 ), #12607, .T. ) ;
#10733=EDGE_CURVE ( 'NONE', #2968, #1559, #20089, .T. ) ;
#10735=ADVANCED_FACE ( 'NONE', ( #6208 ), #8484, .T. ) ;
#10737=VECTOR ( 'NONE', #11153, 1000.000000000000000 ) ;
#10738=ORIENTED_EDGE ( 'NONE', *, *, #22797, .T. ) ;
#10739=DIRECTION ( 'NONE',  ( 0.3090169943749472292, 8.338696094057992503E-17, -0.9510565162951536422 ) ) ;
#10740=DIRECTION ( 'NONE',  ( -0.9510565162951536422, 0.000000000000000000, -0.3090169943749472292 ) ) ;
#10741=ORIENTED_EDGE ( 'NONE', *, *, #12338, .T. ) ;
#10742=VECTOR ( 'NONE', #4775, 1000.000000000000000 ) ;
#10744=FACE_OUTER_BOUND ( 'NONE', #2517, .T. ) ;
#10748=CARTESIAN_POINT ( 'NONE',  ( 172.0152310637604103, -4.999999999999970690, 1.702185954127501066 ) ) ;
#10756=VERTEX_POINT ( 'NONE', #17490 ) ;
#10757=CARTESIAN_POINT ( 'NONE',  ( 144.7287565553230024, -1.999999999999977573, -7.839745962155603820 ) ) ;
#10760=ORIENTED_EDGE ( 'NONE', *, *, #11110, .T. ) ;
#10763=VECTOR ( 'NONE', #1259, 1000.000000000000000 ) ;
#10764=VERTEX_POINT ( 'NONE', #26841 ) ;
#10765=PLANE ( 'NONE',  #2128 ) ;
#10767=DIRECTION ( 'NONE',  ( 1.000000000000000000, 2.698458740408365879E-16, -1.110223024625156540E-16 ) ) ;
#10768=CARTESIAN_POINT ( 'NONE',  ( 139.5152310637606092, -10.00000000000000533, -19.94844914048349338 ) ) ;
#10770=CARTESIAN_POINT ( 'NONE',  ( 177.2287565553228887, -9.999999999999994671, -20.83012701892220520 ) ) ;
#10771=EDGE_CURVE ( 'NONE', #4670, #6014, #13803, .T. ) ;
#10775=CARTESIAN_POINT ( 'NONE',  ( 85.61150514570974224, -4.999999999999993783, 62.20039937490791715 ) ) ;
#10779=DIRECTION ( 'NONE',  ( 0.9510565162951536422, 0.000000000000000000, -0.3090169943749475623 ) ) ;
#10780=DIRECTION ( 'NONE',  ( -0.9510565162951536422, -2.566386769018988323E-16, 0.3090169943749475623 ) ) ;
#10782=CARTESIAN_POINT ( 'NONE',  ( 156.1922820468853672, -1.999999999999974465, -10.74328820663507678 ) ) ;
#10784=VECTOR ( 'NONE', #20228, 1000.000000000000000 ) ;
#10786=VERTEX_POINT ( 'NONE', #1944 ) ;
#10787=VECTOR ( 'NONE', #5885, 1000.000000000000000 ) ;
#10788=CARTESIAN_POINT ( 'NONE',  ( 158.6922820468853956, -4.999999999999974243, -23.73366926340167637 ) ) ;
#10789=DIRECTION ( 'NONE',  ( 0.9510565162951535312, 2.566386769018988816E-16, -0.3090169943749475623 ) ) ;
#10790=PLANE ( 'NONE',  #21956 ) ;
#10791=ORIENTED_EDGE ( 'NONE', *, *, #20768, .T. ) ;
#10797=DIRECTION ( 'NONE',  ( -1.110223024625156540E-16, 0.000000000000000000, -1.000000000000000000 ) ) ;
#10798=DIRECTION ( 'NONE',  ( 0.9510565162951536422, 0.000000000000000000, -0.3090169943749475623 ) ) ;
#10799=CARTESIAN_POINT ( 'NONE',  ( 147.2287565553229740, -4.999999999999978684, -3.509618943233400401 ) ) ;
#10800=EDGE_CURVE ( 'NONE', #7135, #8074, #25425, .T. ) ;
#10801=EDGE_LOOP ( 'NONE', ( #6149, #14297, #16292, #3499 ) ) ;
#10802=CARTESIAN_POINT ( 'NONE',  ( 114.3941076083291648, -4.999999999999985789, -83.11218413067275890 ) ) ;
#10804=DIRECTION ( 'NONE',  ( 0.5877852522924731371, 0.000000000000000000, 0.8090169943749474513 ) ) ;
#10807=VERTEX_POINT ( 'NONE', #8925 ) ;
#10809=VERTEX_POINT ( 'NONE', #2240 ) ;
#10810=VECTOR ( 'NONE', #4613, 1000.000000000000000 ) ;
#10813=FACE_BOUND ( 'NONE', #17536, .T. ) ;
#10815=DIRECTION ( 'NONE',  ( -2.698458740408365879E-16, 1.000000000000000000, 0.000000000000000000 ) ) ;
#10817=VECTOR ( 'NONE', #2632, 1000.000000000000000 ) ;
#10818=CARTESIAN_POINT ( 'NONE',  ( 134.5152310637605524, -4.999999999999981348, -1.493419066897600538E-14 ) ) ;
#10820=ORIENTED_EDGE ( 'NONE', *, *, #18340, .T. ) ;
#10827=EDGE_CURVE ( 'NONE', #28891, #5806, #2093, .T. ) ;
#10828=EDGE_CURVE ( 'NONE', #20539, #2343, #30058, .T. ) ;
#10832=PLANE ( 'NONE',  #123 ) ;
#10833=VECTOR ( 'NONE', #450, 1000.000000000000000 ) ;
#10834=ORIENTED_EDGE ( 'NONE', *, *, #12627, .T. ) ;
#10835=CARTESIAN_POINT ( 'NONE',  ( 154.7287565553229172, -10.00000000000000178, 0.8205080756887930260 ) ) ;
#10838=ORIENTED_EDGE ( 'NONE', *, *, #10605, .F. ) ;
#10840=DIRECTION ( 'NONE',  ( -2.698458740408365879E-16, 1.000000000000000000, 0.000000000000000000 ) ) ;
#10843=EDGE_LOOP ( 'NONE', ( #20002, #26411, #24954, #11738 ) ) ;
#10846=DIRECTION ( 'NONE',  ( 1.110223024625156540E-16, 2.995891024602366092E-32, 1.000000000000000000 ) ) ;
#10847=VERTEX_POINT ( 'NONE', #11511 ) ;
#10848=LINE ( 'NONE', #1569, #1796 ) ;
#10849=ORIENTED_EDGE ( 'NONE', *, *, #12763, .T. ) ;
#10854=ORIENTED_EDGE ( 'NONE', *, *, #16143, .F. ) ;
#10855=EDGE_LOOP ( 'NONE', ( #286, #1060, #27697, #17233, #15159 ) ) ;
#10858=CARTESIAN_POINT ( 'NONE',  ( 168.6922820468853388, -9.999999999999996447, -15.07341522555727664 ) ) ;
#10859=ORIENTED_EDGE ( 'NONE', *, *, #15893, .T. ) ;
#10861=EDGE_CURVE ( 'NONE', #1407, #7486, #9219, .T. ) ;
#10863=EDGE_CURVE ( 'NONE', #19955, #17748, #4070, .T. ) ;
#10866=VERTEX_POINT ( 'NONE', #18547 ) ;
#10867=CARTESIAN_POINT ( 'NONE',  ( 144.7287565553230309, -1.999999999999977129, -33.82050807568879947 ) ) ;
#10868=PLANE ( 'NONE',  #26795 ) ;
#10869=LINE ( 'NONE', #8283, #27511 ) ;
#10873=VECTOR ( 'NONE', #1435, 1000.000000000000000 ) ;
#10878=CARTESIAN_POINT ( 'NONE',  ( 172.7287565553229740, -84.33034373659253902, -33.50000000000000000 ) ) ;
#10879=ORIENTED_EDGE ( 'NONE', *, *, #28317, .F. ) ;
#10881=CARTESIAN_POINT ( 'NONE',  ( 174.5152310637604671, -1.999999999999968914, -30.37205893520531319 ) ) ;
#10883=CARTESIAN_POINT ( 'NONE',  ( 137.0152310637605808, -1.999999999999980016, 1.702185954127501066 ) ) ;
#10885=EDGE_LOOP ( 'NONE', ( #15823, #12310, #12168, #17902, #4520 ) ) ;
#10886=EDGE_LOOP ( 'NONE', ( #14250, #26922, #26625, #15633, #17652 ) ) ;
#10887=DIRECTION ( 'NONE',  ( -0.5877852522924731371, 0.000000000000000000, 0.8090169943749474513 ) ) ;
#10889=ADVANCED_FACE ( 'NONE', ( #20827 ), #18396, .T. ) ;
#10891=PLANE ( 'NONE',  #30089 ) ;
#10894=LINE ( 'NONE', #26079, #23768 ) ;
#10896=ORIENTED_EDGE ( 'NONE', *, *, #14577, .T. ) ;
#10898=( NAMED_UNIT ( * ) SI_UNIT ( $, .STERADIAN. ) SOLID_ANGLE_UNIT ( ) );
#10901=ADVANCED_FACE ( 'NONE', ( #25563 ), #4364, .T. ) ;
#10902=VECTOR ( 'NONE', #15066, 1000.000000000000000 ) ;
#10904=EDGE_CURVE ( 'NONE', #15699, #19168, #13951, .T. ) ;
#10906=VERTEX_POINT ( 'NONE', #27308 ) ;
#10909=CARTESIAN_POINT ( 'NONE',  ( 152.0152310637605808, -10.00000000000000000, -34.70218595412750773 ) ) ;
#10910=CARTESIAN_POINT ( 'NONE',  ( 172.0152310637604103, -4.999999999999970690, -8.721423840594312082 ) ) ;
#10912=LINE ( 'NONE', #8768, #17762 ) ;
#10919=VECTOR ( 'NONE', #4394, 1000.000000000000000 ) ;
#10920=CARTESIAN_POINT ( 'NONE',  ( 19.58373008303804141, -5.000000000000012434, -60.27252367304998870 ) ) ;
#10921=DIRECTION ( 'NONE',  ( 1.000000000000000000, 2.698458740408365879E-16, -1.110223024625156540E-16 ) ) ;
#10923=LINE ( 'NONE', #20231, #27357 ) ;
#10924=CARTESIAN_POINT ( 'NONE',  ( 163.6922820468853672, -1.999999999999971800, -23.73366926340167637 ) ) ;
#10926=VERTEX_POINT ( 'NONE', #13364 ) ;
#10927=FACE_OUTER_BOUND ( 'NONE', #9876, .T. ) ;
#10928=LINE ( 'NONE', #30068, #18565 ) ;
#10929=CARTESIAN_POINT ( 'NONE',  ( 144.7287565553230309, -10.00000000000000355, -25.16025403784439973 ) ) ;
#10930=VECTOR ( 'NONE', #16510, 1000.000000000000000 ) ;
#10931=ORIENTED_EDGE ( 'NONE', *, *, #17913, .F. ) ;
#10935=EDGE_CURVE ( 'NONE', #6165, #14559, #15656, .T. ) ;
#10937=DIRECTION ( 'NONE',  ( -0.8090169943749474513, -2.183098979609982436E-16, -0.5877852522924731371 ) ) ;
#10938=CARTESIAN_POINT ( 'NONE',  ( 137.2287565553230309, -10.00000000000000533, -20.83012701892220164 ) ) ;
#10939=EDGE_CURVE ( 'NONE', #19094, #2770, #27457, .T. ) ;
#10941=ADVANCED_FACE ( 'NONE', ( #13514 ), #22842, .T. ) ;
#10945=ORIENTED_EDGE ( 'NONE', *, *, #14949, .F. ) ;
#10946=CARTESIAN_POINT ( 'NONE',  ( 134.7287565553230024, -4.999999999999981348, 0.8205080756888000204 ) ) ;
#10949=PLANE ( 'NONE',  #5399 ) ;
#10953=EDGE_LOOP ( 'NONE', ( #14667, #29360, #25200, #25604 ) ) ;
#10957=DIRECTION ( 'NONE',  ( -2.698458740408365879E-16, 1.000000000000000000, 0.000000000000000000 ) ) ;
#10960=EDGE_LOOP ( 'NONE', ( #13599, #1910, #8217, #9771 ) ) ;
#10961=LINE ( 'NONE', #22731, #28587 ) ;
#10962=VECTOR ( 'NONE', #25637, 1000.000000000000000 ) ;
#10964=LINE ( 'NONE', #11124, #15968 ) ;
#10965=FACE_OUTER_BOUND ( 'NONE', #18424, .T. ) ;
#10968=ORIENTED_EDGE ( 'NONE', *, *, #4154, .F. ) ;
#10971=VERTEX_POINT ( 'NONE', #28049 ) ;
#10972=CARTESIAN_POINT ( 'NONE',  ( 11.39659457838139112, -5.000000000000014211, 35.07511151374514213 ) ) ;
#10973=ORIENTED_EDGE ( 'NONE', *, *, #12594, .F. ) ;
#10976=EDGE_LOOP ( 'NONE', ( #75, #21036, #11357, #21205 ) ) ;
#10979=CARTESIAN_POINT ( 'NONE',  ( 174.5152310637604387, -4.999999999999970690, -1.937508276747661892E-14 ) ) ;
#10980=DIRECTION ( 'NONE',  ( 0.9510565162951536422, 2.566386769018988816E-16, 0.3090169943749472292 ) ) ;
#10981=VERTEX_POINT ( 'NONE', #5270 ) ;
#10982=LINE ( 'NONE', #20290, #18021 ) ;
#10983=DIRECTION ( 'NONE',  ( 0.3090169943749472292, 8.338696094057992503E-17, -0.9510565162951536422 ) ) ;
#10984=FACE_OUTER_BOUND ( 'NONE', #18485, .T. ) ;
#10985=VERTEX_POINT ( 'NONE', #26038 ) ;
#10986=DIRECTION ( 'NONE',  ( -2.698458740408365879E-16, 1.000000000000000000, -0.000000000000000000 ) ) ;
#10987=EDGE_CURVE ( 'NONE', #22090, #7341, #7557, .T. ) ;
#10992=ORIENTED_EDGE ( 'NONE', *, *, #23593, .T. ) ;
#10994=EDGE_CURVE ( 'NONE', #8651, #22060, #12128, .T. ) ;
#10995=AXIS2_PLACEMENT_3D ( 'NONE', #24687, #4077, #28998 ) ;
#10997=DIRECTION ( 'NONE',  ( 0.3090169943749475623, 8.338696094058001131E-17, 0.9510565162951536422 ) ) ;
#11000=ORIENTED_EDGE ( 'NONE', *, *, #6567, .T. ) ;
#11001=LINE ( 'NONE', #13297, #5216 ) ;
#11002=VERTEX_POINT ( 'NONE', #7707 ) ;
#11004=VECTOR ( 'NONE', #20232, 1000.000000000000000 ) ;
#11007=EDGE_LOOP ( 'NONE', ( #5695, #30071, #29681, #25572 ) ) ;
#11008=VERTEX_POINT ( 'NONE', #554 ) ;
#11009=VECTOR ( 'NONE', #9977, 1000.000000000000000 ) ;
#11010=DIRECTION ( 'NONE',  ( -0.9510565162951536422, 0.000000000000000000, -0.3090169943749472292 ) ) ;
#11015=ORIENTED_EDGE ( 'NONE', *, *, #12550, .F. ) ;
#11016=ORIENTED_EDGE ( 'NONE', *, *, #23730, .T. ) ;
#11017=CARTESIAN_POINT ( 'NONE',  ( 130.7287565553229172, -10.00000000000000888, -19.55415080639416558 ) ) ;
#11018=CARTESIAN_POINT ( 'NONE',  ( 162.2287565553228887, -1.999999999999973133, -3.509618943233403510 ) ) ;
#11019=AXIS2_PLACEMENT_3D ( 'NONE', #3156, #19453, #12133 ) ;
#11020=CARTESIAN_POINT ( 'NONE',  ( 158.6922820468853672, -4.999999999999975131, -17.92658477444275889 ) ) ;
#11021=PLANE ( 'NONE',  #355 ) ;
#11024=DIRECTION ( 'NONE',  ( 0.5877852522924731371, 1.586114251531760728E-16, -0.8090169943749474513 ) ) ;
#11025=AXIS2_PLACEMENT_3D ( 'NONE', #22447, #4276, #13576 ) ;
#11029=DIRECTION ( 'NONE',  ( -2.698458740408365879E-16, 1.000000000000000000, 0.000000000000000000 ) ) ;
#11030=EDGE_CURVE ( 'NONE', #29780, #9765, #14404, .T. ) ;
#11031=EDGE_CURVE ( 'NONE', #26001, #8714, #24051, .T. ) ;
#11034=DIRECTION ( 'NONE',  ( 0.3090169943749472292, 8.338696094057992503E-17, -0.9510565162951536422 ) ) ;
#11035=EDGE_LOOP ( 'NONE', ( #13119, #17174, #17756, #5403 ) ) ;
#11038=DIRECTION ( 'NONE',  ( -2.698458740408365879E-16, 1.000000000000000000, 0.000000000000000000 ) ) ;
#11039=LINE ( 'NONE', #20053, #26858 ) ;
#11041=EDGE_CURVE ( 'NONE', #29646, #10393, #12424, .T. ) ;
#11044=ORIENTED_EDGE ( 'NONE', *, *, #4985, .F. ) ;
#11045=LINE ( 'NONE', #15914, #12988 ) ;
#11048=CARTESIAN_POINT ( 'NONE',  ( 132.0152310637605808, -4.999999999999981348, -6.958068083716893781 ) ) ;
#11051=CARTESIAN_POINT ( 'NONE',  ( 173.6922820468852819, -4.999999999999970690, -6.413161187712876909 ) ) ;
#11054=DIRECTION ( 'NONE',  ( -0.8090169943749474513, -2.183098979609982436E-16, 0.5877852522924731371 ) ) ;
#11056=AXIS2_PLACEMENT_3D ( 'NONE', #29508, #27641, #6707 ) ;
#11058=MECHANICAL_DESIGN_GEOMETRIC_PRESENTATION_REPRESENTATION('',(#7166),#26174);
#11059=VERTEX_POINT ( 'NONE', #18702 ) ;
#11060=PLANE ( 'NONE',  #14607 ) ;
#11061=VECTOR ( 'NONE', #16847, 1000.000000000000000 ) ;
#11062=DIRECTION ( 'NONE',  ( -0.8090169943749474513, -2.183098979609982436E-16, 0.5877852522924731371 ) ) ;
#11063=DIRECTION ( 'NONE',  ( -0.5877852522924731371, -1.586114251531760728E-16, -0.8090169943749474513 ) ) ;
#11064=CARTESIAN_POINT ( 'NONE',  ( 142.2287565553230024, -4.999999999999979572, -3.509618943233414168 ) ) ;
#11065=DIRECTION ( 'NONE',  ( -1.110223024625156540E-16, 0.000000000000000000, -1.000000000000000000 ) ) ;
#11066=VECTOR ( 'NONE', #11631, 1000.000000000000000 ) ;
#11070=EDGE_CURVE ( 'NONE', #18037, #11863, #21285, .T. ) ;
#11073=VECTOR ( 'NONE', #8458, 1000.000000000000000 ) ;
#11075=EDGE_CURVE ( 'NONE', #11059, #26241, #19004, .T. ) ;
#11076=CARTESIAN_POINT ( 'NONE',  ( 176.1922820468853388, -9.999999999999994671, -28.06379628232387802 ) ) ;
#11078=EDGE_CURVE ( 'NONE', #6062, #28182, #9523, .T. ) ;
#11080=LINE ( 'NONE', #25127, #15600 ) ;
#11081=DIRECTION ( 'NONE',  ( -0.8090169943749474513, -2.183098979609982436E-16, 0.5877852522924731371 ) ) ;
#11083=VECTOR ( 'NONE', #4615, 1000.000000000000000 ) ;
#11084=VERTEX_POINT ( 'NONE', #28207 ) ;
#11085=LINE ( 'NONE', #11234, #20280 ) ;
#11087=CARTESIAN_POINT ( 'NONE',  ( 144.5152310637605808, -10.00000000000000178, -21.71180489736091346 ) ) ;
#11097=VECTOR ( 'NONE', #9464, 999.9999999999998863 ) ;
#11098=ORIENTED_EDGE ( 'NONE', *, *, #957, .T. ) ;
#11099=DIRECTION ( 'NONE',  ( -0.5877852522924731371, -1.586114251531760235E-16, 0.8090169943749474513 ) ) ;
#11101=VERTEX_POINT ( 'NONE', #14103 ) ;
#11102=CARTESIAN_POINT ( 'NONE',  ( 138.6922820468854525, -1.999999999999979572, -9.266330736598359152 ) ) ;
#11103=CARTESIAN_POINT ( 'NONE',  ( 156.1922820468853956, -10.00000000000000000, -22.25671179336496053 ) ) ;
#11104=PLANE ( 'NONE',  #8282 ) ;
#11106=VERTEX_POINT ( 'NONE', #23437 ) ;
#11108=ORIENTED_EDGE ( 'NONE', *, *, #9544, .T. ) ;
#11109=EDGE_CURVE ( 'NONE', #16948, #5806, #28362, .T. ) ;
#11110=EDGE_CURVE ( 'NONE', #5536, #28522, #7261, .T. ) ;
#11113=CARTESIAN_POINT ( 'NONE',  ( 164.7287565553229172, -9.999999999999998224, -16.50000000000000355 ) ) ;
#11114=EDGE_CURVE ( 'NONE', #26028, #21141, #25886, .T. ) ;
#11116=FACE_OUTER_BOUND ( 'NONE', #17309, .T. ) ;
#11117=EDGE_CURVE ( 'NONE', #12000, #23017, #28508, .T. ) ;
#11118=EDGE_LOOP ( 'NONE', ( #1805, #19349, #29308, #8114 ) ) ;
#11119=ORIENTED_EDGE ( 'NONE', *, *, #11341, .T. ) ;
#11120=VECTOR ( 'NONE', #14789, 1000.000000000000000 ) ;
#11121=CARTESIAN_POINT ( 'NONE',  ( 144.7287565553230024, -10.00000000000000355, -7.839745962155603820 ) ) ;
#11122=ORIENTED_EDGE ( 'NONE', *, *, #9165, .F. ) ;
#11124=CARTESIAN_POINT ( 'NONE',  ( 175.7287565553229456, -4.999999999999970690, -22.10610323145030520 ) ) ;
#11125=EDGE_LOOP ( 'NONE', ( #27044, #22208, #21671, #4829 ) ) ;
#11126=CARTESIAN_POINT ( 'NONE',  ( 152.2287565553230024, -10.00000000000000178, -20.83012701892220520 ) ) ;
#11127=ORIENTED_EDGE ( 'NONE', *, *, #29831, .T. ) ;
#11132=FACE_OUTER_BOUND ( 'NONE', #7857, .T. ) ;
#11133=LINE ( 'NONE', #27509, #7433 ) ;
#11136=CARTESIAN_POINT ( 'NONE',  ( 132.0152310637605524, -1.999999999999981348, -8.721423840594310306 ) ) ;
#11137=CARTESIAN_POINT ( 'NONE',  ( 134.5152310637605808, -1.999999999999980460, -19.94844914048349338 ) ) ;
#11139=VERTEX_POINT ( 'NONE', #7998 ) ;
#11143=DIRECTION ( 'NONE',  ( -0.9510565162951536422, 0.000000000000000000, -0.3090169943749472292 ) ) ;
#11145=ORIENTED_EDGE ( 'NONE', *, *, #27219, .F. ) ;
#11146=CARTESIAN_POINT ( 'NONE',  ( 172.7287565553229456, -4.999999999999970690, 0.5000000000000029976 ) ) ;
#11148=VECTOR ( 'NONE', #6926, 1000.000000000000000 ) ;
#11151=EDGE_CURVE ( 'NONE', #17474, #9904, #13031, .T. ) ;
#11152=EDGE_LOOP ( 'NONE', ( #18283, #26267, #4397, #12764, #28401, #15775 ) ) ;
#11153=DIRECTION ( 'NONE',  ( -2.698458740408365879E-16, 1.000000000000000000, 0.000000000000000000 ) ) ;
#11155=LINE ( 'NONE', #20606, #11241 ) ;
#11156=EDGE_LOOP ( 'NONE', ( #16443, #3752, #345, #25322, #29750 ) ) ;
#11160=VECTOR ( 'NONE', #18041, 1000.000000000000000 ) ;
#11163=ORIENTED_EDGE ( 'NONE', *, *, #13650, .F. ) ;
#11172=ADVANCED_FACE ( 'NONE', ( #19594 ), #22189, .T. ) ;
#11174=CARTESIAN_POINT ( 'NONE',  ( 129.5152310637605524, -1.999999999999982236, -4.391296821672111328 ) ) ;
#11175=VECTOR ( 'NONE', #28239, 1000.000000000000000 ) ;
#11176=DIRECTION ( 'NONE',  ( -0.5877852522924731371, 0.000000000000000000, 0.8090169943749474513 ) ) ;
#11177=CARTESIAN_POINT ( 'NONE',  ( 166.1922820468853104, -9.999999999999998224, -2.083034168790677043 ) ) ;
#11181=ORIENTED_EDGE ( 'NONE', *, *, #24109, .F. ) ;
#11182=DIRECTION ( 'NONE',  ( -2.698458740408365879E-16, 1.000000000000000000, 0.000000000000000000 ) ) ;
#11183=EDGE_LOOP ( 'NONE', ( #10672, #2647, #6691, #1009 ) ) ;
#11186=CARTESIAN_POINT ( 'NONE',  ( 132.0152310637605808, -1.999999999999981348, -32.93883019725009120 ) ) ;
#11187=DIRECTION ( 'NONE',  ( -1.110223024625156540E-16, 0.000000000000000000, -1.000000000000000000 ) ) ;
#11189=ORIENTED_EDGE ( 'NONE', *, *, #24181, .T. ) ;
#11191=CARTESIAN_POINT ( 'NONE',  ( 173.6922820468853104, -9.999999999999994671, -17.92658477444275889 ) ) ;
#11196=FACE_OUTER_BOUND ( 'NONE', #19374, .T. ) ;
#11198=ORIENTED_EDGE ( 'NONE', *, *, #16704, .T. ) ;
#11200=LINE ( 'NONE', #8904, #14455 ) ;
#11201=VECTOR ( 'NONE', #27459, 1000.000000000000000 ) ;
#11204=VECTOR ( 'NONE', #6918, 1000.000000000000000 ) ;
#11206=VECTOR ( 'NONE', #29286, 1000.000000000000000 ) ;
#11207=ORIENTED_EDGE ( 'NONE', *, *, #1240, .T. ) ;
#11208=EDGE_LOOP ( 'NONE', ( #1527, #27183, #8472, #29878 ) ) ;
#11209=EDGE_CURVE ( 'NONE', #1955, #16958, #29109, .T. ) ;
#11210=EDGE_CURVE ( 'NONE', #6687, #26171, #29427, .T. ) ;
#11211=LINE ( 'NONE', #77, #21452 ) ;
#11212=EDGE_CURVE ( 'NONE', #18633, #2363, #15464, .T. ) ;
#11216=AXIS2_PLACEMENT_3D ( 'NONE', #27109, #1451, #5876 ) ;
#11217=DIRECTION ( 'NONE',  ( -0.5877852522924731371, -1.586114251531760728E-16, -0.8090169943749474513 ) ) ;
#11218=DIRECTION ( 'NONE',  ( 0.5877852522924731371, 1.586114251531760728E-16, 0.8090169943749474513 ) ) ;
#11219=LINE ( 'NONE', #11361, #10155 ) ;
#11223=ORIENTED_EDGE ( 'NONE', *, *, #8321, .T. ) ;
#11224=VECTOR ( 'NONE', #17362, 1000.000000000000000 ) ;
#11225=LINE ( 'NONE', #22221, #13914 ) ;
#11228=CARTESIAN_POINT ( 'NONE',  ( 148.6922820468854525, -10.00000000000000178, -23.73366926340167637 ) ) ;
#11230=FACE_OUTER_BOUND ( 'NONE', #23354, .T. ) ;
#11233=ORIENTED_EDGE ( 'NONE', *, *, #2925, .F. ) ;
#11234=CARTESIAN_POINT ( 'NONE',  ( 88.21376772083030460, -4.999999999999993783, -64.09105380476975711 ) ) ;
#11235=CARTESIAN_POINT ( 'NONE',  ( 129.5152310637605524, -10.00000000000000888, -30.37205893520530964 ) ) ;
#11236=LINE ( 'NONE', #27317, #13204 ) ;
#11241=VECTOR ( 'NONE', #20458, 1000.000000000000000 ) ;
#11243=CARTESIAN_POINT ( 'NONE',  ( 158.6922820468853956, -1.999999999999973577, -26.58683881228715862 ) ) ;
#11248=ADVANCED_FACE ( 'NONE', ( #5877 ), #15157, .T. ) ;
#11249=ORIENTED_EDGE ( 'NONE', *, *, #13183, .F. ) ;
#11250=EDGE_CURVE ( 'NONE', #19044, #15401, #3885, .T. ) ;
#11251=DIRECTION ( 'NONE',  ( 0.3090169943749475623, 8.338696094058001131E-17, 0.9510565162951536422 ) ) ;
#11252=CARTESIAN_POINT ( 'NONE',  ( 147.0152310637605240, -1.999999999999977129, -8.721423840594312082 ) ) ;
#11253=VERTEX_POINT ( 'NONE', #26804 ) ;
#11255=VECTOR ( 'NONE', #26995, 1000.000000000000000 ) ;
#11258=ORIENTED_EDGE ( 'NONE', *, *, #27588, .T. ) ;
#11259=VECTOR ( 'NONE', #18854, 1000.000000000000000 ) ;
#11265=CARTESIAN_POINT ( 'NONE',  ( 175.7287565553229456, -4.999999999999970690, 3.500000000000003109 ) ) ;
#11266=CARTESIAN_POINT ( 'NONE',  ( 162.0152310637604955, -4.999999999999974243, -1.798730398669517955E-14 ) ) ;
#11267=ORIENTED_EDGE ( 'NONE', *, *, #16565, .F. ) ;
#11268=CARTESIAN_POINT ( 'NONE',  ( 157.0152310637604387, -4.999999999999975131, -1.743219247438259497E-14 ) ) ;
#11270=VERTEX_POINT ( 'NONE', #19895 ) ;
#11271=VERTEX_POINT ( 'NONE', #6171 ) ;
#11272=DIRECTION ( 'NONE',  ( 0.9510565162951536422, 0.000000000000000000, -0.3090169943749475623 ) ) ;
#11273=ORIENTED_EDGE ( 'NONE', *, *, #9024, .T. ) ;
#11278=LINE ( 'NONE', #6259, #11608 ) ;
#11279=DIRECTION ( 'NONE',  ( -0.9510565162951536422, -2.566386769018988323E-16, 0.3090169943749475623 ) ) ;
#11280=ORIENTED_EDGE ( 'NONE', *, *, #24801, .F. ) ;
#11284=ORIENTED_EDGE ( 'NONE', *, *, #5545, .T. ) ;
#11285=EDGE_CURVE ( 'NONE', #9780, #209, #24638, .T. ) ;
#11286=EDGE_CURVE ( 'NONE', #9036, #1194, #24492, .T. ) ;
#11288=EDGE_CURVE ( 'NONE', #7265, #8429, #17752, .T. ) ;
#11289=CARTESIAN_POINT ( 'NONE',  ( 172.0152310637604387, -9.999999999999996447, -6.958068083716895558 ) ) ;
#11291=CARTESIAN_POINT ( 'NONE',  ( 159.7287565553229740, -4.999999999999974243, -25.16025403784441394 ) ) ;
#11292=DIRECTION ( 'NONE',  ( 0.5877852522924731371, 1.586114251531760728E-16, -0.8090169943749474513 ) ) ;
#11293=ORIENTED_EDGE ( 'NONE', *, *, #9443, .T. ) ;
#11294=DIRECTION ( 'NONE',  ( 2.698458740408365879E-16, -1.000000000000000000, 0.000000000000000000 ) ) ;
#11298=ORIENTED_EDGE ( 'NONE', *, *, #8956, .F. ) ;
#11300=ORIENTED_EDGE ( 'NONE', *, *, #22076, .T. ) ;
#11301=CARTESIAN_POINT ( 'NONE',  ( 143.6922820468854241, -1.999999999999978462, -9.266330736598359152 ) ) ;
#11303=CARTESIAN_POINT ( 'NONE',  ( 136.1922820468854241, -10.00000000000000533, -2.083034168790677043 ) ) ;
#11304=DIRECTION ( 'NONE',  ( 1.110223024625156540E-16, 2.995891024602366092E-32, 1.000000000000000000 ) ) ;
#11305=ORIENTED_EDGE ( 'NONE', *, *, #4950, .T. ) ;
#11306=CARTESIAN_POINT ( 'NONE',  ( 141.1922820468854241, -1.999999999999979128, -4.936203717676158398 ) ) ;
#11307=ORIENTED_EDGE ( 'NONE', *, *, #15650, .F. ) ;
#11311=LINE ( 'NONE', #22778, #2367 ) ;
#11315=ADVANCED_FACE ( 'NONE', ( #29882 ), #15619, .T. ) ;
#11316=VECTOR ( 'NONE', #11279, 999.9999999999998863 ) ;
#11317=EDGE_CURVE ( 'NONE', #17166, #1955, #27273, .T. ) ;
#11318=EDGE_CURVE ( 'NONE', #9904, #5737, #20496, .T. ) ;
#11319=EDGE_LOOP ( 'NONE', ( #12935, #20895, #2403, #20897 ) ) ;
#11321=CARTESIAN_POINT ( 'NONE',  ( 173.6922820468853104, -1.999999999999970024, -17.92658477444275889 ) ) ;
#11322=DIRECTION ( 'NONE',  ( -2.908569913943825554E-16, 1.000000000000000000, -0.000000000000000000 ) ) ;
#11324=CARTESIAN_POINT ( 'NONE',  ( 157.0152310637605524, -1.999999999999973133, -34.70218595412750773 ) ) ;
#11328=EDGE_LOOP ( 'NONE', ( #13836, #27685, #5544, #8761 ) ) ;
#11330=ORIENTED_EDGE ( 'NONE', *, *, #27690, .T. ) ;
#11334=CARTESIAN_POINT ( 'NONE',  ( 134.5152310637605808, -10.00000000000000533, -19.94844914048349338 ) ) ;
#11337=VERTEX_POINT ( 'NONE', #13472 ) ;
#11338=VERTEX_POINT ( 'NONE', #8890 ) ;
#11339=CARTESIAN_POINT ( 'NONE',  ( 156.1922820468853672, -10.00000000000000000, -10.74328820663507678 ) ) ;
#11341=EDGE_CURVE ( 'NONE', #29240, #17052, #11475, .T. ) ;
#11342=ORIENTED_EDGE ( 'NONE', *, *, #27322, .T. ) ;
#11348=ORIENTED_EDGE ( 'NONE', *, *, #5297, .T. ) ;
#11353=ORIENTED_EDGE ( 'NONE', *, *, #26218, .T. ) ;
#11354=CARTESIAN_POINT ( 'NONE',  ( 23.56128742750157201, -5.000000000000011546, -72.51418643027592736 ) ) ;
#11355=CIRCLE ( 'NONE', #28466, 5.999999999999977796 ) ;
#11357=ORIENTED_EDGE ( 'NONE', *, *, #3151, .F. ) ;
#11358=PLANE ( 'NONE',  #29801 ) ;
#11359=DIRECTION ( 'NONE',  ( 0.9510565162951535312, 2.566386769018988816E-16, -0.3090169943749475623 ) ) ;
#11360=CARTESIAN_POINT ( 'NONE',  ( 138.6922820468854525, -4.999999999999980460, -6.413161187712876909 ) ) ;
#11361=CARTESIAN_POINT ( 'NONE',  ( 111.0562616426541069, -4.999999999999986677, 80.68709708467871167 ) ) ;
#11364=AXIS2_PLACEMENT_3D ( 'NONE', #1110, #3538, #24146 ) ;
#11366=VERTEX_POINT ( 'NONE', #15764 ) ;
#11369=LINE ( 'NONE', #20674, #16644 ) ;
#11370=CARTESIAN_POINT ( 'NONE',  ( 148.6922820468853956, -1.999999999999977129, -9.266330736598359152 ) ) ;
#11374=CARTESIAN_POINT ( 'NONE',  ( 130.7287565553229172, -10.00000000000000888, -28.21440484423856532 ) ) ;
#11376=EDGE_CURVE ( 'NONE', #10549, #2849, #13327, .T. ) ;
#11377=ORIENTED_EDGE ( 'NONE', *, *, #18173, .F. ) ;
#11378=LINE ( 'NONE', #20681, #5168 ) ;
#11380=FACE_OUTER_BOUND ( 'NONE', #29285, .T. ) ;
#11382=ORIENTED_EDGE ( 'NONE', *, *, #6056, .F. ) ;
#11389=ORIENTED_EDGE ( 'NONE', *, *, #24357, .F. ) ;
#11390=LINE ( 'NONE', #6834, #8421 ) ;
#11391=DIRECTION ( 'NONE',  ( -2.698458740408365879E-16, 1.000000000000000000, 0.000000000000000000 ) ) ;
#11392=ORIENTED_EDGE ( 'NONE', *, *, #10002, .T. ) ;
#11393=DIRECTION ( 'NONE',  ( -2.698458740408365879E-16, 1.000000000000000000, 0.000000000000000000 ) ) ;
#11395=DIRECTION ( 'NONE',  ( -1.110223024625156540E-16, 0.000000000000000000, -1.000000000000000000 ) ) ;
#11398=ORIENTED_EDGE ( 'NONE', *, *, #22076, .F. ) ;
#11400=CARTESIAN_POINT ( 'NONE',  ( 149.5152310637605240, -4.999999999999976907, -13.05155085951651195 ) ) ;
#11402=DIRECTION ( 'NONE',  ( 0.9510565162951535312, 2.566386769018988816E-16, -0.3090169943749475623 ) ) ;
#11403=DIRECTION ( 'NONE',  ( -0.8090169943749474513, -2.183098979609982436E-16, -0.5877852522924731371 ) ) ;
#11405=EDGE_CURVE ( 'NONE', #13495, #10404, #29732, .T. ) ;
#11407=DIRECTION ( 'NONE',  ( 0.5877852522924731371, 1.586114251531760728E-16, 0.8090169943749474513 ) ) ;
#11409=ADVANCED_FACE ( 'NONE', ( #22955 ), #24951, .T. ) ;
#11411=ORIENTED_EDGE ( 'NONE', *, *, #19484, .T. ) ;
#11412=EDGE_CURVE ( 'NONE', #2849, #4933, #8740, .T. ) ;
#11413=LINE ( 'NONE', #28250, #15926 ) ;
#11414=ORIENTED_EDGE ( 'NONE', *, *, #13691, .F. ) ;
#11421=FACE_OUTER_BOUND ( 'NONE', #3041, .T. ) ;
#11425=CARTESIAN_POINT ( 'NONE',  ( 17.03854528076240271, -5.000000000000013323, -52.43925030801758425 ) ) ;
#11426=EDGE_CURVE ( 'NONE', #28060, #3594, #25533, .T. ) ;
#11429=FACE_OUTER_BOUND ( 'NONE', #20428, .T. ) ;
#11430=ORIENTED_EDGE ( 'NONE', *, *, #22792, .T. ) ;
#11431=EDGE_LOOP ( 'NONE', ( #28899, #14449, #29580, #20756, #22437 ) ) ;
#11432=CARTESIAN_POINT ( 'NONE',  ( 12.58835545445038306, -5.000000000000014211, 38.74297434227223391 ) ) ;
#11433=VECTOR ( 'NONE', #29563, 1000.000000000000000 ) ;
#11437=EDGE_LOOP ( 'NONE', ( #23133, #23042, #8930, #10543 ) ) ;
#11438=VERTEX_POINT ( 'NONE', #10883 ) ;
#11440=EDGE_CURVE ( 'NONE', #21937, #19636, #15910, .T. ) ;
#11443=LINE ( 'NONE', #15730, #19837 ) ;
#11446=ORIENTED_EDGE ( 'NONE', *, *, #18894, .F. ) ;
#11447=CARTESIAN_POINT ( 'NONE',  ( 149.5152310637606092, -1.999999999999975353, -28.60870317832789667 ) ) ;
#11448=VERTEX_POINT ( 'NONE', #4033 ) ;
#11452=PLANE ( 'NONE',  #17921 ) ;
#11453=LINE ( 'NONE', #20764, #26438 ) ;
#11457=VERTEX_POINT ( 'NONE', #18057 ) ;
#11458=CARTESIAN_POINT ( 'NONE',  ( 166.1922820468853388, -1.999999999999972244, -10.74328820663507678 ) ) ;
#11459=DIRECTION ( 'NONE',  ( -2.698458740408365879E-16, 1.000000000000000000, 0.000000000000000000 ) ) ;
#11462=CARTESIAN_POINT ( 'NONE',  ( 154.5152310637605524, -1.999999999999974021, -30.37205893520531319 ) ) ;
#11463=VECTOR ( 'NONE', #29310, 1000.000000000000000 ) ;
#11471=EDGE_CURVE ( 'NONE', #5728, #23514, #27870, .T. ) ;
#11474=LINE ( 'NONE', #11334, #24897 ) ;
#11475=LINE ( 'NONE', #20792, #21042 ) ;
#11476=EDGE_CURVE ( 'NONE', #23604, #21626, #16219, .T. ) ;
#11479=ORIENTED_EDGE ( 'NONE', *, *, #20647, .T. ) ;
#11480=CARTESIAN_POINT ( 'NONE',  ( 16.56108776669977090, -5.000000000000013323, -50.96978717728640618 ) ) ;
#11481=EDGE_CURVE ( 'NONE', #12783, #18704, #22507, .T. ) ;
#11483=ORIENTED_EDGE ( 'NONE', *, *, #11724, .F. ) ;
#11485=FACE_OUTER_BOUND ( 'NONE', #25634, .T. ) ;
#11486=DIRECTION ( 'NONE',  ( -0.8090169943749474513, -2.183098979609982436E-16, -0.5877852522924731371 ) ) ;
#11489=CARTESIAN_POINT ( 'NONE',  ( 176.1922820468853104, -1.999999999999969358, -22.25671179336496053 ) ) ;
#11490=ORIENTED_EDGE ( 'NONE', *, *, #24414, .F. ) ;
#11494=VECTOR ( 'NONE', #26688, 1000.000000000000000 ) ;
#11495=ORIENTED_EDGE ( 'NONE', *, *, #25327, .T. ) ;
#11496=CARTESIAN_POINT ( 'NONE',  ( 166.1922820468853672, -9.999999999999996447, -28.06379628232387802 ) ) ;
#11499=VERTEX_POINT ( 'NONE', #29577 ) ;
#11500=LINE ( 'NONE', #20812, #17351 ) ;
#11502=CARTESIAN_POINT ( 'NONE',  ( 158.6922820468853388, -1.999999999999974021, -15.07341522555727664 ) ) ;
#11507=CARTESIAN_POINT ( 'NONE',  ( 117.3538932196093185, -4.999999999999985789, -85.26259425104612433 ) ) ;
#11509=AXIS2_PLACEMENT_3D ( 'NONE', #10858, #17868, #6295 ) ;
#11510=LINE ( 'NONE', #4513, #24919 ) ;
#11511=CARTESIAN_POINT ( 'NONE',  ( 137.0152310637606092, -1.999999999999979572, -24.27857615940569147 ) ) ;
#11516=EDGE_CURVE ( 'NONE', #13920, #26554, #23398, .T. ) ;
#11518=VERTEX_POINT ( 'NONE', #2515 ) ;
#11519=VECTOR ( 'NONE', #4182, 1000.000000000000000 ) ;
#11521=CARTESIAN_POINT ( 'NONE',  ( 131.1922820468854241, -10.00000000000000888, -4.936203717676158398 ) ) ;
#11524=ORIENTED_EDGE ( 'NONE', *, *, #14811, .F. ) ;
#11525=ORIENTED_EDGE ( 'NONE', *, *, #25146, .F. ) ;
#11538=EDGE_LOOP ( 'NONE', ( #18059, #15180, #16182, #19808 ) ) ;
#11539=CARTESIAN_POINT ( 'NONE',  ( 137.0152310637606092, -4.999999999999980460, -6.958068083716895558 ) ) ;
#11543=ORIENTED_EDGE ( 'NONE', *, *, #17441, .T. ) ;
#11544=CARTESIAN_POINT ( 'NONE',  ( 162.0152310637604387, -9.999999999999998224, 1.702185954127501066 ) ) ;
#11547=DIRECTION ( 'NONE',  ( 0.3090169943749475623, 8.338696094058001131E-17, 0.9510565162951536422 ) ) ;
#11548=ORIENTED_EDGE ( 'NONE', *, *, #5896, .T. ) ;
#11549=LINE ( 'NONE', #23164, #22210 ) ;
#11550=VERTEX_POINT ( 'NONE', #19114 ) ;
#11551=CARTESIAN_POINT ( 'NONE',  ( 154.5152310637604955, -10.00000000000000178, -2.627941064794695691 ) ) ;
#11553=LINE ( 'NONE', #18281, #3498 ) ;
#11555=FACE_OUTER_BOUND ( 'NONE', #25813, .T. ) ;
#11556=EDGE_LOOP ( 'NONE', ( #23885, #25054, #13128, #26538 ) ) ;
#11558=VECTOR ( 'NONE', #16291, 1000.000000000000000 ) ;
#11561=ORIENTED_EDGE ( 'NONE', *, *, #24531, .F. ) ;
#11563=DIRECTION ( 'NONE',  ( -0.9510565162951536422, -2.566386769018988323E-16, 0.3090169943749475623 ) ) ;
#11564=DIRECTION ( 'NONE',  ( 0.9510565162951536422, 2.566386769018988816E-16, 0.3090169943749472292 ) ) ;
#11565=CARTESIAN_POINT ( 'NONE',  ( 158.6922820468853956, -9.999999999999998224, -23.73366926340167637 ) ) ;
#11567=LINE ( 'NONE', #28498, #9670 ) ;
#11568=EDGE_CURVE ( 'NONE', #26251, #5568, #28322, .T. ) ;
#11569=CARTESIAN_POINT ( 'NONE',  ( 158.6922820468853672, -10.00000000000000000, -17.92658477444275889 ) ) ;
#11570=EDGE_CURVE ( 'NONE', #28726, #23960, #13917, .T. ) ;
#11571=FACE_OUTER_BOUND ( 'NONE', #7785, .T. ) ;
#11572=EDGE_CURVE ( 'NONE', #2975, #10405, #510, .T. ) ;
#11573=VECTOR ( 'NONE', #21392, 1000.000000000000000 ) ;
#11574=PLANE ( 'NONE',  #24885 ) ;
#11575=DIRECTION ( 'NONE',  ( -0.8090169943749474513, -2.183098979609982436E-16, 0.5877852522924731371 ) ) ;
#11576=EDGE_CURVE ( 'NONE', #29180, #14702, #9799, .T. ) ;
#11578=CARTESIAN_POINT ( 'NONE',  ( 164.7287565553229456, -9.999999999999998224, -25.16025403784440329 ) ) ;
#11579=DIRECTION ( 'NONE',  ( 0.3090169943749475623, 8.338696094058001131E-17, 0.9510565162951536422 ) ) ;
#11580=VECTOR ( 'NONE', #17724, 1000.000000000000000 ) ;
#11583=ORIENTED_EDGE ( 'NONE', *, *, #19774, .T. ) ;
#11584=CARTESIAN_POINT ( 'NONE',  ( 164.5152310637604955, -4.999999999999973355, -19.94844914048349693 ) ) ;
#11589=EDGE_LOOP ( 'NONE', ( #5098, #8227, #7156, #19467 ) ) ;
#11592=LINE ( 'NONE', #22505, #12561 ) ;
#11594=DIRECTION ( 'NONE',  ( -0.8090169943749474513, -2.183098979609982436E-16, -0.5877852522924731371 ) ) ;
#11595=LINE ( 'NONE', #2477, #26229 ) ;
#11596=EDGE_LOOP ( 'NONE', ( #28165, #20978, #20956, #21821, #2667 ) ) ;
#11602=ORIENTED_EDGE ( 'NONE', *, *, #26601, .F. ) ;
#11604=DIRECTION ( 'NONE',  ( -0.5877852522924731371, 0.000000000000000000, 0.8090169943749474513 ) ) ;
#11608=VECTOR ( 'NONE', #20585, 1000.000000000000000 ) ;
#11612=CARTESIAN_POINT ( 'NONE',  ( 157.0152310637605240, -9.999999999999998224, -26.04193191628311155 ) ) ;
#11613=EDGE_CURVE ( 'NONE', #29774, #7167, #14520, .T. ) ;
#11615=EDGE_CURVE ( 'NONE', #11457, #2772, #7517, .T. ) ;
#11617=EDGE_CURVE ( 'NONE', #25465, #5840, #23863, .T. ) ;
#11618=EDGE_LOOP ( 'NONE', ( #29498, #6490, #24341, #13022 ) ) ;
#11619=DIRECTION ( 'NONE',  ( 0.3090169943749472292, 8.338696094057992503E-17, -0.9510565162951536422 ) ) ;
#11620=FACE_OUTER_BOUND ( 'NONE', #5287, .T. ) ;
#11621=DIRECTION ( 'NONE',  ( -2.698458740408365879E-16, 1.000000000000000000, 0.000000000000000000 ) ) ;
#11622=UNCERTAINTY_MEASURE_WITH_UNIT (LENGTH_MEASURE( 1.000000000000000082E-05 ), #29747, 'distance_accuracy_value', 'NONE');
#11625=VECTOR ( 'NONE', #731, 1000.000000000000000 ) ;
#11626=FACE_OUTER_BOUND ( 'NONE', #29283, .T. ) ;
#11627=ORIENTED_EDGE ( 'NONE', *, *, #892, .F. ) ;
#11630=CARTESIAN_POINT ( 'NONE',  ( 12.03194932440650966, -5.000000000000014211, 37.03053235585281300 ) ) ;
#11631=DIRECTION ( 'NONE',  ( -2.698458740408365879E-16, 1.000000000000000000, 0.000000000000000000 ) ) ;
#11633=ORIENTED_EDGE ( 'NONE', *, *, #15559, .F. ) ;
#11634=VECTOR ( 'NONE', #24473, 1000.000000000000000 ) ;
#11635=ORIENTED_EDGE ( 'NONE', *, *, #6513, .F. ) ;
#11636=DIRECTION ( 'NONE',  ( -0.9510565162951536422, -2.566386769018988816E-16, -0.3090169943749472292 ) ) ;
#11641=DIRECTION ( 'NONE',  ( 0.000000000000000000, 0.000000000000000000, -1.000000000000000000 ) ) ;
#11642=DIRECTION ( 'NONE',  ( 1.000000000000000000, 2.698458740408365879E-16, -1.110223024625156540E-16 ) ) ;
#11645=CARTESIAN_POINT ( 'NONE',  ( 142.0152310637605808, -4.999999999999978684, -6.958068083716895558 ) ) ;
#11649=FACE_OUTER_BOUND ( 'NONE', #16752, .T. ) ;
#11650=AXIS2_PLACEMENT_3D ( 'NONE', #29206, #8246, #26909 ) ;
#11652=EDGE_CURVE ( 'NONE', #8269, #10703, #20944, .T. ) ;
#11653=ADVANCED_FACE ( 'NONE', ( #2653 ), #28169, .T. ) ;
#11656=EDGE_CURVE ( 'NONE', #319, #15181, #11928, .T. ) ;
#11658=CARTESIAN_POINT ( 'NONE',  ( 142.0152310637605524, -1.999999999999978462, -8.721423840594312082 ) ) ;
#11659=FACE_OUTER_BOUND ( 'NONE', #2224, .T. ) ;
#11664=EDGE_LOOP ( 'NONE', ( #30136, #1644, #29797, #24089 ) ) ;
#11670=VERTEX_POINT ( 'NONE', #7381 ) ;
#11671=DIRECTION ( 'NONE',  ( 0.9510565162951536422, 0.000000000000000000, -0.3090169943749475623 ) ) ;
#11673=VERTEX_POINT ( 'NONE', #362 ) ;
#11675=DIRECTION ( 'NONE',  ( -2.698458740408365879E-16, 1.000000000000000000, 0.000000000000000000 ) ) ;
#11677=ORIENTED_EDGE ( 'NONE', *, *, #23632, .F. ) ;
#11678=VECTOR ( 'NONE', #8810, 1000.000000000000000 ) ;
#11681=VERTEX_POINT ( 'NONE', #16522 ) ;
#11687=EDGE_CURVE ( 'NONE', #23514, #3855, #5533, .T. ) ;
#11688=ORIENTED_EDGE ( 'NONE', *, *, #2346, .T. ) ;
#11694=DIRECTION ( 'NONE',  ( -2.698458740408365879E-16, 1.000000000000000000, 0.000000000000000000 ) ) ;
#11695=ORIENTED_EDGE ( 'NONE', *, *, #25044, .F. ) ;
#11696=EDGE_LOOP ( 'NONE', ( #2415, #29943, #8469, #4056, #24123 ) ) ;
#11697=FACE_OUTER_BOUND ( 'NONE', #8382, .T. ) ;
#11698=LINE ( 'NONE', #9400, #24863 ) ;
#11702=PLANE ( 'NONE',  #20488 ) ;
#11703=PLANE ( 'NONE',  #12824 ) ;
#11706=DIRECTION ( 'NONE',  ( -0.9510565162951536422, 0.000000000000000000, -0.3090169943749472292 ) ) ;
#11708=VERTEX_POINT ( 'NONE', #20015 ) ;
#11709=AXIS2_PLACEMENT_3D ( 'NONE', #22954, #20639, #16974 ) ;
#11710=DIRECTION ( 'NONE',  ( -1.110223024625156540E-16, 0.000000000000000000, -1.000000000000000000 ) ) ;
#11713=ORIENTED_EDGE ( 'NONE', *, *, #5368, .F. ) ;
#11715=ADVANCED_FACE ( 'NONE', ( #961 ), #12533, .T. ) ;
#11716=VECTOR ( 'NONE', #23188, 1000.000000000000000 ) ;
#11720=CARTESIAN_POINT ( 'NONE',  ( 167.2287565553229740, -1.999999999999970468, -29.49038105676660493 ) ) ;
#11721=CARTESIAN_POINT ( 'NONE',  ( 174.5152310637604671, -9.999999999999994671, -19.94844914048349693 ) ) ;
#11722=CARTESIAN_POINT ( 'NONE',  ( 159.7287565553230024, -1.999999999999972244, -33.82050807568879947 ) ) ;
#11724=EDGE_CURVE ( 'NONE', #6838, #6429, #24602, .T. ) ;
#11727=CARTESIAN_POINT ( 'NONE',  ( 144.5152310637605808, -4.999999999999978684, -21.71180489736091346 ) ) ;
#11729=VECTOR ( 'NONE', #19631, 1000.000000000000000 ) ;
#11730=CARTESIAN_POINT ( 'NONE',  ( 15.68512135455575596, -5.000000000000013323, -48.27383977151229999 ) ) ;
#11731=LINE ( 'NONE', #4870, #8949 ) ;
#11734=VERTEX_POINT ( 'NONE', #19705 ) ;
#11736=ORIENTED_EDGE ( 'NONE', *, *, #1203, .T. ) ;
#11738=ORIENTED_EDGE ( 'NONE', *, *, #4234, .F. ) ;
#11739=CARTESIAN_POINT ( 'NONE',  ( 142.0152310637605808, -10.00000000000000355, -34.70218595412750773 ) ) ;
#11742=PLANE ( 'NONE',  #21428 ) ;
#11743=EDGE_LOOP ( 'NONE', ( #26825, #1585, #15044, #26007 ) ) ;
#11745=VERTEX_POINT ( 'NONE', #10706 ) ;
#11747=DIRECTION ( 'NONE',  ( -2.698458740408365879E-16, 1.000000000000000000, 0.000000000000000000 ) ) ;
#11749=CARTESIAN_POINT ( 'NONE',  ( 4.317446301598349301, -5.000000000000016875, 13.28773340506741896 ) ) ;
#11750=DIRECTION ( 'NONE',  ( 0.9510565162951536422, 0.000000000000000000, -0.3090169943749475623 ) ) ;
#11751=VERTEX_POINT ( 'NONE', #8409 ) ;
#11752=CARTESIAN_POINT ( 'NONE',  ( 133.6922820468854241, -1.999999999999981348, -17.92658477444275533 ) ) ;
#11755=EDGE_CURVE ( 'NONE', #1753, #2498, #10547, .T. ) ;
#11756=ORIENTED_EDGE ( 'NONE', *, *, #7531, .F. ) ;
#11758=VECTOR ( 'NONE', #25893, 1000.000000000000000 ) ;
#11760=ADVANCED_FACE ( 'NONE', ( #26300 ), #5833, .T. ) ;
#11767=ORIENTED_EDGE ( 'NONE', *, *, #24908, .F. ) ;
#11768=FACE_BOUND ( 'NONE', #3639, .T. ) ;
#11769=VECTOR ( 'NONE', #11187, 1000.000000000000000 ) ;
#11770=CARTESIAN_POINT ( 'NONE',  ( 169.5152310637604671, -1.999999999999970468, -21.71180489736091346 ) ) ;
#11771=LINE ( 'NONE', #16963, #22393 ) ;
#11772=CARTESIAN_POINT ( 'NONE',  ( 9.964222036193500998, -5.000000000000015099, 30.66672212155160793 ) ) ;
#11774=LINE ( 'NONE', #7217, #10930 ) ;
#11776=ORIENTED_EDGE ( 'NONE', *, *, #29652, .F. ) ;
#11778=EDGE_LOOP ( 'NONE', ( #4115, #25925, #15484, #19634 ) ) ;
#11781=CARTESIAN_POINT ( 'NONE',  ( 13.46432186659439800, -5.000000000000014211, 41.43892174804634010 ) ) ;
#11782=CARTESIAN_POINT ( 'NONE',  ( 13.13993655228012436, -5.000000000000014211, -40.44056640647991685 ) ) ;
#11783=VERTEX_POINT ( 'NONE', #26452 ) ;
#11785=ORIENTED_EDGE ( 'NONE', *, *, #12252, .T. ) ;
#11786=DIRECTION ( 'NONE',  ( -0.5877852522924731371, 0.000000000000000000, 0.8090169943749474513 ) ) ;
#11788=ORIENTED_EDGE ( 'NONE', *, *, #18593, .F. ) ;
#11789=EDGE_CURVE ( 'NONE', #23642, #1088, #19855, .T. ) ;
#11792=EDGE_CURVE ( 'NONE', #18131, #27161, #24452, .T. ) ;
#11793=CARTESIAN_POINT ( 'NONE',  ( 130.7287565553229172, -4.999999999999983125, -22.10610323145025902 ) ) ;
#11798=FACE_OUTER_BOUND ( 'NONE', #25671, .T. ) ;
#11801=EDGE_LOOP ( 'NONE', ( #10398, #6919, #11233, #20175 ) ) ;
#11802=ORIENTED_EDGE ( 'NONE', *, *, #29888, .F. ) ;
#11804=VECTOR ( 'NONE', #1891, 1000.000000000000000 ) ;
#11805=CARTESIAN_POINT ( 'NONE',  ( 167.2287565553228887, -9.999999999999998224, -3.509618943233403510 ) ) ;
#11806=LINE ( 'NONE', #21123, #2261 ) ;
#11808=ORIENTED_EDGE ( 'NONE', *, *, #23802, .T. ) ;
#11810=VECTOR ( 'NONE', #18258, 1000.000000000000000 ) ;
#11814=EDGE_CURVE ( 'NONE', #18644, #6532, #19558, .T. ) ;
#11817=CARTESIAN_POINT ( 'NONE',  ( 9.009307008068239142, -5.000000000000015099, 27.72779586008924468 ) ) ;
#11818=DIRECTION ( 'NONE',  ( 0.9510565162951535312, 2.566386769018988816E-16, -0.3090169943749475623 ) ) ;
#11819=LINE ( 'NONE', #19003, #2534 ) ;
#11820=DIRECTION ( 'NONE',  ( -2.698458740408365879E-16, 1.000000000000000000, 0.000000000000000000 ) ) ;
#11822=ORIENTED_EDGE ( 'NONE', *, *, #13011, .F. ) ;
#11823=PLANE ( 'NONE',  #20758 ) ;
#11825=VERTEX_POINT ( 'NONE', #19406 ) ;
#11826=CARTESIAN_POINT ( 'NONE',  ( 144.5152310637605808, -4.999999999999978684, -1.604441369360116507E-14 ) ) ;
#11827=DIRECTION ( 'NONE',  ( -0.9510565162951536422, 0.000000000000000000, -0.3090169943749472292 ) ) ;
#11828=EDGE_CURVE ( 'NONE', #13853, #8269, #14967, .T. ) ;
#11830=EDGE_CURVE ( 'NONE', #28906, #11448, #803, .T. ) ;
#11833=VERTEX_POINT ( 'NONE', #22469 ) ;
#11834=EDGE_CURVE ( 'NONE', #25350, #11270, #2023, .T. ) ;
#11838=AXIS2_PLACEMENT_3D ( 'NONE', #21800, #19501, #28871 ) ;
#11841=ORIENTED_EDGE ( 'NONE', *, *, #5635, .F. ) ;
#11844=CARTESIAN_POINT ( 'NONE',  ( 133.6922820468854241, -1.999999999999981348, -26.58683881228715506 ) ) ;
#11845=DIRECTION ( 'NONE',  ( 1.110223024625156540E-16, 2.995891024602366092E-32, 1.000000000000000000 ) ) ;
#11849=ORIENTED_EDGE ( 'NONE', *, *, #15593, .T. ) ;
#11850=AXIS2_PLACEMENT_3D ( 'NONE', #18080, #4204, #27441 ) ;
#11851=CARTESIAN_POINT ( 'NONE',  ( 172.7287565553229456, -1.999999999999970468, 6.499999999999977796 ) ) ;
#11852=CARTESIAN_POINT ( 'NONE',  ( 149.5152310637605240, -1.999999999999976685, -2.627941064794695691 ) ) ;
#11854=DIRECTION ( 'NONE',  ( 0.5877852522924731371, 1.586114251531760728E-16, -0.8090169943749474513 ) ) ;
#11855=ORIENTED_EDGE ( 'NONE', *, *, #26747, .F. ) ;
#11857=VERTEX_POINT ( 'NONE', #25206 ) ;
#11859=ADVANCED_FACE ( 'NONE', ( #9000 ), #8856, .T. ) ;
#11860=DIRECTION ( 'NONE',  ( -0.8090169943749474513, -2.183098979609982436E-16, 0.5877852522924731371 ) ) ;
#11861=EDGE_CURVE ( 'NONE', #12653, #15277, #13140, .T. ) ;
#11862=CARTESIAN_POINT ( 'NONE',  ( 173.6922820468852819, -1.999999999999970024, -15.07341522555727664 ) ) ;
#11863=VERTEX_POINT ( 'NONE', #22614 ) ;
#11864=EDGE_CURVE ( 'NONE', #23355, #18808, #16030, .T. ) ;
#11868=LINE ( 'NONE', #11720, #12568 ) ;
#11869=LINE ( 'NONE', #1726, #29235 ) ;
#11870=CARTESIAN_POINT ( 'NONE',  ( 158.6922820468853104, -10.00000000000000000, 2.247092850131519715 ) ) ;
#11872=VECTOR ( 'NONE', #25788, 1000.000000000000000 ) ;
#11873=ORIENTED_EDGE ( 'NONE', *, *, #20443, .T. ) ;
#11874=CARTESIAN_POINT ( 'NONE',  ( 169.7287565553228603, -4.999999999999971578, 0.8205080756888000204 ) ) ;
#11875=CARTESIAN_POINT ( 'NONE',  ( 131.1922820468854241, -10.00000000000000888, -10.74328820663507322 ) ) ;
#11876=FACE_OUTER_BOUND ( 'NONE', #4187, .T. ) ;
#11877=PLANE ( 'NONE',  #28990 ) ;
#11879=EDGE_CURVE ( 'NONE', #28015, #17495, #11443, .T. ) ;
#11880=LINE ( 'NONE', #7174, #29713 ) ;
#11884=EDGE_LOOP ( 'NONE', ( #2803, #19577, #18428, #25733 ) ) ;
#11888=FACE_BOUND ( 'NONE', #25094, .T. ) ;
#11889=ORIENTED_EDGE ( 'NONE', *, *, #12215, .F. ) ;
#11891=PLANE ( 'NONE',  #27242 ) ;
#11892=VECTOR ( 'NONE', #3760, 1000.000000000000000 ) ;
#11894=DIRECTION ( 'NONE',  ( -0.9510565162951536422, -2.566386769018988816E-16, -0.3090169943749472292 ) ) ;
#11895=PLANE ( 'NONE',  #24260 ) ;
#11896=ORIENTED_EDGE ( 'NONE', *, *, #11830, .F. ) ;
#11897=DIRECTION ( 'NONE',  ( 1.000000000000000000, 2.698458740408365879E-16, -1.110223024625156540E-16 ) ) ;
#11898=VERTEX_POINT ( 'NONE', #25354 ) ;
#11901=ORIENTED_EDGE ( 'NONE', *, *, #776, .T. ) ;
#11905=ORIENTED_EDGE ( 'NONE', *, *, #15553, .F. ) ;
#11906=DIRECTION ( 'NONE',  ( -0.9510565162951536422, 0.000000000000000000, -0.3090169943749472292 ) ) ;
#11907=LINE ( 'NONE', #12063, #5472 ) ;
#11911=DIRECTION ( 'NONE',  ( -2.698458740408366372E-16, 1.000000000000000000, 0.000000000000000000 ) ) ;
#11912=VECTOR ( 'NONE', #11955, 1000.000000000000000 ) ;
#11913=EDGE_LOOP ( 'NONE', ( #1234, #15250, #7742, #17267, #2622 ) ) ;
#11914=EDGE_CURVE ( 'NONE', #11708, #8986, #27233, .T. ) ;
#11915=FACE_OUTER_BOUND ( 'NONE', #14099, .T. ) ;
#11916=CARTESIAN_POINT ( 'NONE',  ( 173.6922820468852819, -9.999999999999996447, -9.266330736598359152 ) ) ;
#11918=DIRECTION ( 'NONE',  ( -2.698458740408365879E-16, 1.000000000000000000, 0.000000000000000000 ) ) ;
#11921=DIRECTION ( 'NONE',  ( 1.000000000000000000, 2.698458740408365879E-16, -1.110223024625156540E-16 ) ) ;
#11922=CARTESIAN_POINT ( 'NONE',  ( 137.0152310637605808, -10.00000000000000533, -26.04193191628310800 ) ) ;
#11923=ORIENTED_EDGE ( 'NONE', *, *, #6710, .F. ) ;
#11928=LINE ( 'NONE', #658, #13968 ) ;
#11930=ORIENTED_EDGE ( 'NONE', *, *, #16100, .T. ) ;
#11931=CARTESIAN_POINT ( 'NONE',  ( 163.6922820468853956, -9.999999999999998224, -32.39392330124607611 ) ) ;
#11937=ORIENTED_EDGE ( 'NONE', *, *, #8038, .T. ) ;
#11938=AXIS2_PLACEMENT_3D ( 'NONE', #11739, #7619, #21198 ) ;
#11939=DIRECTION ( 'NONE',  ( 0.9510565162951535312, 2.566386769018988816E-16, -0.3090169943749475623 ) ) ;
#11941=ORIENTED_EDGE ( 'NONE', *, *, #7572, .T. ) ;
#11945=ORIENTED_EDGE ( 'NONE', *, *, #29078, .T. ) ;
#11946=ORIENTED_EDGE ( 'NONE', *, *, #12929, .F. ) ;
#11947=DIRECTION ( 'NONE',  ( 0.9510565162951536422, 2.566386769018988816E-16, 0.3090169943749472292 ) ) ;
#11948=FACE_OUTER_BOUND ( 'NONE', #3580, .T. ) ;
#11949=EDGE_CURVE ( 'NONE', #600, #26457, #13295, .T. ) ;
#11951=CARTESIAN_POINT ( 'NONE',  ( 154.7287565553229172, -4.999999999999975131, 0.8205080756888000204 ) ) ;
#11953=VECTOR ( 'NONE', #24532, 1000.000000000000000 ) ;
#11954=EDGE_CURVE ( 'NONE', #12367, #29073, #9111, .T. ) ;
#11955=DIRECTION ( 'NONE',  ( -0.5877852522924731371, -1.586114251531760728E-16, -0.8090169943749474513 ) ) ;
#11956=VERTEX_POINT ( 'NONE', #13742 ) ;
#11957=VECTOR ( 'NONE', #27453, 1000.000000000000000 ) ;
#11963=VERTEX_POINT ( 'NONE', #8706 ) ;
#11965=CARTESIAN_POINT ( 'NONE',  ( 146.1922820468854241, -10.00000000000000355, -13.59645775552055902 ) ) ;
#11966=CARTESIAN_POINT ( 'NONE',  ( 162.2287565553229456, -1.999999999999972244, -20.83012701892220520 ) ) ;
#11968=VERTEX_POINT ( 'NONE', #17716 ) ;
#11971=VECTOR ( 'NONE', #6962, 1000.000000000000000 ) ;
#11972=ORIENTED_EDGE ( 'NONE', *, *, #6479, .F. ) ;
#11973=CARTESIAN_POINT ( 'NONE',  ( 159.5152310637605240, -9.999999999999998224, -30.37205893520531319 ) ) ;
#11977=VERTEX_POINT ( 'NONE', #15875 ) ;
#11979=ORIENTED_EDGE ( 'NONE', *, *, #18265, .T. ) ;
#11982=VECTOR ( 'NONE', #2688, 1000.000000000000000 ) ;
#11987=VERTEX_POINT ( 'NONE', #4297 ) ;
#11989=ADVANCED_FACE ( 'NONE', ( #27074 ), #6132, .T. ) ;
#11990=CARTESIAN_POINT ( 'NONE',  ( 166.1922820468853104, -1.999999999999972244, -2.083034168790677043 ) ) ;
#11991=ORIENTED_EDGE ( 'NONE', *, *, #29045, .F. ) ;
#11992=EDGE_CURVE ( 'NONE', #28209, #28125, #9610, .T. ) ;
#11993=FACE_OUTER_BOUND ( 'NONE', #19039, .T. ) ;
#11995=EDGE_CURVE ( 'NONE', #24401, #16811, #14032, .T. ) ;
#11998=VECTOR ( 'NONE', #14969, 1000.000000000000000 ) ;
#12000=VERTEX_POINT ( 'NONE', #16787 ) ;
#12001=APPLICATION_CONTEXT ( 'automotive_design' ) ;
#12002=AXIS2_PLACEMENT_3D ( 'NONE', #8733, #30016, #29570 ) ;
#12003=CARTESIAN_POINT ( 'NONE',  ( 167.0152310637604671, -9.999999999999996447, -17.38167787843871182 ) ) ;
#12004=DIRECTION ( 'NONE',  ( -0.9510565162951536422, -2.566386769018988816E-16, -0.3090169943749472292 ) ) ;
#12006=LINE ( 'NONE', #21319, #21948 ) ;
#12007=LINE ( 'NONE', #23473, #25203 ) ;
#12008=ORIENTED_EDGE ( 'NONE', *, *, #231, .F. ) ;
#12009=PLANE ( 'NONE',  #21720 ) ;
#12010=VERTEX_POINT ( 'NONE', #25648 ) ;
#12011=LINE ( 'NONE', #23946, #27369 ) ;
#12012=ORIENTED_EDGE ( 'NONE', *, *, #28646, .F. ) ;
#12018=VECTOR ( 'NONE', #5891, 1000.000000000000000 ) ;
#12019=CARTESIAN_POINT ( 'NONE',  ( 141.1922820468854241, -4.999999999999979572, -4.936203717676158398 ) ) ;
#12020=PLANE ( 'NONE',  #22350 ) ;
#12021=LINE ( 'NONE', #9731, #28448 ) ;
#12022=VECTOR ( 'NONE', #27389, 1000.000000000000000 ) ;
#12025=ORIENTED_EDGE ( 'NONE', *, *, #12331, .F. ) ;
#12026=LINE ( 'NONE', #29973, #15901 ) ;
#12030=ADVANCED_FACE ( 'NONE', ( #9148 ), #16483, .T. ) ;
#12031=EDGE_CURVE ( 'NONE', #3628, #9641, #20, .T. ) ;
#12032=FACE_OUTER_BOUND ( 'NONE', #17908, .T. ) ;
#12033=CARTESIAN_POINT ( 'NONE',  ( 107.3608926408196140, -4.999999999999988454, 78.00225434817323844 ) ) ;
#12034=ADVANCED_FACE ( 'NONE', ( #472 ), #326, .T. ) ;
#12035=EDGE_CURVE ( 'NONE', #5806, #12653, #18632, .T. ) ;
#12039=ORIENTED_EDGE ( 'NONE', *, *, #16797, .T. ) ;
#12041=VERTEX_POINT ( 'NONE', #9760 ) ;
#12043=VECTOR ( 'NONE', #3546, 1000.000000000000000 ) ;
#12046=CARTESIAN_POINT ( 'NONE',  ( 171.1922820468853104, -4.999999999999971578, -10.74328820663507678 ) ) ;
#12048=VECTOR ( 'NONE', #3895, 1000.000000000000000 ) ;
#12050=FACE_BOUND ( 'NONE', #5691, .T. ) ;
#12052=CARTESIAN_POINT ( 'NONE',  ( 163.6922820468853956, -1.999999999999971356, -32.39392330124607611 ) ) ;
#12055=ORIENTED_EDGE ( 'NONE', *, *, #18862, .F. ) ;
#12061=CARTESIAN_POINT ( 'NONE',  ( 152.2287565553230024, -10.00000000000000178, -20.83012701892220520 ) ) ;
#12062=ORIENTED_EDGE ( 'NONE', *, *, #8284, .F. ) ;
#12063=CARTESIAN_POINT ( 'NONE',  ( 108.2718491523516207, -4.999999999999987566, -78.66410299496463665 ) ) ;
#12067=VECTOR ( 'NONE', #22582, 1000.000000000000000 ) ;
#12069=FACE_BOUND ( 'NONE', #29356, .T. ) ;
#12071=EDGE_CURVE ( 'NONE', #20011, #18400, #4740, .T. ) ;
#12072=EDGE_CURVE ( 'NONE', #12263, #23543, #21211, .T. ) ;
#12073=ORIENTED_EDGE ( 'NONE', *, *, #10557, .T. ) ;
#12075=CARTESIAN_POINT ( 'NONE',  ( 169.7287565553229740, -9.999999999999996447, -33.82050807568879947 ) ) ;
#12077=FACE_OUTER_BOUND ( 'NONE', #19187, .T. ) ;
#12078=CARTESIAN_POINT ( 'NONE',  ( 153.6922820468853672, -1.999999999999975353, -6.413161187712876909 ) ) ;
#12080=LINE ( 'NONE', #20784, #11204 ) ;
#12085=VECTOR ( 'NONE', #11747, 1000.000000000000000 ) ;
#12087=CARTESIAN_POINT ( 'NONE',  ( 158.6922820468853956, -9.999999999999998224, -26.58683881228715862 ) ) ;
#12089=ORIENTED_EDGE ( 'NONE', *, *, #12547, .F. ) ;
#12091=ORIENTED_EDGE ( 'NONE', *, *, #9890, .F. ) ;
#12092=CARTESIAN_POINT ( 'NONE',  ( 174.5152310637604387, -9.999999999999994671, -11.28819510263909542 ) ) ;
#12094=VERTEX_POINT ( 'NONE', #7340 ) ;
#12095=VECTOR ( 'NONE', #12778, 1000.000000000000000 ) ;
#12098=CARTESIAN_POINT ( 'NONE',  ( 92.33196323856196841, -4.999999999999992006, -67.08309798704286209 ) ) ;
#12101=ORIENTED_EDGE ( 'NONE', *, *, #19067, .F. ) ;
#12102=VECTOR ( 'NONE', #10334, 1000.000000000000000 ) ;
#12104=ADVANCED_FACE ( 'NONE', ( #7040 ), #11895, .T. ) ;
#12108=CARTESIAN_POINT ( 'NONE',  ( 134.7287565553230024, -10.00000000000000711, -33.82050807568879947 ) ) ;
#12109=VERTEX_POINT ( 'NONE', #16331 ) ;
#12111=EDGE_CURVE ( 'NONE', #24640, #26897, #11595, .T. ) ;
#12112=DIRECTION ( 'NONE',  ( -2.698458740408365879E-16, 1.000000000000000000, 0.000000000000000000 ) ) ;
#12114=VECTOR ( 'NONE', #12471, 1000.000000000000000 ) ;
#12119=VECTOR ( 'NONE', #8046, 1000.000000000000000 ) ;
#12123=ORIENTED_EDGE ( 'NONE', *, *, #11117, .T. ) ;
#12124=VECTOR ( 'NONE', #2392, 1000.000000000000000 ) ;
#12125=CARTESIAN_POINT ( 'NONE',  ( 142.0152310637605808, -4.999999999999979572, -17.38167787843871182 ) ) ;
#12127=CARTESIAN_POINT ( 'NONE',  ( 173.6922820468853672, -1.999999999999970024, -32.39392330124607611 ) ) ;
#12128=LINE ( 'NONE', #21136, #16351 ) ;
#12130=VERTEX_POINT ( 'NONE', #173 ) ;
#12131=DIRECTION ( 'NONE',  ( -2.698458740408365879E-16, 1.000000000000000000, 0.000000000000000000 ) ) ;
#12133=DIRECTION ( 'NONE',  ( 0.5877852522924731371, 0.000000000000000000, 0.8090169943749474513 ) ) ;
#12134=CARTESIAN_POINT ( 'NONE',  ( 90.57535369523569102, -4.999999999999992895, 65.80684644871624300 ) ) ;
#12135=ORIENTED_EDGE ( 'NONE', *, *, #13650, .T. ) ;
#12138=VERTEX_POINT ( 'NONE', #16639 ) ;
#12141=AXIS2_PLACEMENT_3D ( 'NONE', #13613, #22943, #16049 ) ;
#12143=ORIENTED_EDGE ( 'NONE', *, *, #25072, .F. ) ;
#12144=EDGE_CURVE ( 'NONE', #4293, #11898, #14184, .T. ) ;
#12146=VECTOR ( 'NONE', #24779, 1000.000000000000000 ) ;
#12148=VERTEX_POINT ( 'NONE', #5190 ) ;
#12152=DIRECTION ( 'NONE',  ( -0.5877852522924731371, 0.000000000000000000, 0.8090169943749474513 ) ) ;
#12153=DIRECTION ( 'NONE',  ( -0.5877852522924731371, -1.586114251531760235E-16, 0.8090169943749474513 ) ) ;
#12157=CARTESIAN_POINT ( 'NONE',  ( 143.6922820468853956, -10.00000000000000533, 2.247092850131519715 ) ) ;
#12158=LINE ( 'NONE', #19478, #27094 ) ;
#12160=DIRECTION ( 'NONE',  ( 2.908569913943825554E-16, -1.000000000000000000, 0.000000000000000000 ) ) ;
#12161=VECTOR ( 'NONE', #15368, 1000.000000000000000 ) ;
#12163=ORIENTED_EDGE ( 'NONE', *, *, #21933, .F. ) ;
#12164=LINE ( 'NONE', #3333, #19768 ) ;
#12166=VERTEX_POINT ( 'NONE', #6896 ) ;
#12167=LINE ( 'NONE', #28972, #12048 ) ;
#12168=ORIENTED_EDGE ( 'NONE', *, *, #950, .T. ) ;
#12170=EDGE_CURVE ( 'NONE', #134, #5625, #2769, .T. ) ;
#12172=EDGE_CURVE ( 'NONE', #3548, #17432, #25505, .T. ) ;
#12175=DIRECTION ( 'NONE',  ( 0.5877852522924731371, 1.586114251531760728E-16, 0.8090169943749474513 ) ) ;
#12176=ADVANCED_FACE ( 'NONE', ( #29185 ), #3217, .T. ) ;
#12178=VECTOR ( 'NONE', #21014, 999.9999999999998863 ) ;
#12179=CARTESIAN_POINT ( 'NONE',  ( 164.7287565553228887, -9.999999999999998224, 0.8205080756887930260 ) ) ;
#12180=DIRECTION ( 'NONE',  ( 0.3090169943749472292, 8.338696094057992503E-17, -0.9510565162951536422 ) ) ;
#12181=DIRECTION ( 'NONE',  ( 1.000000000000000000, 2.698458740408365879E-16, -1.110223024625156540E-16 ) ) ;
#12182=PLANE ( 'NONE',  #25372 ) ;
#12183=LINE ( 'NONE', #17516, #13344 ) ;
#12184=AXIS2_PLACEMENT_3D ( 'NONE', #8253, #6127, #27230 ) ;
#12187=DIRECTION ( 'NONE',  ( -1.000000000000000000, -2.698458740408366372E-16, 8.163404592832029035E-16 ) ) ;
#12190=VECTOR ( 'NONE', #25239, 1000.000000000000000 ) ;
#12195=FACE_BOUND ( 'NONE', #50, .T. ) ;
#12198=VERTEX_POINT ( 'NONE', #7779 ) ;
#12200=DIRECTION ( 'NONE',  ( -0.5877852522924731371, -1.586114251531760235E-16, 0.8090169943749474513 ) ) ;
#12202=DIRECTION ( 'NONE',  ( -0.9510565162951536422, 0.000000000000000000, -0.3090169943749472292 ) ) ;
#12203=ORIENTED_EDGE ( 'NONE', *, *, #8452, .F. ) ;
#12204=DIRECTION ( 'NONE',  ( -0.5877852522924731371, -1.586114251531760235E-16, 0.8090169943749474513 ) ) ;
#12205=EDGE_LOOP ( 'NONE', ( #22510, #12537, #7828, #28589, #7782 ) ) ;
#12207=ORIENTED_EDGE ( 'NONE', *, *, #24184, .F. ) ;
#12211=VERTEX_POINT ( 'NONE', #8070 ) ;
#12212=EDGE_CURVE ( 'NONE', #1890, #26875, #8222, .T. ) ;
#12213=CARTESIAN_POINT ( 'NONE',  ( 16.16257886861838955, -5.000000000000013323, -49.74330290224348516 ) ) ;
#12215=EDGE_CURVE ( 'NONE', #23323, #29393, #19820, .T. ) ;
#12216=EDGE_CURVE ( 'NONE', #2560, #4171, #17380, .T. ) ;
#12221=AXIS2_PLACEMENT_3D ( 'NONE', #22306, #19854, #3545 ) ;
#12223=CARTESIAN_POINT ( 'NONE',  ( 146.1922820468854525, -4.999999999999978684, -30.91696583120935671 ) ) ;
#12224=FACE_BOUND ( 'NONE', #2482, .T. ) ;
#12227=CARTESIAN_POINT ( 'NONE',  ( 166.1922820468853388, -1.999999999999971800, -10.74328820663507678 ) ) ;
#12228=CARTESIAN_POINT ( 'NONE',  ( 129.5152310637605808, -10.00000000000000888, -2.627941064794695691 ) ) ;
#12231=DIRECTION ( 'NONE',  ( 1.110223024625156540E-16, 2.995891024602366092E-32, 1.000000000000000000 ) ) ;
#12232=AXIS2_PLACEMENT_3D ( 'NONE', #11965, #4656, #2239 ) ;
#12233=CARTESIAN_POINT ( 'NONE',  ( 152.0152310637606092, -1.999999999999974465, -32.93883019725009120 ) ) ;
#12234=VERTEX_POINT ( 'NONE', #15079 ) ;
#12235=VECTOR ( 'NONE', #3740, 1000.000000000000000 ) ;
#12237=ORIENTED_EDGE ( 'NONE', *, *, #28491, .T. ) ;
#12240=CARTESIAN_POINT ( 'NONE',  ( 164.5152310637604671, -9.999999999999998224, -2.627941064794695691 ) ) ;
#12241=DIRECTION ( 'NONE',  ( -0.8090169943749474513, -2.183098979609982436E-16, 0.5877852522924731371 ) ) ;
#12242=ORIENTED_EDGE ( 'NONE', *, *, #10477, .F. ) ;
#12243=FACE_OUTER_BOUND ( 'NONE', #12352, .T. ) ;
#12248=ADVANCED_FACE ( 'NONE', ( #12495 ), #760, .T. ) ;
#12249=DIRECTION ( 'NONE',  ( -0.8090169943749474513, -2.183098979609982436E-16, -0.5877852522924731371 ) ) ;
#12252=EDGE_CURVE ( 'NONE', #10971, #3997, #24120, .T. ) ;
#12253=LINE ( 'NONE', #28483, #18844 ) ;
#12257=ORIENTED_EDGE ( 'NONE', *, *, #4534, .T. ) ;
#12258=CARTESIAN_POINT ( 'NONE',  ( 130.7287565553229172, -4.999999999999983125, -28.21440484423857242 ) ) ;
#12259=ORIENTED_EDGE ( 'NONE', *, *, #10581, .F. ) ;
#12260=DIRECTION ( 'NONE',  ( 0.5877852522924731371, 0.000000000000000000, 0.8090169943749474513 ) ) ;
#12261=VECTOR ( 'NONE', #1296, 1000.000000000000000 ) ;
#12262=PLANE ( 'NONE',  #6992 ) ;
#12263=VERTEX_POINT ( 'NONE', #24268 ) ;
#12264=CARTESIAN_POINT ( 'NONE',  ( 144.5152310637605240, -4.999999999999978684, -1.604441369360115876E-14 ) ) ;
#12265=DIRECTION ( 'NONE',  ( -1.000000000000000000, 0.000000000000000000, 0.000000000000000000 ) ) ;
#12266=FACE_OUTER_BOUND ( 'NONE', #17765, .T. ) ;
#12270=EDGE_CURVE ( 'NONE', #24297, #25495, #918, .T. ) ;
#12277=PLANE ( 'NONE',  #17552 ) ;
#12280=ORIENTED_EDGE ( 'NONE', *, *, #30125, .T. ) ;
#12281=DIRECTION ( 'NONE',  ( -2.698458740408365879E-16, 1.000000000000000000, 0.000000000000000000 ) ) ;
#12283=CARTESIAN_POINT ( 'NONE',  ( 142.0152310637605808, -10.00000000000000355, -34.70218595412750773 ) ) ;
#12287=EDGE_LOOP ( 'NONE', ( #24966, #25393, #2583, #24815, #23035, #16542 ) ) ;
#12290=VECTOR ( 'NONE', #18335, 1000.000000000000000 ) ;
#12292=VERTEX_POINT ( 'NONE', #12347 ) ;
#12295=AXIS2_PLACEMENT_3D ( 'NONE', #8048, #24095, #3197 ) ;
#12296=ORIENTED_EDGE ( 'NONE', *, *, #24912, .T. ) ;
#12297=CARTESIAN_POINT ( 'NONE',  ( 172.7287565553229456, -1.999999999999970468, -33.50000000000000000 ) ) ;
#12298=LINE ( 'NONE', #1781, #11892 ) ;
#12299=DIRECTION ( 'NONE',  ( 0.3090169943749475623, 8.338696094058001131E-17, 0.9510565162951536422 ) ) ;
#12304=VECTOR ( 'NONE', #4907, 1000.000000000000000 ) ;
#12305=DIRECTION ( 'NONE',  ( 0.5877852522924731371, 0.000000000000000000, 0.8090169943749474513 ) ) ;
#12306=CARTESIAN_POINT ( 'NONE',  ( 152.0152310637605808, -1.999999999999974465, -34.70218595412750773 ) ) ;
#12308=CARTESIAN_POINT ( 'NONE',  ( 157.0152310637604955, -1.999999999999974021, -17.38167787843871182 ) ) ;
#12309=LINE ( 'NONE', #19330, #28593 ) ;
#12310=ORIENTED_EDGE ( 'NONE', *, *, #4611, .T. ) ;
#12311=ORIENTED_EDGE ( 'NONE', *, *, #26083, .T. ) ;
#12312=DIRECTION ( 'NONE',  ( -0.8090169943749474513, -2.183098979609982436E-16, -0.5877852522924731371 ) ) ;
#12313=ORIENTED_EDGE ( 'NONE', *, *, #4123, .T. ) ;
#12314=ORIENTED_EDGE ( 'NONE', *, *, #12592, .F. ) ;
#12318=CARTESIAN_POINT ( 'NONE',  ( 171.1922820468852819, -1.999999999999971356, -4.936203717676158398 ) ) ;
#12320=DIRECTION ( 'NONE',  ( -0.9510565162951536422, -2.566386769018988816E-16, -0.3090169943749472292 ) ) ;
#12321=VERTEX_POINT ( 'NONE', #3513 ) ;
#12322=ORIENTED_EDGE ( 'NONE', *, *, #3151, .T. ) ;
#12323=LINE ( 'NONE', #21638, #3576 ) ;
#12324=CARTESIAN_POINT ( 'NONE',  ( 157.2287565553229740, -10.00000000000000000, -20.83012701892220520 ) ) ;
#12325=PLANE ( 'NONE',  #19965 ) ;
#12326=DIRECTION ( 'NONE',  ( -0.8090169943749474513, -2.183098979609982436E-16, -0.5877852522924731371 ) ) ;
#12328=AXIS2_PLACEMENT_3D ( 'NONE', #7985, #26630, #3718 ) ;
#12330=EDGE_CURVE ( 'NONE', #9369, #19861, #26566, .T. ) ;
#12331=EDGE_CURVE ( 'NONE', #21151, #14407, #15237, .T. ) ;
#12332=PLANE ( 'NONE',  #23844 ) ;
#12336=EDGE_CURVE ( 'NONE', #1843, #15349, #12652, .T. ) ;
#12337=CARTESIAN_POINT ( 'NONE',  ( 136.1922820468854241, -10.00000000000000533, -22.25671179336495697 ) ) ;
#12338=EDGE_CURVE ( 'NONE', #5003, #280, #3660, .T. ) ;
#12341=DIRECTION ( 'NONE',  ( -1.110223024625156540E-16, 0.000000000000000000, -1.000000000000000000 ) ) ;
#12342=ORIENTED_EDGE ( 'NONE', *, *, #20669, .F. ) ;
#12343=ORIENTED_EDGE ( 'NONE', *, *, #16658, .T. ) ;
#12345=CARTESIAN_POINT ( 'NONE',  ( 151.1922820468853956, -1.999999999999976241, -13.59645775552055902 ) ) ;
#12347=CARTESIAN_POINT ( 'NONE',  ( 130.7287565553229456, -10.00000000000000888, -2.233642730705364343 ) ) ;
#12348=ORIENTED_EDGE ( 'NONE', *, *, #16347, .F. ) ;
#12349=CARTESIAN_POINT ( 'NONE',  ( 149.5152310637605240, -10.00000000000000178, -2.627941064794695691 ) ) ;
#12350=ORIENTED_EDGE ( 'NONE', *, *, #13852, .F. ) ;
#12352=EDGE_LOOP ( 'NONE', ( #8825, #29900, #27229, #19278 ) ) ;
#12356=ORIENTED_EDGE ( 'NONE', *, *, #15375, .T. ) ;
#12357=ORIENTED_EDGE ( 'NONE', *, *, #10828, .T. ) ;
#12359=VECTOR ( 'NONE', #26871, 1000.000000000000000 ) ;
#12360=ORIENTED_EDGE ( 'NONE', *, *, #2557, .F. ) ;
#12365=LINE ( 'NONE', #3238, #14420 ) ;
#12366=FACE_BOUND ( 'NONE', #27036, .T. ) ;
#12367=VERTEX_POINT ( 'NONE', #623 ) ;
#12368=DIRECTION ( 'NONE',  ( 0.9510565162951536422, 2.566386769018988816E-16, 0.3090169943749472292 ) ) ;
#12370=DIRECTION ( 'NONE',  ( -0.5877852522924731371, 0.000000000000000000, 0.8090169943749474513 ) ) ;
#12371=EDGE_CURVE ( 'NONE', #21981, #3855, #19218, .T. ) ;
#12372=CARTESIAN_POINT ( 'NONE',  ( 174.5152310637604387, -1.999999999999969580, -11.28819510263909542 ) ) ;
#12373=VECTOR ( 'NONE', #11218, 1000.000000000000000 ) ;
#12374=EDGE_CURVE ( 'NONE', #9954, #24408, #23981, .T. ) ;
#12375=ADVANCED_FACE ( 'NONE', ( #19523 ), #28894, .T. ) ;
#12379=ORIENTED_EDGE ( 'NONE', *, *, #7439, .T. ) ;
#12380=CARTESIAN_POINT ( 'NONE',  ( 144.5152310637605808, -10.00000000000000355, -11.28819510263909542 ) ) ;
#12381=VERTEX_POINT ( 'NONE', #29815 ) ;
#12383=VERTEX_POINT ( 'NONE', #3813 ) ;
#12386=CARTESIAN_POINT ( 'NONE',  ( 154.5152310637605524, -10.00000000000000000, -30.37205893520531319 ) ) ;
#12387=CARTESIAN_POINT ( 'NONE',  ( 151.1922820468854525, -4.999999999999976907, -30.91696583120936026 ) ) ;
#12389=FACE_OUTER_BOUND ( 'NONE', #17554, .T. ) ;
#12391=ORIENTED_EDGE ( 'NONE', *, *, #12414, .F. ) ;
#12395=FACE_OUTER_BOUND ( 'NONE', #5769, .T. ) ;
#12397=ORIENTED_EDGE ( 'NONE', *, *, #26650, .T. ) ;
#12401=VECTOR ( 'NONE', #7547, 1000.000000000000000 ) ;
#12403=EDGE_LOOP ( 'NONE', ( #5916, #15109, #7349, #21329 ) ) ;
#12404=ORIENTED_EDGE ( 'NONE', *, *, #1892, .F. ) ;
#12406=CARTESIAN_POINT ( 'NONE',  ( 163.6922820468853388, -4.999999999999973355, -17.92658477444275889 ) ) ;
#12407=LINE ( 'NONE', #5560, #29605 ) ;
#12408=DIRECTION ( 'NONE',  ( -2.698458740408365879E-16, 1.000000000000000000, 0.000000000000000000 ) ) ;
#12409=EDGE_CURVE ( 'NONE', #10981, #28540, #13106, .T. ) ;
#12412=ADVANCED_FACE ( 'NONE', ( #1990 ), #24726, .T. ) ;
#12414=EDGE_CURVE ( 'NONE', #18724, #11499, #6550, .T. ) ;
#12418=VERTEX_POINT ( 'NONE', #25027 ) ;
#12419=CARTESIAN_POINT ( 'NONE',  ( 169.7287565553229740, -1.999999999999969580, -33.82050807568879947 ) ) ;
#12421=CARTESIAN_POINT ( 'NONE',  ( 149.5152310637605808, -10.00000000000000178, -19.94844914048349693 ) ) ;
#12422=CARTESIAN_POINT ( 'NONE',  ( 166.1922820468853104, -4.999999999999973355, -4.936203717676158398 ) ) ;
#12423=CARTESIAN_POINT ( 'NONE',  ( 157.0152310637604955, -10.00000000000000000, -17.38167787843871182 ) ) ;
#12424=LINE ( 'NONE', #2684, #20252 ) ;
#12426=ORIENTED_EDGE ( 'NONE', *, *, #5742, .F. ) ;
#12427=PLANE ( 'NONE',  #13912 ) ;
#12430=CARTESIAN_POINT ( 'NONE',  ( 139.5152310637606092, -4.999999999999980460, -19.94844914048349338 ) ) ;
#12433=ORIENTED_EDGE ( 'NONE', *, *, #19276, .F. ) ;
#12437=VECTOR ( 'NONE', #10840, 1000.000000000000000 ) ;
#12439=LINE ( 'NONE', #3756, #15253 ) ;
#12441=FACE_OUTER_BOUND ( 'NONE', #29387, .T. ) ;
#12442=CARTESIAN_POINT ( 'NONE',  ( 134.7287565553230024, -10.00000000000000711, -25.16025403784439973 ) ) ;
#12443=CARTESIAN_POINT ( 'NONE',  ( 173.6922820468852535, -1.999999999999970912, -0.6060766987539614181 ) ) ;
#12444=EDGE_CURVE ( 'NONE', #17847, #21366, #29660, .T. ) ;
#12445=EDGE_CURVE ( 'NONE', #5191, #3131, #20127, .T. ) ;
#12447=AXIS2_PLACEMENT_3D ( 'NONE', #27749, #27903, #30210 ) ;
#12451=CARTESIAN_POINT ( 'NONE',  ( 164.7287565553229740, -9.999999999999998224, -33.82050807568879947 ) ) ;
#12452=CARTESIAN_POINT ( 'NONE',  ( 172.0152310637605240, -4.999999999999971578, -32.93883019725009120 ) ) ;
#12454=CARTESIAN_POINT ( 'NONE',  ( 174.7287565553228603, -1.999999999999969580, -7.839745962155603820 ) ) ;
#12455=CARTESIAN_POINT ( 'NONE',  ( 162.2287565553229172, -1.999999999999972689, -12.16987298107780369 ) ) ;
#12456=ORIENTED_EDGE ( 'NONE', *, *, #25339, .F. ) ;
#12457=EDGE_LOOP ( 'NONE', ( #22622, #21655, #3735, #16470 ) ) ;
#12458=VECTOR ( 'NONE', #2845, 1000.000000000000000 ) ;
#12459=PLANE ( 'NONE',  #18295 ) ;
#12460=CARTESIAN_POINT ( 'NONE',  ( 152.0152310637604955, -1.999999999999976241, 1.702185954127501066 ) ) ;
#12462=CARTESIAN_POINT ( 'NONE',  ( 172.2287565553228603, -9.999999999999996447, -3.509618943233403510 ) ) ;
#12463=ORIENTED_EDGE ( 'NONE', *, *, #18173, .T. ) ;
#12464=VERTEX_POINT ( 'NONE', #17829 ) ;
#12466=VERTEX_POINT ( 'NONE', #3967 ) ;
#12468=VECTOR ( 'NONE', #28037, 1000.000000000000000 ) ;
#12471=DIRECTION ( 'NONE',  ( 0.9510565162951535312, 2.566386769018988816E-16, -0.3090169943749475623 ) ) ;
#12473=PLANE ( 'NONE',  #614 ) ;
#12474=ADVANCED_FACE ( 'NONE', ( #13559 ), #18136, .T. ) ;
#12475=VECTOR ( 'NONE', #6817, 1000.000000000000000 ) ;
#12476=PLANE ( 'NONE',  #11838 ) ;
#12477=FACE_OUTER_BOUND ( 'NONE', #24459, .T. ) ;
#12478=PLANE ( 'NONE',  #21430 ) ;
#12482=CARTESIAN_POINT ( 'NONE',  ( 139.5152310637605524, -10.00000000000000533, -4.391296821672111328 ) ) ;
#12490=FACE_BOUND ( 'NONE', #1521, .T. ) ;
#12492=PLANE ( 'NONE',  #2377 ) ;
#12495=FACE_OUTER_BOUND ( 'NONE', #15933, .T. ) ;
#12496=VERTEX_POINT ( 'NONE', #10671 ) ;
#12497=PLANE ( 'NONE',  #9579 ) ;
#12498=ORIENTED_EDGE ( 'NONE', *, *, #28580, .T. ) ;
#12500=ORIENTED_EDGE ( 'NONE', *, *, #1587, .F. ) ;
#12501=VECTOR ( 'NONE', #17685, 1000.000000000000000 ) ;
#12505=VECTOR ( 'NONE', #16669, 1000.000000000000000 ) ;
#12506=CARTESIAN_POINT ( 'NONE',  ( 177.2287565553228603, -9.999999999999994671, -12.16987298107780369 ) ) ;
#12508=CARTESIAN_POINT ( 'NONE',  ( 156.1922820468853956, -10.00000000000000000, -19.40354224447947828 ) ) ;
#12510=EDGE_CURVE ( 'NONE', #590, #13010, #13265, .T. ) ;
#12511=EDGE_CURVE ( 'NONE', #13196, #12109, #10964, .T. ) ;
#12517=FACE_BOUND ( 'NONE', #25462, .T. ) ;
#12518=VECTOR ( 'NONE', #7072, 1000.000000000000000 ) ;
#12519=CARTESIAN_POINT ( 'NONE',  ( 134.7287565553230024, -1.999999999999980460, -16.50000000000000000 ) ) ;
#12520=LINE ( 'NONE', #21393, #19904 ) ;
#12522=VECTOR ( 'NONE', #18522, 1000.000000000000000 ) ;
#12523=CARTESIAN_POINT ( 'NONE',  ( 139.7287565553230309, -10.00000000000000533, -16.50000000000000000 ) ) ;
#12525=DIRECTION ( 'NONE',  ( -0.9510565162951536422, 0.000000000000000000, -0.3090169943749472292 ) ) ;
#12526=VECTOR ( 'NONE', #27096, 1000.000000000000000 ) ;
#12527=CARTESIAN_POINT ( 'NONE',  ( 137.0152310637606092, -10.00000000000000533, -6.958068083716895558 ) ) ;
#12528=ORIENTED_EDGE ( 'NONE', *, *, #22032, .T. ) ;
#12530=EDGE_LOOP ( 'NONE', ( #26914, #26459, #16262, #7295 ) ) ;
#12532=CARTESIAN_POINT ( 'NONE',  ( 163.6922820468853104, -1.999999999999973133, -6.413161187712876909 ) ) ;
#12533=PLANE ( 'NONE',  #23257 ) ;
#12534=LINE ( 'NONE', #10397, #3917 ) ;
#12535=ORIENTED_EDGE ( 'NONE', *, *, #21229, .F. ) ;
#12536=CARTESIAN_POINT ( 'NONE',  ( 130.7287565553229172, -4.999999999999983125, -33.50000000000000000 ) ) ;
#12537=ORIENTED_EDGE ( 'NONE', *, *, #20651, .T. ) ;
#12539=ORIENTED_EDGE ( 'NONE', *, *, #22246, .F. ) ;
#12543=VECTOR ( 'NONE', #26368, 999.9999999999998863 ) ;
#12544=LINE ( 'NONE', #21863, #19872 ) ;
#12547=EDGE_CURVE ( 'NONE', #17432, #12041, #27498, .T. ) ;
#12549=VECTOR ( 'NONE', #2334, 1000.000000000000000 ) ;
#12550=EDGE_CURVE ( 'NONE', #2172, #29884, #12900, .T. ) ;
#12553=ORIENTED_EDGE ( 'NONE', *, *, #3952, .T. ) ;
#12554=EDGE_CURVE ( 'NONE', #3882, #14836, #28679, .T. ) ;
#12555=VERTEX_POINT ( 'NONE', #1323 ) ;
#12556=DIRECTION ( 'NONE',  ( -2.698458740408365879E-16, 1.000000000000000000, 0.000000000000000000 ) ) ;
#12558=DIRECTION ( 'NONE',  ( 1.110223024625156540E-16, 2.995891024602366092E-32, 1.000000000000000000 ) ) ;
#12559=LINE ( 'NONE', #21877, #27780 ) ;
#12560=DIRECTION ( 'NONE',  ( -0.9510565162951536422, -2.566386769018988323E-16, 0.3090169943749475623 ) ) ;
#12561=VECTOR ( 'NONE', #20905, 1000.000000000000000 ) ;
#12566=VERTEX_POINT ( 'NONE', #26831 ) ;
#12567=CARTESIAN_POINT ( 'NONE',  ( 103.6655236389851069, -4.999999999999989342, 75.31741161166775100 ) ) ;
#12568=VECTOR ( 'NONE', #21038, 1000.000000000000000 ) ;
#12569=LINE ( 'NONE', #5419, #2879 ) ;
#12570=CARTESIAN_POINT ( 'NONE',  ( 157.2287565553229172, -10.00000000000000178, -3.509618943233403510 ) ) ;
#12572=LINE ( 'NONE', #21891, #26362 ) ;
#12573=CARTESIAN_POINT ( 'NONE',  ( 134.7287565553230024, -1.999999999999980460, -7.839745962155602044 ) ) ;
#12575=ORIENTED_EDGE ( 'NONE', *, *, #27973, .T. ) ;
#12576=LINE ( 'NONE', #29112, #7610 ) ;
#12580=CARTESIAN_POINT ( 'NONE',  ( 141.1922820468853956, -1.999999999999979128, -2.083034168790675267 ) ) ;
#12581=ORIENTED_EDGE ( 'NONE', *, *, #1373, .T. ) ;
#12582=ORIENTED_EDGE ( 'NONE', *, *, #16268, .F. ) ;
#12585=ORIENTED_EDGE ( 'NONE', *, *, #2713, .F. ) ;
#12591=VECTOR ( 'NONE', #13403, 1000.000000000000000 ) ;
#12592=EDGE_CURVE ( 'NONE', #1878, #6853, #19318, .T. ) ;
#12593=ADVANCED_FACE ( 'NONE', ( #24070 ), #10615, .T. ) ;
#12594=EDGE_CURVE ( 'NONE', #18794, #4418, #17329, .T. ) ;
#12596=VECTOR ( 'NONE', #10797, 1000.000000000000000 ) ;
#12597=CARTESIAN_POINT ( 'NONE',  ( 4.873852431642221816, -5.000000000000015987, 15.00017539148683454 ) ) ;
#12598=VECTOR ( 'NONE', #12175, 1000.000000000000000 ) ;
#12601=PLANE ( 'NONE',  #4773 ) ;
#12602=CARTESIAN_POINT ( 'NONE',  ( 154.5152310637605808, -10.00000000000000000, -28.60870317832789667 ) ) ;
#12606=DIRECTION ( 'NONE',  ( 0.5877852522924731371, 0.000000000000000000, 0.8090169943749474513 ) ) ;
#12607=PLANE ( 'NONE',  #26119 ) ;
#12609=FACE_OUTER_BOUND ( 'NONE', #11538, .T. ) ;
#12610=ORIENTED_EDGE ( 'NONE', *, *, #20161, .T. ) ;
#12612=VERTEX_POINT ( 'NONE', #7728 ) ;
#12613=ORIENTED_EDGE ( 'NONE', *, *, #28003, .T. ) ;
#12615=CARTESIAN_POINT ( 'NONE',  ( 173.6922820468853388, -4.999999999999969802, -23.73366926340167637 ) ) ;
#12616=DIRECTION ( 'NONE',  ( -2.698458740408365879E-16, 1.000000000000000000, 0.000000000000000000 ) ) ;
#12617=PLANE ( 'NONE',  #27858 ) ;
#12619=ORIENTED_EDGE ( 'NONE', *, *, #6123, .T. ) ;
#12623=EDGE_CURVE ( 'NONE', #8261, #26148, #14876, .T. ) ;
#12625=LINE ( 'NONE', #17656, #21876 ) ;
#12626=PLANE ( 'NONE',  #25296 ) ;
#12627=EDGE_CURVE ( 'NONE', #14866, #13813, #3173, .T. ) ;
#12628=CARTESIAN_POINT ( 'NONE',  ( 149.7287565553230024, -1.999999999999975797, -16.50000000000000355 ) ) ;
#12631=DIRECTION ( 'NONE',  ( 0.3090169943749472292, 8.338696094057992503E-17, -0.9510565162951536422 ) ) ;
#12632=CARTESIAN_POINT ( 'NONE',  ( 152.0152310637605240, -1.999999999999975797, -6.958068083716895558 ) ) ;
#12633=VECTOR ( 'NONE', #1557, 999.9999999999998863 ) ;
#12635=DIRECTION ( 'NONE',  ( 0.9510565162951536422, 0.000000000000000000, -0.3090169943749475623 ) ) ;
#12638=CARTESIAN_POINT ( 'NONE',  ( 12.43045822248789456, -5.000000000000014211, 38.25701663089573401 ) ) ;
#12642=VERTEX_POINT ( 'NONE', #1177 ) ;
#12646=FACE_BOUND ( 'NONE', #18851, .T. ) ;
#12647=ORIENTED_EDGE ( 'NONE', *, *, #5086, .F. ) ;
#12648=EDGE_CURVE ( 'NONE', #5025, #23986, #29287, .T. ) ;
#12649=ORIENTED_EDGE ( 'NONE', *, *, #24528, .T. ) ;
#12650=CARTESIAN_POINT ( 'NONE',  ( 157.0152310637604955, -1.999999999999974021, -17.38167787843871182 ) ) ;
#12652=LINE ( 'NONE', #29032, #18414 ) ;
#12653=VERTEX_POINT ( 'NONE', #21769 ) ;
#12654=LINE ( 'NONE', #5349, #350 ) ;
#12656=VECTOR ( 'NONE', #3320, 1000.000000000000000 ) ;
#12658=ORIENTED_EDGE ( 'NONE', *, *, #23456, .T. ) ;
#12662=CARTESIAN_POINT ( 'NONE',  ( 159.5152310637604955, -1.999999999999973577, -11.28819510263909542 ) ) ;
#12663=ORIENTED_EDGE ( 'NONE', *, *, #20036, .T. ) ;
#12664=VECTOR ( 'NONE', #25453, 1000.000000000000000 ) ;
#12671=DIRECTION ( 'NONE',  ( 0.9510565162951536422, 0.000000000000000000, -0.3090169943749475623 ) ) ;
#12672=DIRECTION ( 'NONE',  ( 0.3090169943749472292, 8.338696094057992503E-17, -0.9510565162951536422 ) ) ;
#12673=VECTOR ( 'NONE', #6021, 1000.000000000000000 ) ;
#12675=FACE_OUTER_BOUND ( 'NONE', #23631, .T. ) ;
#12676=PLANE ( 'NONE',  #13059 ) ;
#12677=VECTOR ( 'NONE', #8180, 1000.000000000000000 ) ;
#12679=LINE ( 'NONE', #21999, #8540 ) ;
#12683=CARTESIAN_POINT ( 'NONE',  ( 136.1922820468854241, -1.999999999999980460, -2.083034168790677043 ) ) ;
#12686=ADVANCED_FACE ( 'NONE', ( #26986 ), #1030, .F. ) ;
#12689=CARTESIAN_POINT ( 'NONE',  ( 132.0152310637605524, -10.00000000000000711, -8.721423840594310306 ) ) ;
#12690=CARTESIAN_POINT ( 'NONE',  ( 152.2287565553229740, -10.00000000000000178, -12.16987298107780369 ) ) ;
#12691=VERTEX_POINT ( 'NONE', #28840 ) ;
#12692=CARTESIAN_POINT ( 'NONE',  ( 172.0152310637604387, -4.999999999999970690, -6.958068083716895558 ) ) ;
#12693=ORIENTED_EDGE ( 'NONE', *, *, #18075, .T. ) ;
#12696=VECTOR ( 'NONE', #15578, 1000.000000000000000 ) ;
#12698=EDGE_LOOP ( 'NONE', ( #22927, #15226, #2811, #22697, #7967 ) ) ;
#12699=CARTESIAN_POINT ( 'NONE',  ( 149.5152310637604955, -1.999999999999976685, -4.391296821672111328 ) ) ;
#12701=LINE ( 'NONE', #19714, #15543 ) ;
#12702=PLANE ( 'NONE',  #11509 ) ;
#12703=VECTOR ( 'NONE', #10650, 1000.000000000000000 ) ;
#12708=FACE_OUTER_BOUND ( 'NONE', #3115, .T. ) ;
#12709=CARTESIAN_POINT ( 'NONE',  ( 174.5152310637604103, -4.999999999999970690, -2.627941064794695691 ) ) ;
#12710=VECTOR ( 'NONE', #9254, 1000.000000000000000 ) ;
#12711=LINE ( 'NONE', #8135, #1779 ) ;
#12712=DIRECTION ( 'NONE',  ( 1.000000000000000000, 2.698458740408365879E-16, -1.110223024625156540E-16 ) ) ;
#12713=VECTOR ( 'NONE', #3754, 1000.000000000000000 ) ;
#12714=DIRECTION ( 'NONE',  ( -0.9510565162951536422, -2.566386769018988816E-16, -0.3090169943749472292 ) ) ;
#12715=EDGE_LOOP ( 'NONE', ( #11284, #8734, #11249, #6547 ) ) ;
#12720=ORIENTED_EDGE ( 'NONE', *, *, #26320, .F. ) ;
#12722=PLANE ( 'NONE',  #7250 ) ;
#12723=LINE ( 'NONE', #10585, #15050 ) ;
#12724=CARTESIAN_POINT ( 'NONE',  ( 130.7287565553229456, -4.999999999999982236, -22.10610323145026257 ) ) ;
#12728=ADVANCED_FACE ( 'NONE', ( #3322 ), #12601, .T. ) ;
#12730=ORIENTED_EDGE ( 'NONE', *, *, #19233, .T. ) ;
#12735=ORIENTED_EDGE ( 'NONE', *, *, #19274, .T. ) ;
#12739=ORIENTED_EDGE ( 'NONE', *, *, #23377, .T. ) ;
#12740=CARTESIAN_POINT ( 'NONE',  ( 133.7287565553229456, -1.999999999999980904, 0.5000000000000029976 ) ) ;
#12741=VECTOR ( 'NONE', #2548, 1000.000000000000000 ) ;
#12744=VECTOR ( 'NONE', #21740, 1000.000000000000000 ) ;
#12749=DIRECTION ( 'NONE',  ( -2.698458740408365879E-16, 1.000000000000000000, 0.000000000000000000 ) ) ;
#12750=LINE ( 'NONE', #24365, #11206 ) ;
#12752=CARTESIAN_POINT ( 'NONE',  ( 134.5152310637605524, -1.999999999999980460, -30.37205893520530964 ) ) ;
#12753=LINE ( 'NONE', #27139, #6341 ) ;
#12756=EDGE_CURVE ( 'NONE', #16032, #29409, #16089, .T. ) ;
#12757=LINE ( 'NONE', #9866, #22488 ) ;
#12758=DIRECTION ( 'NONE',  ( -0.5877852522924731371, 0.000000000000000000, 0.8090169943749474513 ) ) ;
#12759=EDGE_CURVE ( 'NONE', #26933, #24650, #4206, .T. ) ;
#12760=EDGE_CURVE ( 'NONE', #11338, #20741, #3909, .T. ) ;
#12763=EDGE_CURVE ( 'NONE', #22297, #15701, #23120, .T. ) ;
#12764=ORIENTED_EDGE ( 'NONE', *, *, #9412, .F. ) ;
#12766=ORIENTED_EDGE ( 'NONE', *, *, #17070, .T. ) ;
#12768=CARTESIAN_POINT ( 'NONE',  ( 123.8989781914840336, -4.999999999999984013, -90.01787683252187833 ) ) ;
#12769=VECTOR ( 'NONE', #25371, 1000.000000000000000 ) ;
#12771=VERTEX_POINT ( 'NONE', #25414 ) ;
#12774=VERTEX_POINT ( 'NONE', #13794 ) ;
#12778=DIRECTION ( 'NONE',  ( 0.5877852522924731371, 1.586114251531760728E-16, 0.8090169943749474513 ) ) ;
#12779=CARTESIAN_POINT ( 'NONE',  ( 158.6922820468853104, -4.999999999999975131, -0.6060766987539614181 ) ) ;
#12780=VECTOR ( 'NONE', #6261, 1000.000000000000000 ) ;
#12781=DIRECTION ( 'NONE',  ( 0.5877852522924731371, 0.000000000000000000, 0.8090169943749474513 ) ) ;
#12782=ORIENTED_EDGE ( 'NONE', *, *, #9964, .F. ) ;
#12783=VERTEX_POINT ( 'NONE', #20520 ) ;
#12785=VERTEX_POINT ( 'NONE', #4058 ) ;
#12787=EDGE_CURVE ( 'NONE', #2431, #2626, #13502, .T. ) ;
#12789=AXIS2_PLACEMENT_3D ( 'NONE', #19200, #12180, #20886 ) ;
#12791=FACE_OUTER_BOUND ( 'NONE', #11183, .T. ) ;
#12794=EDGE_LOOP ( 'NONE', ( #2014, #12135, #23747, #7324, #30145 ) ) ;
#12796=EDGE_CURVE ( 'NONE', #20051, #26875, #15491, .T. ) ;
#12797=VECTOR ( 'NONE', #23722, 1000.000000000000000 ) ;
#12801=FACE_BOUND ( 'NONE', #4744, .T. ) ;
#12802=EDGE_CURVE ( 'NONE', #2569, #5343, #6646, .T. ) ;
#12805=CARTESIAN_POINT ( 'NONE',  ( 7.896494747980494111, -5.000000000000015987, 24.30291188725040641 ) ) ;
#12807=DIRECTION ( 'NONE',  ( -2.698458740408365879E-16, 1.000000000000000000, 0.000000000000000000 ) ) ;
#12808=ORIENTED_EDGE ( 'NONE', *, *, #25485, .F. ) ;
#12810=ORIENTED_EDGE ( 'NONE', *, *, #7533, .F. ) ;
#12812=VERTEX_POINT ( 'NONE', #11064 ) ;
#12822=FACE_BOUND ( 'NONE', #22972, .T. ) ;
#12823=CARTESIAN_POINT ( 'NONE',  ( 166.1922820468853388, -9.999999999999998224, -13.59645775552055902 ) ) ;
#12824=AXIS2_PLACEMENT_3D ( 'NONE', #11113, #9255, #22876 ) ;
#12827=EDGE_LOOP ( 'NONE', ( #5463, #4815, #5348, #16388 ) ) ;
#12828=LINE ( 'NONE', #26589, #22680 ) ;
#12830=EDGE_CURVE ( 'NONE', #7141, #7643, #1632, .T. ) ;
#12831=LINE ( 'NONE', #21843, #22601 ) ;
#12833=DIRECTION ( 'NONE',  ( -0.5877852522924731371, 0.000000000000000000, 0.8090169943749474513 ) ) ;
#12834=VERTEX_POINT ( 'NONE', #29906 ) ;
#12837=VECTOR ( 'NONE', #9208, 1000.000000000000000 ) ;
#12839=CARTESIAN_POINT ( 'NONE',  ( 130.7287565553229456, -4.999999999999983125, 3.500000000000003109 ) ) ;
#12840=DIRECTION ( 'NONE',  ( -2.698458740408365879E-16, 1.000000000000000000, 0.000000000000000000 ) ) ;
#12841=DIRECTION ( 'NONE',  ( -0.5877852522924731371, 0.000000000000000000, 0.8090169943749474513 ) ) ;
#12842=ORIENTED_EDGE ( 'NONE', *, *, #12330, .T. ) ;
#12844=ORIENTED_EDGE ( 'NONE', *, *, #13348, .F. ) ;
#12848=ORIENTED_EDGE ( 'NONE', *, *, #7980, .F. ) ;
#12849=CARTESIAN_POINT ( 'NONE',  ( 154.7287565553229172, -1.999999999999975353, -16.50000000000000000 ) ) ;
#12852=FACE_OUTER_BOUND ( 'NONE', #21719, .T. ) ;
#12853=VECTOR ( 'NONE', #13550, 1000.000000000000000 ) ;
#12856=VERTEX_POINT ( 'NONE', #29759 ) ;
#12857=ORIENTED_EDGE ( 'NONE', *, *, #28067, .F. ) ;
#12859=CARTESIAN_POINT ( 'NONE',  ( 154.5152310637604671, -4.999999999999976019, -4.391296821672111328 ) ) ;
#12860=VECTOR ( 'NONE', #20890, 1000.000000000000000 ) ;
#12862=EDGE_LOOP ( 'NONE', ( #3267, #14773, #7559, #9377 ) ) ;
#12863=LINE ( 'NONE', #20180, #18863 ) ;
#12864=LINE ( 'NONE', #15145, #17001 ) ;
#12869=ORIENTED_EDGE ( 'NONE', *, *, #27136, .T. ) ;
#12873=PLANE ( 'NONE',  #9259 ) ;
#12874=DIRECTION ( 'NONE',  ( -0.5877852522924731371, -1.586114251531760728E-16, -0.8090169943749474513 ) ) ;
#12875=DIRECTION ( 'NONE',  ( 0.5877852522924731371, 1.586114251531760728E-16, 0.8090169943749474513 ) ) ;
#12878=DIRECTION ( 'NONE',  ( 0.9510565162951536422, 2.566386769018988816E-16, 0.3090169943749472292 ) ) ;
#12880=DIRECTION ( 'NONE',  ( 0.000000000000000000, 0.000000000000000000, -1.000000000000000000 ) ) ;
#12881=LINE ( 'NONE', #1014, #8343 ) ;
#12883=AXIS2_PLACEMENT_3D ( 'NONE', #12602, #28384, #1031 ) ;
#12884=FACE_OUTER_BOUND ( 'NONE', #28690, .T. ) ;
#12886=ORIENTED_EDGE ( 'NONE', *, *, #27766, .T. ) ;
#12887=CARTESIAN_POINT ( 'NONE',  ( 132.0152310637605808, -10.00000000000000711, 1.702185954127501066 ) ) ;
#12891=EDGE_CURVE ( 'NONE', #23695, #22008, #6498, .T. ) ;
#12895=EDGE_CURVE ( 'NONE', #3997, #6165, #20219, .T. ) ;
#12896=EDGE_CURVE ( 'NONE', #983, #2523, #17922, .T. ) ;
#12897=CARTESIAN_POINT ( 'NONE',  ( 162.2287565553228887, -10.00000000000000000, -3.509618943233403510 ) ) ;
#12898=ORIENTED_EDGE ( 'NONE', *, *, #16900, .T. ) ;
#12899=DIRECTION ( 'NONE',  ( 1.000000000000000000, 2.698458740408365879E-16, -1.110223024625156540E-16 ) ) ;
#12900=LINE ( 'NONE', #7881, #23785 ) ;
#12901=LINE ( 'NONE', #1633, #24096 ) ;
#12902=VECTOR ( 'NONE', #25833, 1000.000000000000000 ) ;
#12903=FACE_OUTER_BOUND ( 'NONE', #16260, .T. ) ;
#12905=CARTESIAN_POINT ( 'NONE',  ( 147.0152310637604955, -1.999999999999977573, -0.06116980274991495881 ) ) ;
#12907=CARTESIAN_POINT ( 'NONE',  ( 157.2287565553229740, -1.999999999999973577, -20.83012701892220520 ) ) ;
#12909=CARTESIAN_POINT ( 'NONE',  ( 162.2287565553229740, -9.999999999999998224, -29.49038105676660493 ) ) ;
#12912=DIRECTION ( 'NONE',  ( 0.000000000000000000, -1.000000000000000000, 0.000000000000000000 ) ) ;
#12913=LINE ( 'NONE', #5914, #17324 ) ;
#12915=VECTOR ( 'NONE', #12004, 1000.000000000000000 ) ;
#12917=CARTESIAN_POINT ( 'NONE',  ( 19.74162731500053525, -5.000000000000012434, -60.75848138442648860 ) ) ;
#12918=DIRECTION ( 'NONE',  ( -2.698458740408365879E-16, 1.000000000000000000, 0.000000000000000000 ) ) ;
#12919=LINE ( 'NONE', #10175, #15124 ) ;
#12925=DIRECTION ( 'NONE',  ( 0.9510565162951536422, 0.000000000000000000, -0.3090169943749475623 ) ) ;
#12926=PLANE ( 'NONE',  #17951 ) ;
#12927=VECTOR ( 'NONE', #25496, 1000.000000000000000 ) ;
#12928=CARTESIAN_POINT ( 'NONE',  ( 130.7287565553229456, -9.999999999999982236, 3.500000000000003109 ) ) ;
#12929=EDGE_CURVE ( 'NONE', #2363, #10720, #6800, .T. ) ;
#12930=EDGE_CURVE ( 'NONE', #966, #18633, #27739, .T. ) ;
#12931=EDGE_CURVE ( 'NONE', #2910, #23077, #27133, .T. ) ;
#12932=VERTEX_POINT ( 'NONE', #18952 ) ;
#12933=EDGE_CURVE ( 'NONE', #24767, #11084, #944, .T. ) ;
#12934=DIRECTION ( 'NONE',  ( -0.8090169943749474513, -2.183098979609982436E-16, -0.5877852522924731371 ) ) ;
#12935=ORIENTED_EDGE ( 'NONE', *, *, #3148, .T. ) ;
#12938=ORIENTED_EDGE ( 'NONE', *, *, #22704, .T. ) ;
#12939=DIRECTION ( 'NONE',  ( -2.698458740408365879E-16, 1.000000000000000000, 0.000000000000000000 ) ) ;
#12941=VECTOR ( 'NONE', #23168, 1000.000000000000000 ) ;
#12944=EDGE_LOOP ( 'NONE', ( #15621, #15032, #1978, #3904, #14079 ) ) ;
#12945=VECTOR ( 'NONE', #17051, 1000.000000000000000 ) ;
#12947=ORIENTED_EDGE ( 'NONE', *, *, #26743, .F. ) ;
#12950=FACE_BOUND ( 'NONE', #1900, .T. ) ;
#12951=ORIENTED_EDGE ( 'NONE', *, *, #22881, .T. ) ;
#12952=ORIENTED_EDGE ( 'NONE', *, *, #2530, .T. ) ;
#12953=LINE ( 'NONE', #6249, #27260 ) ;
#12955=CARTESIAN_POINT ( 'NONE',  ( 137.0152310637605808, -10.00000000000000533, -17.38167787843870826 ) ) ;
#12956=ORIENTED_EDGE ( 'NONE', *, *, #12216, .F. ) ;
#12957=FACE_OUTER_BOUND ( 'NONE', #7639, .T. ) ;
#12958=ORIENTED_EDGE ( 'NONE', *, *, #19776, .F. ) ;
#12960=ADVANCED_FACE ( 'NONE', ( #9634 ), #2947, .T. ) ;
#12961=ORIENTED_EDGE ( 'NONE', *, *, #11114, .F. ) ;
#12964=AXIS2_PLACEMENT_3D ( 'NONE', #19301, #699, #7266 ) ;
#12965=LINE ( 'NONE', #21670, #16957 ) ;
#12968=EDGE_LOOP ( 'NONE', ( #11258, #7780, #19604, #10021 ) ) ;
#12969=VECTOR ( 'NONE', #7560, 1000.000000000000000 ) ;
#12971=ADVANCED_FACE ( 'NONE', ( #21839 ), #5520, .T. ) ;
#12972=ADVANCED_FACE ( 'NONE', ( #14656 ), #10231, .T. ) ;
#12973=AXIS2_PLACEMENT_3D ( 'NONE', #28505, #5265, #14553 ) ;
#12975=LINE ( 'NONE', #10979, #16416 ) ;
#12977=DIRECTION ( 'NONE',  ( 1.000000000000000000, 2.698458740408365879E-16, 0.000000000000000000 ) ) ;
#12979=DIRECTION ( 'NONE',  ( -2.698458740408365879E-16, 1.000000000000000000, 0.000000000000000000 ) ) ;
#12983=CARTESIAN_POINT ( 'NONE',  ( 175.7287565553229456, -4.999999999999970690, -2.233642730705308832 ) ) ;
#12987=EDGE_LOOP ( 'NONE', ( #28931, #18381, #3999, #21879 ) ) ;
#12988=VECTOR ( 'NONE', #25243, 1000.000000000000000 ) ;
#12990=ORIENTED_EDGE ( 'NONE', *, *, #22628, .F. ) ;
#12992=AXIS2_PLACEMENT_3D ( 'NONE', #15561, #29367, #10686 ) ;
#12994=DIRECTION ( 'NONE',  ( 0.9510565162951536422, 0.000000000000000000, -0.3090169943749475623 ) ) ;
#12995=DIRECTION ( 'NONE',  ( -2.698458740408365879E-16, 1.000000000000000000, 0.000000000000000000 ) ) ;
#12996=ORIENTED_EDGE ( 'NONE', *, *, #11516, .F. ) ;
#12997=CARTESIAN_POINT ( 'NONE',  ( 174.5152310637603819, -1.999999999999970024, -4.391296821672111328 ) ) ;
#12998=ORIENTED_EDGE ( 'NONE', *, *, #2348, .T. ) ;
#13004=DIRECTION ( 'NONE',  ( -0.5877852522924731371, 0.000000000000000000, 0.8090169943749474513 ) ) ;
#13008=EDGE_CURVE ( 'NONE', #23323, #357, #14350, .T. ) ;
#13009=EDGE_CURVE ( 'NONE', #17627, #29771, #21541, .T. ) ;
#13010=VERTEX_POINT ( 'NONE', #5059 ) ;
#13011=EDGE_CURVE ( 'NONE', #29392, #2975, #23687, .T. ) ;
#13012=ORIENTED_EDGE ( 'NONE', *, *, #27134, .F. ) ;
#13013=ORIENTED_EDGE ( 'NONE', *, *, #31, .T. ) ;
#13014=LINE ( 'NONE', #24325, #10326 ) ;
#13015=VECTOR ( 'NONE', #22123, 1000.000000000000000 ) ;
#13016=DIRECTION ( 'NONE',  ( -2.698458740408365879E-16, 1.000000000000000000, 0.000000000000000000 ) ) ;
#13018=PLANE ( 'NONE',  #9087 ) ;
#13019=FACE_OUTER_BOUND ( 'NONE', #7540, .T. ) ;
#13022=ORIENTED_EDGE ( 'NONE', *, *, #29829, .F. ) ;
#13026=DIRECTION ( 'NONE',  ( -0.9510565162951536422, 0.000000000000000000, -0.3090169943749472292 ) ) ;
#13027=DIRECTION ( 'NONE',  ( -0.9510565162951536422, -2.566386769018988816E-16, -0.3090169943749472292 ) ) ;
#13028=ORIENTED_EDGE ( 'NONE', *, *, #5468, .F. ) ;
#13030=FACE_OUTER_BOUND ( 'NONE', #23860, .T. ) ;
#13031=LINE ( 'NONE', #21892, #996 ) ;
#13033=ORIENTED_EDGE ( 'NONE', *, *, #7370, .T. ) ;
#13035=FACE_OUTER_BOUND ( 'NONE', #27560, .T. ) ;
#13038=AXIS2_PLACEMENT_3D ( 'NONE', #18819, #28178, #665 ) ;
#13039=FACE_OUTER_BOUND ( 'NONE', #7870, .T. ) ;
#13040=LINE ( 'NONE', #15919, #24938 ) ;
#13042=DIRECTION ( 'NONE',  ( 0.9510565162951535312, 2.566386769018988816E-16, -0.3090169943749475623 ) ) ;
#13044=VERTEX_POINT ( 'NONE', #14507 ) ;
#13049=AXIS2_PLACEMENT_3D ( 'NONE', #22121, #7925, #5494 ) ;
#13050=LINE ( 'NONE', #13350, #3095 ) ;
#13051=CARTESIAN_POINT ( 'NONE',  ( 152.0152310637604671, -10.00000000000000178, -0.06116980274991495881 ) ) ;
#13055=DIRECTION ( 'NONE',  ( 8.163404592832029035E-16, 0.000000000000000000, 1.000000000000000000 ) ) ;
#13059=AXIS2_PLACEMENT_3D ( 'NONE', #3834, #10983, #13285 ) ;
#13060=DIRECTION ( 'NONE',  ( 0.3090169943749472292, 8.338696094057992503E-17, -0.9510565162951536422 ) ) ;
#13062=DIRECTION ( 'NONE',  ( -2.698458740408365879E-16, 1.000000000000000000, 0.000000000000000000 ) ) ;
#13063=DIRECTION ( 'NONE',  ( -0.5877852522924731371, -1.586114251531760235E-16, 0.8090169943749474513 ) ) ;
#13065=LINE ( 'NONE', #15801, #13163 ) ;
#13066=VERTEX_POINT ( 'NONE', #12519 ) ;
#13067=DIRECTION ( 'NONE',  ( -0.5877852522924731371, -1.586114251531760235E-16, 0.8090169943749474513 ) ) ;
#13069=EDGE_CURVE ( 'NONE', #6853, #7751, #26286, .T. ) ;
#13070=VERTEX_POINT ( 'NONE', #26135 ) ;
#13071=PLANE ( 'NONE',  #30069 ) ;
#13072=PLANE ( 'NONE',  #28375 ) ;
#13073=EDGE_CURVE ( 'NONE', #3516, #23103, #10078, .T. ) ;
#13082=FACE_OUTER_BOUND ( 'NONE', #15473, .T. ) ;
#13083=PLANE ( 'NONE',  #18968 ) ;
#13085=VERTEX_POINT ( 'NONE', #7654 ) ;
#13088=LINE ( 'NONE', #11658, #22455 ) ;
#13089=CARTESIAN_POINT ( 'NONE',  ( 122.2076721278953642, -4.999999999999984901, -88.78907104945136552 ) ) ;
#13092=AXIS2_PLACEMENT_3D ( 'NONE', #17439, #26792, #5863 ) ;
#13093=ORIENTED_EDGE ( 'NONE', *, *, #22031, .T. ) ;
#13095=VERTEX_POINT ( 'NONE', #28597 ) ;
#13098=FACE_BOUND ( 'NONE', #28343, .T. ) ;
#13102=ORIENTED_EDGE ( 'NONE', *, *, #11792, .T. ) ;
#13103=CARTESIAN_POINT ( 'NONE',  ( 130.7287565553229456, -4.999999999999983125, -2.233642730705363455 ) ) ;
#13106=LINE ( 'NONE', #8824, #14502 ) ;
#13107=EDGE_CURVE ( 'NONE', #9848, #14997, #20813, .T. ) ;
#13108=ORIENTED_EDGE ( 'NONE', *, *, #29078, .F. ) ;
#13110=ORIENTED_EDGE ( 'NONE', *, *, #25877, .T. ) ;
#13116=EDGE_LOOP ( 'NONE', ( #28427, #4180, #22196, #855 ) ) ;
#13119=ORIENTED_EDGE ( 'NONE', *, *, #27691, .F. ) ;
#13122=LINE ( 'NONE', #17549, #10068 ) ;
#13123=FACE_BOUND ( 'NONE', #28827, .T. ) ;
#13124=ORIENTED_EDGE ( 'NONE', *, *, #12931, .F. ) ;
#13125=LINE ( 'NONE', #22600, #17194 ) ;
#13127=DIRECTION ( 'NONE',  ( -2.698458740408365879E-16, 1.000000000000000000, 0.000000000000000000 ) ) ;
#13128=ORIENTED_EDGE ( 'NONE', *, *, #27, .F. ) ;
#13130=DIRECTION ( 'NONE',  ( -2.698458740408365879E-16, 1.000000000000000000, 0.000000000000000000 ) ) ;
#13136=PLANE ( 'NONE',  #4410 ) ;
#13137=EDGE_CURVE ( 'NONE', #25794, #13010, #14029, .T. ) ;
#13139=DIRECTION ( 'NONE',  ( -0.5877852522924731371, -1.586114251531760235E-16, 0.8090169943749474513 ) ) ;
#13140=LINE ( 'NONE', #8556, #3761 ) ;
#13141=EDGE_CURVE ( 'NONE', #14190, #12612, #17891, .T. ) ;
#13142=ADVANCED_FACE ( 'NONE', ( #4175 ), #28127, .T. ) ;
#13144=ORIENTED_EDGE ( 'NONE', *, *, #27871, .F. ) ;
#13145=VECTOR ( 'NONE', #29758, 1000.000000000000000 ) ;
#13147=EDGE_CURVE ( 'NONE', #27090, #7113, #22799, .T. ) ;
#13154=VERTEX_POINT ( 'NONE', #2473 ) ;
#13155=CARTESIAN_POINT ( 'NONE',  ( 136.1922820468854241, -1.999999999999980460, -4.936203717676158398 ) ) ;
#13156=CARTESIAN_POINT ( 'NONE',  ( 161.1922820468853956, -1.999999999999972244, -28.06379628232387802 ) ) ;
#13157=DIRECTION ( 'NONE',  ( 0.5877852522924731371, 1.586114251531760728E-16, 0.8090169943749474513 ) ) ;
#13161=ORIENTED_EDGE ( 'NONE', *, *, #7705, .T. ) ;
#13162=DIRECTION ( 'NONE',  ( -2.698458740408365879E-16, 1.000000000000000000, 0.000000000000000000 ) ) ;
#13163=VECTOR ( 'NONE', #24990, 1000.000000000000000 ) ;
#13164=VECTOR ( 'NONE', #7089, 1000.000000000000000 ) ;
#13165=LINE ( 'NONE', #18458, #1427 ) ;
#13166=CARTESIAN_POINT ( 'NONE',  ( 159.7287565553229740, -9.999999999999998224, -25.16025403784440329 ) ) ;
#13167=DIRECTION ( 'NONE',  ( -2.698458740408365879E-16, 1.000000000000000000, 0.000000000000000000 ) ) ;
#13168=FACE_OUTER_BOUND ( 'NONE', #8210, .T. ) ;
#13169=CARTESIAN_POINT ( 'NONE',  ( 137.2287565553230309, -1.999999999999979572, -3.509618943233403510 ) ) ;
#13172=LINE ( 'NONE', #13464, #23387 ) ;
#13174=VERTEX_POINT ( 'NONE', #4031 ) ;
#13175=PLANE ( 'NONE',  #13938 ) ;
#13177=EDGE_LOOP ( 'NONE', ( #12357, #3246, #19786, #12257, #14683 ) ) ;
#13179=EDGE_CURVE ( 'NONE', #6891, #4371, #11592, .T. ) ;
#13180=DIRECTION ( 'NONE',  ( -0.8090169943749474513, -2.183098979609982436E-16, 0.5877852522924731371 ) ) ;
#13181=DIRECTION ( 'NONE',  ( 0.5877852522924731371, 1.586114251531760728E-16, 0.8090169943749474513 ) ) ;
#13183=EDGE_CURVE ( 'NONE', #30043, #29696, #29729, .T. ) ;
#13185=ORIENTED_EDGE ( 'NONE', *, *, #9665, .F. ) ;
#13187=DIRECTION ( 'NONE',  ( -0.8090169943749474513, -2.183098979609982436E-16, -0.5877852522924731371 ) ) ;
#13188=EDGE_CURVE ( 'NONE', #30193, #8651, #22649, .T. ) ;
#13190=AXIS2_PLACEMENT_3D ( 'NONE', #5435, #19606, #10446 ) ;
#13191=LINE ( 'NONE', #17900, #25180 ) ;
#13194=DIRECTION ( 'NONE',  ( -2.698458740408365879E-16, 1.000000000000000000, 0.000000000000000000 ) ) ;
#13196=VERTEX_POINT ( 'NONE', #1749 ) ;
#13197=FACE_OUTER_BOUND ( 'NONE', #14071, .T. ) ;
#13198=ORIENTED_EDGE ( 'NONE', *, *, #2349, .T. ) ;
#13199=PRESENTATION_STYLE_ASSIGNMENT (( #27123 ) ) ;
#13202=ORIENTED_EDGE ( 'NONE', *, *, #6639, .F. ) ;
#13203=ORIENTED_EDGE ( 'NONE', *, *, #5670, .T. ) ;
#13204=VECTOR ( 'NONE', #4079, 1000.000000000000000 ) ;
#13207=LINE ( 'NONE', #24513, #7493 ) ;
#13208=EDGE_CURVE ( 'NONE', #10971, #16231, #16328, .T. ) ;
#13209=PLANE ( 'NONE',  #20462 ) ;
#13211=LINE ( 'NONE', #24671, #712 ) ;
#13212=DIRECTION ( 'NONE',  ( 0.5877852522924731371, 1.586114251531760728E-16, -0.8090169943749474513 ) ) ;
#13218=CARTESIAN_POINT ( 'NONE',  ( 153.6922820468854241, -10.00000000000000000, -23.73366926340167637 ) ) ;
#13219=DIRECTION ( 'NONE',  ( -0.8090169943749474513, -2.183098979609982436E-16, -0.5877852522924731371 ) ) ;
#13222=VERTEX_POINT ( 'NONE', #9304 ) ;
#13223=DIRECTION ( 'NONE',  ( 1.110223024625156540E-16, 2.995891024602366092E-32, 1.000000000000000000 ) ) ;
#13225=AXIS2_PLACEMENT_3D ( 'NONE', #12909, #14586, #12305 ) ;
#13227=VECTOR ( 'NONE', #14854, 1000.000000000000000 ) ;
#13229=AXIS2_PLACEMENT_3D ( 'NONE', #21603, #25249, #24960 ) ;
#13230=LINE ( 'NONE', #10631, #6634 ) ;
#13231=DIRECTION ( 'NONE',  ( -0.9510565162951536422, -2.566386769018988323E-16, 0.3090169943749475623 ) ) ;
#13232=DIRECTION ( 'NONE',  ( -0.8090169943749474513, -2.183098979609982436E-16, 0.5877852522924731371 ) ) ;
#13234=ORIENTED_EDGE ( 'NONE', *, *, #20027, .F. ) ;
#13237=ORIENTED_EDGE ( 'NONE', *, *, #29578, .T. ) ;
#13240=LINE ( 'NONE', #15358, #8711 ) ;
#13241=LINE ( 'NONE', #20105, #20891 ) ;
#13244=EDGE_LOOP ( 'NONE', ( #6576, #26668, #4811, #23653, #12553 ) ) ;
#13245=DIRECTION ( 'NONE',  ( 0.9510565162951535312, 2.566386769018988816E-16, -0.3090169943749475623 ) ) ;
#13246=EDGE_CURVE ( 'NONE', #220, #7982, #7338, .T. ) ;
#13247=LINE ( 'NONE', #1818, #9712 ) ;
#13248=EDGE_CURVE ( 'NONE', #28330, #24722, #27417, .T. ) ;
#13249=DIRECTION ( 'NONE',  ( -2.698458740408365879E-16, 1.000000000000000000, 0.000000000000000000 ) ) ;
#13250=FACE_OUTER_BOUND ( 'NONE', #10443, .T. ) ;
#13253=VERTEX_POINT ( 'NONE', #21065 ) ;
#13256=VERTEX_POINT ( 'NONE', #10881 ) ;
#13259=FACE_OUTER_BOUND ( 'NONE', #7494, .T. ) ;
#13260=ORIENTED_EDGE ( 'NONE', *, *, #29249, .F. ) ;
#13261=ORIENTED_EDGE ( 'NONE', *, *, #13183, .T. ) ;
#13262=CARTESIAN_POINT ( 'NONE',  ( 176.1922820468852535, -9.999999999999994671, -4.936203717676158398 ) ) ;
#13265=LINE ( 'NONE', #29351, #12067 ) ;
#13266=ORIENTED_EDGE ( 'NONE', *, *, #12648, .T. ) ;
#13267=DIRECTION ( 'NONE',  ( 0.3090169943749475623, 8.338696094058001131E-17, 0.9510565162951536422 ) ) ;
#13273=DIRECTION ( 'NONE',  ( 0.5877852522924731371, 0.000000000000000000, 0.8090169943749474513 ) ) ;
#13275=VECTOR ( 'NONE', #25784, 1000.000000000000000 ) ;
#13276=ORIENTED_EDGE ( 'NONE', *, *, #30084, .F. ) ;
#13277=FACE_OUTER_BOUND ( 'NONE', #27913, .T. ) ;
#13278=ADVANCED_FACE ( 'NONE', ( #20192 ), #15617, .T. ) ;
#13280=EDGE_CURVE ( 'NONE', #21455, #4011, #18774, .T. ) ;
#13281=ADVANCED_FACE ( 'NONE', ( #6470 ), #15761, .T. ) ;
#13282=VECTOR ( 'NONE', #7904, 1000.000000000000000 ) ;
#13283=ADVANCED_FACE ( 'NONE', ( #23508 ), #11891, .T. ) ;
#13284=DIRECTION ( 'NONE',  ( -2.698458740408365879E-16, 1.000000000000000000, 0.000000000000000000 ) ) ;
#13285=DIRECTION ( 'NONE',  ( -0.9510565162951536422, 0.000000000000000000, -0.3090169943749472292 ) ) ;
#13286=DIRECTION ( 'NONE',  ( 2.908569913943825061E-16, -1.000000000000000000, -6.826925868028081731E-18 ) ) ;
#13287=ORIENTED_EDGE ( 'NONE', *, *, #9887, .T. ) ;
#13288=FACE_OUTER_BOUND ( 'NONE', #24273, .T. ) ;
#13291=EDGE_LOOP ( 'NONE', ( #13093, #25160, #7552, #26672 ) ) ;
#13292=LINE ( 'NONE', #1709, #10737 ) ;
#13295=LINE ( 'NONE', #23070, #5236 ) ;
#13297=CARTESIAN_POINT ( 'NONE',  ( 13.86283076467578113, -5.000000000000014211, 42.66540602308926111 ) ) ;
#13298=EDGE_LOOP ( 'NONE', ( #13565, #25765, #3460, #9990, #27341 ) ) ;
#13305=LINE ( 'NONE', #22779, #23501 ) ;
#13311=ADVANCED_FACE ( 'NONE', ( #3071 ), #2766, .T. ) ;
#13314=CARTESIAN_POINT ( 'NONE',  ( 138.6922820468854525, -10.00000000000000533, -35.24709285013155835 ) ) ;
#13315=CARTESIAN_POINT ( 'NONE',  ( 175.7287565553229456, -4.999999999999970690, 3.500000000000003109 ) ) ;
#13316=CARTESIAN_POINT ( 'NONE',  ( 139.7287565553230309, -10.00000000000000533, -16.50000000000000000 ) ) ;
#13317=VECTOR ( 'NONE', #27582, 999.9999999999998863 ) ;
#13321=CARTESIAN_POINT ( 'NONE',  ( 159.5152310637604671, -1.999999999999973577, -13.05155085951651195 ) ) ;
#13325=CARTESIAN_POINT ( 'NONE',  ( 173.6922820468853672, -9.999999999999994671, -32.39392330124607611 ) ) ;
#13326=CARTESIAN_POINT ( 'NONE',  ( 144.7287565553229740, -1.999999999999978018, 0.8205080756887930260 ) ) ;
#13327=LINE ( 'NONE', #6473, #24471 ) ;
#13330=ORIENTED_EDGE ( 'NONE', *, *, #25451, .T. ) ;
#13333=AXIS2_PLACEMENT_3D ( 'NONE', #20861, #18434, #4404 ) ;
#13335=DIRECTION ( 'NONE',  ( -0.9510565162951536422, 0.000000000000000000, -0.3090169943749472292 ) ) ;
#13336=EDGE_LOOP ( 'NONE', ( #17770, #3888, #28477, #10945 ) ) ;
#13341=DIRECTION ( 'NONE',  ( 0.5877852522924731371, 1.586114251531760728E-16, -0.8090169943749474513 ) ) ;
#13344=VECTOR ( 'NONE', #21644, 1000.000000000000000 ) ;
#13345=ORIENTED_EDGE ( 'NONE', *, *, #9404, .F. ) ;
#13346=DIRECTION ( 'NONE',  ( -0.9510565162951536422, -2.566386769018988323E-16, 0.3090169943749475623 ) ) ;
#13347=EDGE_CURVE ( 'NONE', #7328, #12130, #758, .T. ) ;
#13348=EDGE_CURVE ( 'NONE', #16735, #12932, #5036, .T. ) ;
#13349=EDGE_CURVE ( 'NONE', #12321, #7426, #5492, .T. ) ;
#13350=CARTESIAN_POINT ( 'NONE',  ( 169.5152310637604671, -1.999999999999970912, -11.28819510263909542 ) ) ;
#13351=EDGE_CURVE ( 'NONE', #23086, #10981, #26562, .T. ) ;
#13352=ORIENTED_EDGE ( 'NONE', *, *, #26083, .F. ) ;
#13355=LINE ( 'NONE', #22679, #15315 ) ;
#13360=CARTESIAN_POINT ( 'NONE',  ( 146.1922820468854525, -10.00000000000000178, -30.91696583120935671 ) ) ;
#13362=VECTOR ( 'NONE', #5751, 1000.000000000000000 ) ;
#13363=DIRECTION ( 'NONE',  ( 0.3090169943749475623, 8.338696094058001131E-17, 0.9510565162951536422 ) ) ;
#13364=CARTESIAN_POINT ( 'NONE',  ( 164.5152310637604671, -4.999999999999973355, -13.05155085951651195 ) ) ;
#13367=ORIENTED_EDGE ( 'NONE', *, *, #2826, .F. ) ;
#13370=ORIENTED_EDGE ( 'NONE', *, *, #20369, .T. ) ;
#13372=LINE ( 'NONE', #29926, #21961 ) ;
#13373=FACE_OUTER_BOUND ( 'NONE', #24449, .T. ) ;
#13375=ORIENTED_EDGE ( 'NONE', *, *, #13348, .T. ) ;
#13380=CARTESIAN_POINT ( 'NONE',  ( 115.6625871560206491, -4.999999999999985789, -84.03378846797562574 ) ) ;
#13381=CARTESIAN_POINT ( 'NONE',  ( 138.6922820468854525, -1.999999999999979572, -9.266330736598359152 ) ) ;
#13383=VECTOR ( 'NONE', #15749, 1000.000000000000000 ) ;
#13384=EDGE_LOOP ( 'NONE', ( #10372, #3184, #28399, #27269, #11930 ) ) ;
#13385=EDGE_CURVE ( 'NONE', #9036, #475, #3215, .T. ) ;
#13386=CARTESIAN_POINT ( 'NONE',  ( 143.6922820468854525, -1.999999999999978018, -26.58683881228715506 ) ) ;
#13387=ADVANCED_FACE ( 'NONE', ( #470 ), #12492, .T. ) ;
#13388=CARTESIAN_POINT ( 'NONE',  ( 139.7287565553230309, -1.999999999999978684, -33.82050807568879947 ) ) ;
#13392=PLANE ( 'NONE',  #676 ) ;
#13393=CARTESIAN_POINT ( 'NONE',  ( 169.5152310637604387, -1.999999999999970912, -13.05155085951651195 ) ) ;
#13395=EDGE_LOOP ( 'NONE', ( #6754, #7544, #19846, #18987, #8186 ) ) ;
#13397=ORIENTED_EDGE ( 'NONE', *, *, #23769, .T. ) ;
#13399=CARTESIAN_POINT ( 'NONE',  ( 177.2287565553228603, -1.999999999999968914, -12.16987298107780369 ) ) ;
#13401=PLANE ( 'NONE',  #3900 ) ;
#13402=VERTEX_POINT ( 'NONE', #916 ) ;
#13403=DIRECTION ( 'NONE',  ( -1.110223024625156540E-16, 0.000000000000000000, -1.000000000000000000 ) ) ;
#13404=EDGE_LOOP ( 'NONE', ( #28964, #27680, #2463, #23073 ) ) ;
#13405=VECTOR ( 'NONE', #22755, 1000.000000000000000 ) ;
#13406=DIRECTION ( 'NONE',  ( 0.000000000000000000, -1.000000000000000000, 0.000000000000000000 ) ) ;
#13408=VERTEX_POINT ( 'NONE', #12650 ) ;
#13410=ORIENTED_EDGE ( 'NONE', *, *, #4465, .T. ) ;
#13415=CARTESIAN_POINT ( 'NONE',  ( 149.5152310637605808, -1.999999999999975797, -19.94844914048349693 ) ) ;
#13416=LINE ( 'NONE', #24891, #12780 ) ;
#13418=VERTEX_POINT ( 'NONE', #28892 ) ;
#13420=DIRECTION ( 'NONE',  ( 0.3090169943749472292, 8.338696094057992503E-17, -0.9510565162951536422 ) ) ;
#13421=VECTOR ( 'NONE', #19628, 1000.000000000000000 ) ;
#13422=VECTOR ( 'NONE', #21508, 1000.000000000000000 ) ;
#13423=ORIENTED_EDGE ( 'NONE', *, *, #20443, .F. ) ;
#13426=PLANE ( 'NONE',  #985 ) ;
#13427=ORIENTED_EDGE ( 'NONE', *, *, #13852, .T. ) ;
#13428=ORIENTED_EDGE ( 'NONE', *, *, #24738, .T. ) ;
#13429=CARTESIAN_POINT ( 'NONE',  ( 164.5152310637604955, -1.999999999999971800, -19.94844914048349693 ) ) ;
#13432=CARTESIAN_POINT ( 'NONE',  ( 147.0152310637605240, -4.999999999999977796, -1.632196944975744790E-14 ) ) ;
#13434=ORIENTED_EDGE ( 'NONE', *, *, #10502, .F. ) ;
#13436=VECTOR ( 'NONE', #7000, 1000.000000000000000 ) ;
#13438=DIRECTION ( 'NONE',  ( -0.5877852522924731371, 0.000000000000000000, 0.8090169943749474513 ) ) ;
#13439=DIRECTION ( 'NONE',  ( -2.698458740408365879E-16, 1.000000000000000000, 0.000000000000000000 ) ) ;
#13440=LINE ( 'NONE', #6442, #16412 ) ;
#13445=VECTOR ( 'NONE', #20987, 1000.000000000000000 ) ;
#13450=CARTESIAN_POINT ( 'NONE',  ( 159.5152310637605524, -9.999999999999998224, -28.60870317832789667 ) ) ;
#13456=AXIS2_PLACEMENT_3D ( 'NONE', #4665, #4816, #13958 ) ;
#13457=ADVANCED_BREP_SHAPE_REPRESENTATION ( '', ( #21992, #13190 ), #7783 ) ;
#13458=CARTESIAN_POINT ( 'NONE',  ( 177.2287565553228887, -1.999999999999968470, -20.83012701892220520 ) ) ;
#13459=CARTESIAN_POINT ( 'NONE',  ( 169.7287565553228603, -1.999999999999971356, 0.8205080756887930260 ) ) ;
#13460=VECTOR ( 'NONE', #27424, 1000.000000000000000 ) ;
#13461=CARTESIAN_POINT ( 'NONE',  ( 172.0152310637604387, -9.999999999999996447, -6.958068083716895558 ) ) ;
#13462=VECTOR ( 'NONE', #24741, 1000.000000000000000 ) ;
#13464=CARTESIAN_POINT ( 'NONE',  ( 157.0152310637604671, -1.999999999999974465, -8.721423840594312082 ) ) ;
#13465=ORIENTED_EDGE ( 'NONE', *, *, #20921, .T. ) ;
#13466=DIRECTION ( 'NONE',  ( 0.9510565162951535312, 2.566386769018988816E-16, -0.3090169943749475623 ) ) ;
#13469=DIRECTION ( 'NONE',  ( -0.5877852522924731371, -1.586114251531760235E-16, 0.8090169943749474513 ) ) ;
#13471=PLANE ( 'NONE',  #21461 ) ;
#13472=CARTESIAN_POINT ( 'NONE',  ( 172.0152310637603819, -4.999999999999970690, -0.06116980274991495881 ) ) ;
#13474=VERTEX_POINT ( 'NONE', #19521 ) ;
#13475=ORIENTED_EDGE ( 'NONE', *, *, #3856, .T. ) ;
#13476=LINE ( 'NONE', #11480, #13460 ) ;
#13480=DIRECTION ( 'NONE',  ( 0.3090169943749475623, 8.338696094058001131E-17, 0.9510565162951536422 ) ) ;
#13482=EDGE_CURVE ( 'NONE', #28074, #11734, #7777, .T. ) ;
#13483=AXIS2_PLACEMENT_3D ( 'NONE', #6939, #16232, #21710 ) ;
#13486=EDGE_CURVE ( 'NONE', #16252, #18592, #17234, .T. ) ;
#13489=ORIENTED_EDGE ( 'NONE', *, *, #20169, .F. ) ;
#13490=CARTESIAN_POINT ( 'NONE',  ( 167.2287565553229740, -1.999999999999970468, -29.49038105676660493 ) ) ;
#13492=VECTOR ( 'NONE', #27795, 1000.000000000000000 ) ;
#13494=AXIS2_PLACEMENT_3D ( 'NONE', #8099, #10539, #24149 ) ;
#13495=VERTEX_POINT ( 'NONE', #29029 ) ;
#13497=VECTOR ( 'NONE', #1737, 1000.000000000000000 ) ;
#13499=DIRECTION ( 'NONE',  ( 0.3090169943749475623, 8.338696094058001131E-17, 0.9510565162951536422 ) ) ;
#13501=LINE ( 'NONE', #6497, #1974 ) ;
#13502=LINE ( 'NONE', #6197, #2357 ) ;
#13503=FACE_OUTER_BOUND ( 'NONE', #16485, .T. ) ;
#13508=ADVANCED_FACE ( 'NONE', ( #8067, #12050 ), #1220, .T. ) ;
#13510=LINE ( 'NONE', #20375, #4174 ) ;
#13511=VECTOR ( 'NONE', #20061, 1000.000000000000000 ) ;
#13514=FACE_OUTER_BOUND ( 'NONE', #8565, .T. ) ;
#13516=FACE_OUTER_BOUND ( 'NONE', #5160, .T. ) ;
#13519=AXIS2_PLACEMENT_3D ( 'NONE', #18953, #18496, #16663 ) ;
#13520=ORIENTED_EDGE ( 'NONE', *, *, #23085, .T. ) ;
#13522=DIRECTION ( 'NONE',  ( 1.000000000000000000, 2.698458740408365879E-16, -1.110223024625156540E-16 ) ) ;
#13523=EDGE_CURVE ( 'NONE', #12812, #5460, #12953, .T. ) ;
#13524=DIRECTION ( 'NONE',  ( -2.698458740408365879E-16, 1.000000000000000000, 0.000000000000000000 ) ) ;
#13525=EDGE_CURVE ( 'NONE', #27161, #25583, #901, .T. ) ;
#13527=ORIENTED_EDGE ( 'NONE', *, *, #7768, .F. ) ;
#13528=EDGE_CURVE ( 'NONE', #14964, #2461, #26884, .T. ) ;
#13533=VECTOR ( 'NONE', #17980, 999.9999999999998863 ) ;
#13534=CARTESIAN_POINT ( 'NONE',  ( 159.5152310637604671, -10.00000000000000000, -2.627941064794695691 ) ) ;
#13537=ORIENTED_EDGE ( 'NONE', *, *, #18299, .T. ) ;
#13538=DIRECTION ( 'NONE',  ( 1.000000000000000000, 2.698458740408365879E-16, -1.110223024625156540E-16 ) ) ;
#13539=DIRECTION ( 'NONE',  ( -0.5877852522924731371, -1.586114251531760728E-16, -0.8090169943749474513 ) ) ;
#13541=CARTESIAN_POINT ( 'NONE',  ( 22.28681211727617040, -5.000000000000011546, -68.59175474945887174 ) ) ;
#13542=CARTESIAN_POINT ( 'NONE',  ( 143.6922820468854241, -4.999999999999978684, -6.413161187712876909 ) ) ;
#13543=CARTESIAN_POINT ( 'NONE',  ( 164.7287565553229172, -4.999999999999973355, -7.839745962155600267 ) ) ;
#13545=EDGE_LOOP ( 'NONE', ( #25574, #28734, #20939, #2478 ) ) ;
#13547=ORIENTED_EDGE ( 'NONE', *, *, #27585, .F. ) ;
#13549=DIRECTION ( 'NONE',  ( -2.698458740408365879E-16, 1.000000000000000000, 0.000000000000000000 ) ) ;
#13550=DIRECTION ( 'NONE',  ( -1.110223024625156540E-16, 0.000000000000000000, -1.000000000000000000 ) ) ;
#13552=FACE_BOUND ( 'NONE', #6928, .T. ) ;
#13554=VECTOR ( 'NONE', #8196, 1000.000000000000000 ) ;
#13555=CARTESIAN_POINT ( 'NONE',  ( 144.5152310637605524, -10.00000000000000355, -2.627941064794695691 ) ) ;
#13556=ORIENTED_EDGE ( 'NONE', *, *, #20160, .F. ) ;
#13557=EDGE_CURVE ( 'NONE', #22085, #20929, #17978, .T. ) ;
#13558=LINE ( 'NONE', #18441, #25914 ) ;
#13559=FACE_OUTER_BOUND ( 'NONE', #28434, .T. ) ;
#13560=ORIENTED_EDGE ( 'NONE', *, *, #1589, .T. ) ;
#13562=ORIENTED_EDGE ( 'NONE', *, *, #20073, .F. ) ;
#13565=ORIENTED_EDGE ( 'NONE', *, *, #23106, .T. ) ;
#13566=EDGE_CURVE ( 'NONE', #12292, #28726, #3510, .T. ) ;
#13570=ORIENTED_EDGE ( 'NONE', *, *, #5784, .F. ) ;
#13573=DIRECTION ( 'NONE',  ( -0.9510565162951536422, 0.000000000000000000, -0.3090169943749472292 ) ) ;
#13576=DIRECTION ( 'NONE',  ( 0.5877852522924731371, 0.000000000000000000, 0.8090169943749474513 ) ) ;
#13578=VECTOR ( 'NONE', #26177, 1000.000000000000000 ) ;
#13580=EDGE_LOOP ( 'NONE', ( #15436, #3128, #16656, #8597, #25343 ) ) ;
#13581=ADVANCED_FACE ( 'NONE', ( #10669 ), #22266, .T. ) ;
#13585=DIRECTION ( 'NONE',  ( -0.8090169943749474513, -2.183098979609982436E-16, -0.5877852522924731371 ) ) ;
#13586=ORIENTED_EDGE ( 'NONE', *, *, #9062, .F. ) ;
#13588=DIRECTION ( 'NONE',  ( 0.9510565162951535312, 2.566386769018988816E-16, -0.3090169943749475623 ) ) ;
#13593=ORIENTED_EDGE ( 'NONE', *, *, #9275, .F. ) ;
#13596=DIRECTION ( 'NONE',  ( -0.9510565162951536422, 0.000000000000000000, -0.3090169943749472292 ) ) ;
#13599=ORIENTED_EDGE ( 'NONE', *, *, #17744, .T. ) ;
#13603=DIRECTION ( 'NONE',  ( 0.9510565162951535312, 2.566386769018988816E-16, -0.3090169943749475623 ) ) ;
#13604=VECTOR ( 'NONE', #14849, 1000.000000000000000 ) ;
#13605=LINE ( 'NONE', #22933, #24002 ) ;
#13608=ORIENTED_EDGE ( 'NONE', *, *, #6862, .F. ) ;
#13610=EDGE_CURVE ( 'NONE', #28478, #1397, #27195, .T. ) ;
#13611=CARTESIAN_POINT ( 'NONE',  ( 147.2287565553230309, -1.999999999999976241, -20.83012701892220520 ) ) ;
#13613=CARTESIAN_POINT ( 'NONE',  ( 144.5152310637605808, -10.00000000000000178, -30.37205893520530964 ) ) ;
#13616=VECTOR ( 'NONE', #13539, 1000.000000000000000 ) ;
#13620=ORIENTED_EDGE ( 'NONE', *, *, #26927, .T. ) ;
#13623=LINE ( 'NONE', #7071, #19999 ) ;
#13624=DIRECTION ( 'NONE',  ( 0.3090169943749472292, 8.338696094057992503E-17, -0.9510565162951536422 ) ) ;
#13626=ORIENTED_EDGE ( 'NONE', *, *, #13895, .F. ) ;
#13627=ORIENTED_EDGE ( 'NONE', *, *, #21387, .F. ) ;
#13630=ORIENTED_EDGE ( 'NONE', *, *, #12895, .F. ) ;
#13633=ORIENTED_EDGE ( 'NONE', *, *, #19722, .F. ) ;
#13634=ORIENTED_EDGE ( 'NONE', *, *, #29176, .F. ) ;
#13638=ORIENTED_EDGE ( 'NONE', *, *, #15591, .T. ) ;
#13640=CARTESIAN_POINT ( 'NONE',  ( 129.5152310637605808, -1.999999999999982236, -2.627941064794695691 ) ) ;
#13641=VECTOR ( 'NONE', #4218, 1000.000000000000000 ) ;
#13645=VECTOR ( 'NONE', #15785, 1000.000000000000000 ) ;
#13646=EDGE_LOOP ( 'NONE', ( #3494, #19888, #55, #30236 ) ) ;
#13647=DIRECTION ( 'NONE',  ( -2.698458740408365879E-16, 1.000000000000000000, 0.000000000000000000 ) ) ;
#13650=EDGE_CURVE ( 'NONE', #26271, #1554, #8523, .T. ) ;
#13651=EDGE_CURVE ( 'NONE', #15181, #6555, #29657, .T. ) ;
#13652=LINE ( 'NONE', #4057, #19016 ) ;
#13653=VECTOR ( 'NONE', #693, 1000.000000000000000 ) ;
#13654=DIRECTION ( 'NONE',  ( -0.5877852522924731371, -1.586114251531760235E-16, 0.8090169943749474513 ) ) ;
#13655=EDGE_CURVE ( 'NONE', #22368, #220, #29504, .T. ) ;
#13656=CARTESIAN_POINT ( 'NONE',  ( 169.5152310637605240, -4.999999999999971578, -28.60870317832789667 ) ) ;
#13657=EDGE_CURVE ( 'NONE', #10342, #24640, #10961, .T. ) ;
#13658=LINE ( 'NONE', #22982, #28728 ) ;
#13669=ORIENTED_EDGE ( 'NONE', *, *, #21164, .F. ) ;
#13670=CARTESIAN_POINT ( 'NONE',  ( 110.3859817318374184, -4.999999999999987566, -80.20011022380273857 ) ) ;
#13672=ORIENTED_EDGE ( 'NONE', *, *, #9062, .T. ) ;
#13676=ORIENTED_EDGE ( 'NONE', *, *, #2713, .T. ) ;
#13677=ORIENTED_EDGE ( 'NONE', *, *, #12929, .T. ) ;
#13684=DIRECTION ( 'NONE',  ( 0.9510565162951535312, 2.566386769018988816E-16, -0.3090169943749475623 ) ) ;
#13686=EDGE_CURVE ( 'NONE', #30115, #14294, #19816, .T. ) ;
#13687=ORIENTED_EDGE ( 'NONE', *, *, #22321, .T. ) ;
#13688=DIRECTION ( 'NONE',  ( 1.000000000000000000, 2.698458740408365879E-16, -1.110223024625156540E-16 ) ) ;
#13691=EDGE_CURVE ( 'NONE', #23457, #24548, #17681, .T. ) ;
#13692=DIRECTION ( 'NONE',  ( 0.9510565162951536422, 0.000000000000000000, -0.3090169943749475623 ) ) ;
#13693=EDGE_CURVE ( 'NONE', #17086, #6558, #8373, .T. ) ;
#13694=ADVANCED_FACE ( 'NONE', ( #26723 ), #17826, .T. ) ;
#13695=ADVANCED_FACE ( 'NONE', ( #1533 ), #17528, .T. ) ;
#13696=VECTOR ( 'NONE', #29915, 1000.000000000000000 ) ;
#13697=CARTESIAN_POINT ( 'NONE',  ( 143.6922820468853956, -1.999999999999978684, -0.6060766987539614181 ) ) ;
#13699=VECTOR ( 'NONE', #19157, 1000.000000000000000 ) ;
#13701=VERTEX_POINT ( 'NONE', #2432 ) ;
#13703=DIRECTION ( 'NONE',  ( 0.9510565162951535312, 2.566386769018988816E-16, -0.3090169943749475623 ) ) ;
#13705=FACE_BOUND ( 'NONE', #14146, .T. ) ;
#13706=CARTESIAN_POINT ( 'NONE',  ( 141.1922820468854241, -10.00000000000000533, -4.936203717676158398 ) ) ;
#13707=EDGE_LOOP ( 'NONE', ( #28062, #21462, #29170, #27194, #20363 ) ) ;
#13708=CARTESIAN_POINT ( 'NONE',  ( 134.7287565553230024, -1.999999999999980460, -25.16025403784439973 ) ) ;
#13710=ORIENTED_EDGE ( 'NONE', *, *, #29061, .F. ) ;
#13711=LINE ( 'NONE', #23478, #3303 ) ;
#13712=ORIENTED_EDGE ( 'NONE', *, *, #12510, .F. ) ;
#13717=PLANE ( 'NONE',  #14526 ) ;
#13718=FACE_OUTER_BOUND ( 'NONE', #28314, .T. ) ;
#13719=AXIS2_PLACEMENT_3D ( 'NONE', #25202, #4294, #26916 ) ;
#13721=CARTESIAN_POINT ( 'NONE',  ( 166.1922820468853672, -4.999999999999972466, -19.40354224447947828 ) ) ;
#13722=CARTESIAN_POINT ( 'NONE',  ( 172.7287565553229740, -84.33034373659253902, 8.500000000000003553 ) ) ;
#13723=EDGE_CURVE ( 'NONE', #10764, #26487, #16147, .T. ) ;
#13724=EDGE_CURVE ( 'NONE', #8663, #5681, #15836, .T. ) ;
#13725=EDGE_CURVE ( 'NONE', #8387, #22090, #23475, .T. ) ;
#13726=ADVANCED_FACE ( 'NONE', ( #27496 ), #20713, .T. ) ;
#13730=ORIENTED_EDGE ( 'NONE', *, *, #14021, .F. ) ;
#13731=ORIENTED_EDGE ( 'NONE', *, *, #4156, .F. ) ;
#13733=VECTOR ( 'NONE', #15851, 1000.000000000000000 ) ;
#13738=ORIENTED_EDGE ( 'NONE', *, *, #12554, .F. ) ;
#13741=PLANE ( 'NONE',  #2006 ) ;
#13742=CARTESIAN_POINT ( 'NONE',  ( 133.6922820468854241, -4.999999999999982236, -9.266330736598357376 ) ) ;
#13744=LINE ( 'NONE', #24915, #8610 ) ;
#13745=ORIENTED_EDGE ( 'NONE', *, *, #3481, .F. ) ;
#13750=LINE ( 'NONE', #2184, #29406 ) ;
#13754=VECTOR ( 'NONE', #8504, 1000.000000000000000 ) ;
#13756=CARTESIAN_POINT ( 'NONE',  ( 167.0152310637604103, -9.999999999999998224, -0.06116980274991495881 ) ) ;
#13757=EDGE_CURVE ( 'NONE', #26976, #8129, #7144, .T. ) ;
#13759=CARTESIAN_POINT ( 'NONE',  ( 152.0152310637604671, -1.999999999999976241, -17.38167787843870826 ) ) ;
#13760=AXIS2_PLACEMENT_3D ( 'NONE', #2787, #25826, #14505 ) ;
#13761=CARTESIAN_POINT ( 'NONE',  ( 147.0152310637605808, -10.00000000000000178, -26.04193191628311155 ) ) ;
#13766=PLANE ( 'NONE',  #3279 ) ;
#13769=AXIS2_PLACEMENT_3D ( 'NONE', #14873, #5135, #4984 ) ;
#13771=LINE ( 'NONE', #27869, #16088 ) ;
#13772=CARTESIAN_POINT ( 'NONE',  ( 5.986664691729967736, -5.000000000000015987, 18.42505936432567282 ) ) ;
#13774=ORIENTED_EDGE ( 'NONE', *, *, #16004, .T. ) ;
#13775=ORIENTED_EDGE ( 'NONE', *, *, #14573, .F. ) ;
#13776=DIRECTION ( 'NONE',  ( 0.000000000000000000, 0.000000000000000000, 1.000000000000000000 ) ) ;
#13778=ORIENTED_EDGE ( 'NONE', *, *, #15683, .F. ) ;
#13780=CARTESIAN_POINT ( 'NONE',  ( 154.7287565553230309, -1.999999999999973577, -33.82050807568879947 ) ) ;
#13782=DIRECTION ( 'NONE',  ( -1.110223024625156540E-16, 0.000000000000000000, -1.000000000000000000 ) ) ;
#13784=ORIENTED_EDGE ( 'NONE', *, *, #23336, .F. ) ;
#13785=FACE_OUTER_BOUND ( 'NONE', #11437, .T. ) ;
#13790=DIRECTION ( 'NONE',  ( 0.9510565162951536422, 2.566386769018988816E-16, 0.3090169943749472292 ) ) ;
#13791=VECTOR ( 'NONE', #29244, 1000.000000000000000 ) ;
#13792=PLANE ( 'NONE',  #28981 ) ;
#13794=CARTESIAN_POINT ( 'NONE',  ( 162.0152310637605240, -4.999999999999973355, -24.27857615940569502 ) ) ;
#13795=CARTESIAN_POINT ( 'NONE',  ( 21.17399985718842714, -5.000000000000011546, -65.16687077662002991 ) ) ;
#13802=LINE ( 'NONE', #30209, #3975 ) ;
#13803=LINE ( 'NONE', #16102, #29520 ) ;
#13805=ORIENTED_EDGE ( 'NONE', *, *, #26527, .T. ) ;
#13806=LINE ( 'NONE', #20534, #10525 ) ;
#13808=ORIENTED_EDGE ( 'NONE', *, *, #12172, .F. ) ;
#13809=CARTESIAN_POINT ( 'NONE',  ( 166.1922820468853388, -1.999999999999972244, -13.59645775552055902 ) ) ;
#13810=LINE ( 'NONE', #23444, #26902 ) ;
#13812=VECTOR ( 'NONE', #6795, 1000.000000000000000 ) ;
#13813=VERTEX_POINT ( 'NONE', #13708 ) ;
#13817=EDGE_CURVE ( 'NONE', #27886, #14797, #25599, .T. ) ;
#13818=EDGE_CURVE ( 'NONE', #8784, #563, #20571, .T. ) ;
#13820=EDGE_CURVE ( 'NONE', #18076, #22605, #25169, .T. ) ;
#13822=ADVANCED_FACE ( 'NONE', ( #18440 ), #6855, .T. ) ;
#13823=ORIENTED_EDGE ( 'NONE', *, *, #18902, .T. ) ;
#13827=DIRECTION ( 'NONE',  ( -2.698458740408365879E-16, 1.000000000000000000, 0.000000000000000000 ) ) ;
#13828=ORIENTED_EDGE ( 'NONE', *, *, #9336, .T. ) ;
#13830=VERTEX_POINT ( 'NONE', #2283 ) ;
#13833=DIRECTION ( 'NONE',  ( 1.110223024625156540E-16, 2.995891024602366092E-32, 1.000000000000000000 ) ) ;
#13836=ORIENTED_EDGE ( 'NONE', *, *, #4868, .T. ) ;
#13837=DIRECTION ( 'NONE',  ( -2.698458740408365879E-16, 1.000000000000000000, 0.000000000000000000 ) ) ;
#13840=PLANE ( 'NONE',  #22410 ) ;
#13841=CARTESIAN_POINT ( 'NONE',  ( 129.5152310637605524, -1.999999999999982236, -21.71180489736090991 ) ) ;
#13843=CARTESIAN_POINT ( 'NONE',  ( 24.11769355754544719, -5.000000000000010658, -74.22662841669534828 ) ) ;
#13844=DIRECTION ( 'NONE',  ( 0.5877852522924731371, 1.586114251531760728E-16, -0.8090169943749474513 ) ) ;
#13845=ORIENTED_EDGE ( 'NONE', *, *, #25254, .F. ) ;
#13846=DIRECTION ( 'NONE',  ( 0.9510565162951536422, 0.000000000000000000, -0.3090169943749475623 ) ) ;
#13847=ORIENTED_EDGE ( 'NONE', *, *, #14440, .T. ) ;
#13849=ADVANCED_FACE ( 'NONE', ( #4848 ), #4555, .T. ) ;
#13852=EDGE_CURVE ( 'NONE', #4340, #29774, #14148, .T. ) ;
#13853=VERTEX_POINT ( 'NONE', #22885 ) ;
#13854=EDGE_CURVE ( 'NONE', #5854, #26798, #29956, .T. ) ;
#13856=CARTESIAN_POINT ( 'NONE',  ( 166.1922820468853388, -4.999999999999973355, -13.59645775552055902 ) ) ;
#13858=VECTOR ( 'NONE', #18873, 1000.000000000000000 ) ;
#13863=SURFACE_STYLE_FILL_AREA ( #8979 ) ;
#13865=DIRECTION ( 'NONE',  ( 1.000000000000000000, 2.698458740408365879E-16, -1.110223024625156540E-16 ) ) ;
#13867=CARTESIAN_POINT ( 'NONE',  ( 137.0152310637606092, -10.00000000000000533, -24.27857615940569147 ) ) ;
#13870=CARTESIAN_POINT ( 'NONE',  ( 144.7287565553230309, -10.00000000000000355, -33.82050807568879947 ) ) ;
#13873=EDGE_LOOP ( 'NONE', ( #767, #15256, #29160, #6885 ) ) ;
#13874=LINE ( 'NONE', #29842, #7079 ) ;
#13875=VECTOR ( 'NONE', #13906, 1000.000000000000000 ) ;
#13879=ORIENTED_EDGE ( 'NONE', *, *, #13009, .F. ) ;
#13882=CARTESIAN_POINT ( 'NONE',  ( 11.87405209244401760, -5.000000000000014211, 36.54457464447630599 ) ) ;
#13883=DIRECTION ( 'NONE',  ( -0.8090169943749474513, -2.183098979609982436E-16, 0.5877852522924731371 ) ) ;
#13884=ORIENTED_EDGE ( 'NONE', *, *, #7018, .T. ) ;
#13888=AXIS2_PLACEMENT_3D ( 'NONE', #4842, #7445, #276 ) ;
#13891=EDGE_CURVE ( 'NONE', #23347, #1829, #18132, .T. ) ;
#13892=EDGE_CURVE ( 'NONE', #5942, #134, #23033, .T. ) ;
#13893=DIRECTION ( 'NONE',  ( 0.3090169943749472292, 8.338696094057992503E-17, -0.9510565162951536422 ) ) ;
#13895=EDGE_CURVE ( 'NONE', #633, #9909, #5152, .T. ) ;
#13896=DIRECTION ( 'NONE',  ( -0.5877852522924731371, -1.586114251531760728E-16, -0.8090169943749474513 ) ) ;
#13900=VECTOR ( 'NONE', #2951, 1000.000000000000000 ) ;
#13901=ORIENTED_EDGE ( 'NONE', *, *, #7876, .T. ) ;
#13902=CARTESIAN_POINT ( 'NONE',  ( 172.0152310637604387, -9.999999999999994671, -17.38167787843871182 ) ) ;
#13904=LINE ( 'NONE', #13611, #11083 ) ;
#13905=LINE ( 'NONE', #30166, #30240 ) ;
#13906=DIRECTION ( 'NONE',  ( -2.698458740408365879E-16, 1.000000000000000000, 0.000000000000000000 ) ) ;
#13907=VECTOR ( 'NONE', #17940, 1000.000000000000000 ) ;
#13910=DIRECTION ( 'NONE',  ( -2.698458740408365879E-16, 1.000000000000000000, -0.000000000000000000 ) ) ;
#13911=ORIENTED_EDGE ( 'NONE', *, *, #20819, .T. ) ;
#13912=AXIS2_PLACEMENT_3D ( 'NONE', #21745, #19451, #8895 ) ;
#13914=VECTOR ( 'NONE', #20527, 1000.000000000000000 ) ;
#13917=LINE ( 'NONE', #11782, #10077 ) ;
#13919=ORIENTED_EDGE ( 'NONE', *, *, #16738, .T. ) ;
#13920=VERTEX_POINT ( 'NONE', #432 ) ;
#13921=CARTESIAN_POINT ( 'NONE',  ( 148.6922820468853956, -4.999999999999976907, -9.266330736598359152 ) ) ;
#13924=CARTESIAN_POINT ( 'NONE',  ( 138.6922820468854525, -4.999999999999980460, -32.39392330124607611 ) ) ;
#13926=DIRECTION ( 'NONE',  ( -2.698458740408365879E-16, 1.000000000000000000, 0.000000000000000000 ) ) ;
#13928=ADVANCED_FACE ( 'NONE', ( #26382 ), #7592, .T. ) ;
#13929=ORIENTED_EDGE ( 'NONE', *, *, #24184, .T. ) ;
#13930=EDGE_CURVE ( 'NONE', #21255, #27047, #17201, .T. ) ;
#13931=DIRECTION ( 'NONE',  ( -0.9510565162951536422, -2.566386769018988323E-16, 0.3090169943749475623 ) ) ;
#13934=VECTOR ( 'NONE', #12880, 1000.000000000000000 ) ;
#13935=ORIENTED_EDGE ( 'NONE', *, *, #20854, .F. ) ;
#13936=DIRECTION ( 'NONE',  ( -2.698458740408366372E-16, 1.000000000000000000, 0.000000000000000000 ) ) ;
#13938=AXIS2_PLACEMENT_3D ( 'NONE', #22342, #8293, #22501 ) ;
#13939=CARTESIAN_POINT ( 'NONE',  ( 161.1922820468853672, -9.999999999999998224, -22.25671179336496053 ) ) ;
#13940=CARTESIAN_POINT ( 'NONE',  ( 164.5152310637604955, -1.999999999999971356, -30.37205893520531319 ) ) ;
#13945=EDGE_CURVE ( 'NONE', #1081, #12381, #2880, .T. ) ;
#13950=PLANE ( 'NONE',  #2029 ) ;
#13951=LINE ( 'NONE', #23281, #18293 ) ;
#13952=DIRECTION ( 'NONE',  ( 0.3090169943749472292, 8.338696094057992503E-17, -0.9510565162951536422 ) ) ;
#13956=ORIENTED_EDGE ( 'NONE', *, *, #18943, .F. ) ;
#13957=VECTOR ( 'NONE', #22890, 1000.000000000000000 ) ;
#13958=DIRECTION ( 'NONE',  ( -2.698458740408365879E-16, 1.000000000000000000, 0.000000000000000000 ) ) ;
#13959=DIRECTION ( 'NONE',  ( 0.9510565162951536422, 0.000000000000000000, -0.3090169943749475623 ) ) ;
#13962=EDGE_CURVE ( 'NONE', #20312, #11101, #19185, .T. ) ;
#13963=VERTEX_POINT ( 'NONE', #23945 ) ;
#13968=VECTOR ( 'NONE', #9340, 999.9999999999998863 ) ;
#13969=ORIENTED_EDGE ( 'NONE', *, *, #15442, .F. ) ;
#13970=DIRECTION ( 'NONE',  ( -0.9510565162951536422, -2.566386769018988816E-16, -0.3090169943749472292 ) ) ;
#13971=PLANE ( 'NONE',  #17031 ) ;
#13972=VERTEX_POINT ( 'NONE', #3035 ) ;
#13973=VECTOR ( 'NONE', #21415, 1000.000000000000000 ) ;
#13974=ORIENTED_EDGE ( 'NONE', *, *, #6683, .F. ) ;
#13975=DIRECTION ( 'NONE',  ( -1.110223024625156540E-16, 0.000000000000000000, -1.000000000000000000 ) ) ;
#13976=CARTESIAN_POINT ( 'NONE',  ( 159.5152310637605524, -1.999999999999972689, -28.60870317832789667 ) ) ;
#13977=ADVANCED_FACE ( 'NONE', ( #23784 ), #21783, .T. ) ;
#13980=ADVANCED_FACE ( 'NONE', ( #28691 ), #12009, .T. ) ;
#13981=ORIENTED_EDGE ( 'NONE', *, *, #11117, .F. ) ;
#13983=DIRECTION ( 'NONE',  ( 0.5877852522924731371, 1.586114251531760728E-16, 0.8090169943749474513 ) ) ;
#13984=CARTESIAN_POINT ( 'NONE',  ( 157.0152310637604387, -1.999999999999974909, -0.06116980274991495881 ) ) ;
#13987=DIRECTION ( 'NONE',  ( -2.698458740408365879E-16, 1.000000000000000000, 0.000000000000000000 ) ) ;
#13989=CARTESIAN_POINT ( 'NONE',  ( 164.5152310637604387, -4.999999999999973355, -1.826485974285146238E-14 ) ) ;
#13990=VECTOR ( 'NONE', #23208, 1000.000000000000000 ) ;
#13991=CARTESIAN_POINT ( 'NONE',  ( 156.1922820468853672, -4.999999999999975131, -10.74328820663507678 ) ) ;
#13992=ORIENTED_EDGE ( 'NONE', *, *, #9375, .T. ) ;
#13993=PLANE ( 'NONE',  #7184 ) ;
#13996=VECTOR ( 'NONE', #28622, 1000.000000000000000 ) ;
#14000=DIRECTION ( 'NONE',  ( -1.110223024625156540E-16, 0.000000000000000000, -1.000000000000000000 ) ) ;
#14001=CARTESIAN_POINT ( 'NONE',  ( 159.5152310637605240, -4.999999999999973355, -19.94844914048349693 ) ) ;
#14004=DIRECTION ( 'NONE',  ( -2.698458740408365879E-16, 1.000000000000000000, 0.000000000000000000 ) ) ;
#14005=DIRECTION ( 'NONE',  ( 0.5877852522924731371, 0.000000000000000000, 0.8090169943749474513 ) ) ;
#14007=AXIS2_PLACEMENT_3D ( 'NONE', #7481, #24117, #23662 ) ;
#14008=CARTESIAN_POINT ( 'NONE',  ( 147.0152310637605240, -10.00000000000000355, 1.702185954127501066 ) ) ;
#14011=ADVANCED_FACE ( 'NONE', ( #723 ), #12459, .T. ) ;
#14012=LINE ( 'NONE', #16015, #17955 ) ;
#14013=VERTEX_POINT ( 'NONE', #7744 ) ;
#14014=DIRECTION ( 'NONE',  ( 0.9510565162951536422, 0.000000000000000000, -0.3090169943749475623 ) ) ;
#14016=VERTEX_POINT ( 'NONE', #12615 ) ;
#14019=ORIENTED_EDGE ( 'NONE', *, *, #23837, .F. ) ;
#14020=DIRECTION ( 'NONE',  ( 1.000000000000000000, 0.000000000000000000, 0.000000000000000000 ) ) ;
#14021=EDGE_CURVE ( 'NONE', #10807, #2818, #5611, .T. ) ;
#14025=ORIENTED_EDGE ( 'NONE', *, *, #27215, .F. ) ;
#14027=ORIENTED_EDGE ( 'NONE', *, *, #11250, .T. ) ;
#14029=LINE ( 'NONE', #4736, #20843 ) ;
#14031=DIRECTION ( 'NONE',  ( 0.5877852522924731371, 1.586114251531760728E-16, 0.8090169943749474513 ) ) ;
#14032=LINE ( 'NONE', #5038, #4278 ) ;
#14033=EDGE_LOOP ( 'NONE', ( #13237, #5707, #5069, #24734, #21479 ) ) ;
#14034=CARTESIAN_POINT ( 'NONE',  ( 176.1922820468853104, -9.999999999999994671, -19.40354224447947828 ) ) ;
#14035=EDGE_LOOP ( 'NONE', ( #28132, #24728, #7432, #21215 ) ) ;
#14037=ORIENTED_EDGE ( 'NONE', *, *, #27058, .F. ) ;
#14041=PLANE ( 'NONE',  #4759 ) ;
#14045=AXIS2_PLACEMENT_3D ( 'NONE', #23485, #2592, #23329 ) ;
#14047=VECTOR ( 'NONE', #19497, 1000.000000000000000 ) ;
#14048=ORIENTED_EDGE ( 'NONE', *, *, #11078, .T. ) ;
#14049=FACE_BOUND ( 'NONE', #1343, .T. ) ;
#14050=VECTOR ( 'NONE', #4281, 1000.000000000000000 ) ;
#14052=CARTESIAN_POINT ( 'NONE',  ( 146.1922820468853956, -1.999999999999977573, -2.083034168790677043 ) ) ;
#14059=EDGE_CURVE ( 'NONE', #1878, #24297, #12164, .T. ) ;
#14062=AXIS2_PLACEMENT_3D ( 'NONE', #7702, #17013, #14704 ) ;
#14063=CARTESIAN_POINT ( 'NONE',  ( 107.8490226364544498, -4.999999999999987566, -78.35690154919700490 ) ) ;
#14064=ORIENTED_EDGE ( 'NONE', *, *, #5894, .T. ) ;
#14071=EDGE_LOOP ( 'NONE', ( #2885, #7398, #19518, #8496 ) ) ;
#14072=CARTESIAN_POINT ( 'NONE',  ( 149.5152310637604955, -1.999999999999976685, -4.391296821672111328 ) ) ;
#14077=DIRECTION ( 'NONE',  ( -0.5877852522924731371, -1.586114251531760728E-16, -0.8090169943749474513 ) ) ;
#14079=ORIENTED_EDGE ( 'NONE', *, *, #30163, .T. ) ;
#14083=VERTEX_POINT ( 'NONE', #8184 ) ;
#14084=ORIENTED_EDGE ( 'NONE', *, *, #7018, .F. ) ;
#14085=CARTESIAN_POINT ( 'NONE',  ( 19.50478146705679450, -5.000000000000012434, -60.02954481736172454 ) ) ;
#14086=VECTOR ( 'NONE', #11322, 1000.000000000000000 ) ;
#14087=CARTESIAN_POINT ( 'NONE',  ( 8.772461160124507273, -5.000000000000015099, 26.99885929302450904 ) ) ;
#14089=PLANE ( 'NONE',  #29104 ) ;
#14090=DIRECTION ( 'NONE',  ( 0.5877852522924731371, 1.586114251531760728E-16, 0.8090169943749474513 ) ) ;
#14091=EDGE_CURVE ( 'NONE', #17985, #4670, #26848, .T. ) ;
#14092=DIRECTION ( 'NONE',  ( -0.8090169943749474513, -2.183098979609982436E-16, -0.5877852522924731371 ) ) ;
#14093=EDGE_CURVE ( 'NONE', #30260, #1558, #13230, .T. ) ;
#14095=ADVANCED_FACE ( 'NONE', ( #3928 ), #13071, .T. ) ;
#14099=EDGE_LOOP ( 'NONE', ( #8567, #5153, #1269, #96 ) ) ;
#14100=DIRECTION ( 'NONE',  ( -1.110223024625156540E-16, 0.000000000000000000, -1.000000000000000000 ) ) ;
#14101=CARTESIAN_POINT ( 'NONE',  ( 158.6922820468853104, -10.00000000000000000, -0.6060766987539614181 ) ) ;
#14102=CARTESIAN_POINT ( 'NONE',  ( 143.6922820468854525, -4.999999999999978684, -17.92658477444275889 ) ) ;
#14103=CARTESIAN_POINT ( 'NONE',  ( 168.6922820468852819, -1.999999999999971356, 2.247092850131519715 ) ) ;
#14106=EDGE_LOOP ( 'NONE', ( #16726, #7906, #19815, #18327 ) ) ;
#14107=CARTESIAN_POINT ( 'NONE',  ( 148.6922820468854241, -10.00000000000000178, -15.07341522555727664 ) ) ;
#14111=DIRECTION ( 'NONE',  ( -0.8090169943749474513, -2.183098979609982436E-16, 0.5877852522924731371 ) ) ;
#14112=CARTESIAN_POINT ( 'NONE',  ( 168.6922820468852819, -9.999999999999998224, -0.6060766987539614181 ) ) ;
#14113=VECTOR ( 'NONE', #2643, 1000.000000000000000 ) ;
#14116=VECTOR ( 'NONE', #10313, 1000.000000000000000 ) ;
#14119=ORIENTED_EDGE ( 'NONE', *, *, #23378, .T. ) ;
#14123=EDGE_LOOP ( 'NONE', ( #20754, #28070, #10328, #26665, #20614 ) ) ;
#14125=ADVANCED_FACE ( 'NONE', ( #10927 ), #6063, .T. ) ;
#14126=VECTOR ( 'NONE', #22049, 1000.000000000000000 ) ;
#14127=VECTOR ( 'NONE', #5074, 1000.000000000000000 ) ;
#14129=DIRECTION ( 'NONE',  ( 0.5877852522924731371, 1.586114251531760728E-16, -0.8090169943749474513 ) ) ;
#14131=LINE ( 'NONE', #14277, #5332 ) ;
#14132=ORIENTED_EDGE ( 'NONE', *, *, #21975, .F. ) ;
#14133=DIRECTION ( 'NONE',  ( 0.3090169943749472292, 8.338696094057992503E-17, -0.9510565162951536422 ) ) ;
#14135=LINE ( 'NONE', #7440, #10725 ) ;
#14138=ORIENTED_EDGE ( 'NONE', *, *, #15715, .T. ) ;
#14139=DIRECTION ( 'NONE',  ( -0.5877852522924731371, 0.000000000000000000, 0.8090169943749474513 ) ) ;
#14140=DIRECTION ( 'NONE',  ( 0.9510565162951536422, 2.566386769018988816E-16, 0.3090169943749472292 ) ) ;
#14142=DIRECTION ( 'NONE',  ( -1.110223024625156540E-16, 0.000000000000000000, -1.000000000000000000 ) ) ;
#14143=DIRECTION ( 'NONE',  ( 1.000000000000000000, 2.698458740408365879E-16, -1.110223024625156540E-16 ) ) ;
#14144=VECTOR ( 'NONE', #8039, 1000.000000000000000 ) ;
#14146=EDGE_LOOP ( 'NONE', ( #19723, #28474, #4612, #14808, #19075 ) ) ;
#14147=VECTOR ( 'NONE', #8786, 999.9999999999998863 ) ;
#14148=LINE ( 'NONE', #13989, #1283 ) ;
#14150=VERTEX_POINT ( 'NONE', #1498 ) ;
#14151=FACE_OUTER_BOUND ( 'NONE', #30180, .T. ) ;
#14152=EDGE_LOOP ( 'NONE', ( #26358, #12857, #22939, #22159 ) ) ;
#14154=VECTOR ( 'NONE', #12939, 1000.000000000000000 ) ;
#14157=CARTESIAN_POINT ( 'NONE',  ( 164.5152310637604387, -1.999999999999972689, -4.391296821672111328 ) ) ;
#14160=EDGE_CURVE ( 'NONE', #27873, #23858, #5918, .T. ) ;
#14163=CARTESIAN_POINT ( 'NONE',  ( 142.0152310637605524, -1.999999999999978684, 1.702185954127501066 ) ) ;
#14164=CARTESIAN_POINT ( 'NONE',  ( 15.45310053882616153, -5.000000000000013323, 47.55975312665928811 ) ) ;
#14165=VECTOR ( 'NONE', #12616, 1000.000000000000000 ) ;
#14167=CARTESIAN_POINT ( 'NONE',  ( 149.7287565553230309, -1.999999999999975353, -33.82050807568879947 ) ) ;
#14173=ORIENTED_EDGE ( 'NONE', *, *, #22566, .F. ) ;
#14174=CARTESIAN_POINT ( 'NONE',  ( 167.2287565553229456, -4.999999999999972466, -20.83012701892220164 ) ) ;
#14177=FACE_BOUND ( 'NONE', #6892, .T. ) ;
#14178=ORIENTED_EDGE ( 'NONE', *, *, #10143, .F. ) ;
#14179=EDGE_LOOP ( 'NONE', ( #5057, #27985, #13745, #4584 ) ) ;
#14181=DIRECTION ( 'NONE',  ( -2.698458740408365879E-16, 1.000000000000000000, 0.000000000000000000 ) ) ;
#14184=LINE ( 'NONE', #27831, #17890 ) ;
#14185=VERTEX_POINT ( 'NONE', #10788 ) ;
#14186=DIRECTION ( 'NONE',  ( -2.698458740408365879E-16, 1.000000000000000000, 0.000000000000000000 ) ) ;
#14189=VECTOR ( 'NONE', #3297, 1000.000000000000000 ) ;
#14190=VERTEX_POINT ( 'NONE', #8036 ) ;
#14192=CIRCLE ( 'NONE', #10301, 3.000000000000002665 ) ;
#14195=ORIENTED_EDGE ( 'NONE', *, *, #25974, .T. ) ;
#14196=ORIENTED_EDGE ( 'NONE', *, *, #5259, .F. ) ;
#14200=EDGE_CURVE ( 'NONE', #13154, #4554, #3690, .T. ) ;
#14203=EDGE_CURVE ( 'NONE', #11438, #22675, #27315, .T. ) ;
#14205=EDGE_CURVE ( 'NONE', #24876, #22090, #22550, .T. ) ;
#14207=FACE_BOUND ( 'NONE', #1189, .T. ) ;
#14208=DIRECTION ( 'NONE',  ( 0.9510565162951536422, 0.000000000000000000, -0.3090169943749475623 ) ) ;
#14209=CARTESIAN_POINT ( 'NONE',  ( 143.6922820468854525, -10.00000000000000355, -32.39392330124607611 ) ) ;
#14214=LINE ( 'NONE', #14063, #3751 ) ;
#14222=DIRECTION ( 'NONE',  ( -0.8090169943749474513, -2.183098979609982436E-16, -0.5877852522924731371 ) ) ;
#14224=VERTEX_POINT ( 'NONE', #24380 ) ;
#14226=CARTESIAN_POINT ( 'NONE',  ( 9.486764522130870958, -5.000000000000015099, 29.19725899082042986 ) ) ;
#14227=CARTESIAN_POINT ( 'NONE',  ( 132.2287565553230309, -4.999999999999982236, -20.83012701892220875 ) ) ;
#14228=VECTOR ( 'NONE', #24393, 1000.000000000000000 ) ;
#14230=ORIENTED_EDGE ( 'NONE', *, *, #29888, .T. ) ;
#14231=LINE ( 'NONE', #21419, #9093 ) ;
#14237=ORIENTED_EDGE ( 'NONE', *, *, #26935, .F. ) ;
#14238=ORIENTED_EDGE ( 'NONE', *, *, #23209, .T. ) ;
#14239=DIRECTION ( 'NONE',  ( -0.9510565162951536422, -2.566386769018988323E-16, 0.3090169943749475623 ) ) ;
#14240=VECTOR ( 'NONE', #3529, 1000.000000000000000 ) ;
#14243=LINE ( 'NONE', #21124, #26770 ) ;
#14244=DIRECTION ( 'NONE',  ( 0.5877852522924731371, 1.586114251531760728E-16, -0.8090169943749474513 ) ) ;
#14245=VECTOR ( 'NONE', #26019, 1000.000000000000000 ) ;
#14250=ORIENTED_EDGE ( 'NONE', *, *, #22240, .T. ) ;
#14253=CARTESIAN_POINT ( 'NONE',  ( 109.5403287000431192, -4.999999999999987566, -79.58570733226751770 ) ) ;
#14254=CARTESIAN_POINT ( 'NONE',  ( 132.0152310637605524, -4.999999999999982236, -1.465663491281971624E-14 ) ) ;
#14256=CARTESIAN_POINT ( 'NONE',  ( 141.1922820468854525, -1.999999999999978462, -19.40354224447947473 ) ) ;
#14258=ORIENTED_EDGE ( 'NONE', *, *, #30196, .F. ) ;
#14259=FACE_OUTER_BOUND ( 'NONE', #27387, .T. ) ;
#14260=CARTESIAN_POINT ( 'NONE',  ( 154.7287565553229456, -4.999999999999976019, -7.839745962155600267 ) ) ;
#14261=EDGE_CURVE ( 'NONE', #17616, #14597, #15506, .T. ) ;
#14263=ORIENTED_EDGE ( 'NONE', *, *, #9572, .F. ) ;
#14265=ORIENTED_EDGE ( 'NONE', *, *, #681, .F. ) ;
#14268=EDGE_CURVE ( 'NONE', #12321, #11833, #6370, .T. ) ;
#14271=VECTOR ( 'NONE', #14129, 1000.000000000000000 ) ;
#14272=EDGE_CURVE ( 'NONE', #16967, #18308, #19630, .T. ) ;
#14273=EDGE_CURVE ( 'NONE', #17474, #23715, #5763, .T. ) ;
#14276=CARTESIAN_POINT ( 'NONE',  ( 143.6922820468853956, -1.999999999999978462, 2.247092850131519715 ) ) ;
#14277=CARTESIAN_POINT ( 'NONE',  ( 152.0152310637604671, -10.00000000000000178, -17.38167787843870826 ) ) ;
#14278=ORIENTED_EDGE ( 'NONE', *, *, #14859, .F. ) ;
#14280=CARTESIAN_POINT ( 'NONE',  ( 149.7287565553229456, -1.999999999999976685, 0.8205080756887930260 ) ) ;
#14284=FACE_OUTER_BOUND ( 'NONE', #8119, .T. ) ;
#14285=CARTESIAN_POINT ( 'NONE',  ( 156.1922820468854241, -1.999999999999974909, -28.06379628232387446 ) ) ;
#14287=DIRECTION ( 'NONE',  ( 1.000000000000000000, 2.698458740408365879E-16, -1.110223024625156540E-16 ) ) ;
#14290=CARTESIAN_POINT ( 'NONE',  ( 21.01610262522592976, -5.000000000000011546, -64.68091306524351580 ) ) ;
#14293=CARTESIAN_POINT ( 'NONE',  ( 164.7287565553228887, -9.999999999999998224, -7.839745962155603820 ) ) ;
#14294=VERTEX_POINT ( 'NONE', #25133 ) ;
#14295=EDGE_LOOP ( 'NONE', ( #8641, #28965, #7722, #1577 ) ) ;
#14296=DIRECTION ( 'NONE',  ( 1.000000000000000000, 2.698458740408365879E-16, 0.000000000000000000 ) ) ;
#14297=ORIENTED_EDGE ( 'NONE', *, *, #817, .F. ) ;
#14302=LINE ( 'NONE', #16610, #6270 ) ;
#14304=CARTESIAN_POINT ( 'NONE',  ( 149.5152310637606092, -10.00000000000000178, -28.60870317832789667 ) ) ;
#14307=VECTOR ( 'NONE', #5330, 1000.000000000000000 ) ;
#14309=LINE ( 'NONE', #5017, #17180 ) ;
#14310=PLANE ( 'NONE',  #27296 ) ;
#14311=DIRECTION ( 'NONE',  ( -0.5877852522924731371, -1.586114251531760728E-16, -0.8090169943749474513 ) ) ;
#14312=CARTESIAN_POINT ( 'NONE',  ( 172.0152310637604387, -4.999999999999970690, -1.909752701132032978E-14 ) ) ;
#14314=DIRECTION ( 'NONE',  ( -2.698458740408365879E-16, 1.000000000000000000, 0.000000000000000000 ) ) ;
#14316=ORIENTED_EDGE ( 'NONE', *, *, #20037, .F. ) ;
#14322=CARTESIAN_POINT ( 'NONE',  ( 175.7287565553229456, -4.999999999999970690, 3.500000000000003109 ) ) ;
#14323=ORIENTED_EDGE ( 'NONE', *, *, #16704, .F. ) ;
#14324=EDGE_CURVE ( 'NONE', #22052, #18123, #4223, .T. ) ;
#14325=EDGE_LOOP ( 'NONE', ( #28357, #15082, #8857, #5206, #14538 ) ) ;
#14328=AXIS2_PLACEMENT_3D ( 'NONE', #29457, #19764, #29289 ) ;
#14330=DIRECTION ( 'NONE',  ( -2.698458740408365879E-16, 1.000000000000000000, 0.000000000000000000 ) ) ;
#14331=ORIENTED_EDGE ( 'NONE', *, *, #16759, .F. ) ;
#14335=ORIENTED_EDGE ( 'NONE', *, *, #13962, .T. ) ;
#14341=ADVANCED_FACE ( 'NONE', ( #27910 ), #6969, .T. ) ;
#14346=ORIENTED_EDGE ( 'NONE', *, *, #7599, .F. ) ;
#14347=FACE_BOUND ( 'NONE', #14635, .T. ) ;
#14348=VECTOR ( 'NONE', #12714, 1000.000000000000000 ) ;
#14349=ORIENTED_EDGE ( 'NONE', *, *, #19614, .F. ) ;
#14350=LINE ( 'NONE', #7804, #11573 ) ;
#14351=LINE ( 'NONE', #14508, #4761 ) ;
#14352=PLANE ( 'NONE',  #3379 ) ;
#14353=CARTESIAN_POINT ( 'NONE',  ( 169.7287565553228603, -1.999999999999971356, 0.8205080756887930260 ) ) ;
#14356=FACE_OUTER_BOUND ( 'NONE', #9603, .T. ) ;
#14357=EDGE_CURVE ( 'NONE', #25113, #6635, #29925, .T. ) ;
#14358=EDGE_CURVE ( 'NONE', #11977, #20122, #20385, .T. ) ;
#14361=ORIENTED_EDGE ( 'NONE', *, *, #18156, .T. ) ;
#14364=VERTEX_POINT ( 'NONE', #2247 ) ;
#14367=DIRECTION ( 'NONE',  ( 0.9510565162951536422, 0.000000000000000000, -0.3090169943749475623 ) ) ;
#14369=PLANE ( 'NONE',  #15423 ) ;
#14371=EDGE_LOOP ( 'NONE', ( #6934, #10000, #27924, #11905 ) ) ;
#14375=LINE ( 'NONE', #23712, #13973 ) ;
#14378=ORIENTED_EDGE ( 'NONE', *, *, #20647, .F. ) ;
#14379=CARTESIAN_POINT ( 'NONE',  ( 172.7287565553229456, -4.999999999999970690, -33.50000000000000000 ) ) ;
#14380=EDGE_LOOP ( 'NONE', ( #25980, #23154, #1716, #11602 ) ) ;
#14385=VECTOR ( 'NONE', #247, 1000.000000000000000 ) ;
#14386=DIRECTION ( 'NONE',  ( -1.110223024625156540E-16, 0.000000000000000000, -1.000000000000000000 ) ) ;
#14387=CARTESIAN_POINT ( 'NONE',  ( 132.0152310637605524, -1.999999999999981348, -26.04193191628310800 ) ) ;
#14388=ADVANCED_FACE ( 'NONE', ( #20990 ), #23289, .T. ) ;
#14390=LINE ( 'NONE', #18993, #13578 ) ;
#14391=AXIS2_PLACEMENT_3D ( 'NONE', #16893, #21475, #26226 ) ;
#14393=AXIS2_PLACEMENT_3D ( 'NONE', #20086, #13060, #15497 ) ;
#14397=EDGE_CURVE ( 'NONE', #18151, #2772, #18101, .T. ) ;
#14399=ORIENTED_EDGE ( 'NONE', *, *, #8792, .F. ) ;
#14400=DIRECTION ( 'NONE',  ( 0.3090169943749472292, 8.338696094057992503E-17, -0.9510565162951536422 ) ) ;
#14402=EDGE_CURVE ( 'NONE', #14895, #2921, #1952, .T. ) ;
#14403=CARTESIAN_POINT ( 'NONE',  ( 132.0152310637605808, -10.00000000000000711, 1.702185954127501066 ) ) ;
#14404=LINE ( 'NONE', #17017, #14385 ) ;
#14405=EDGE_CURVE ( 'NONE', #16007, #18100, #11085, .T. ) ;
#14407=VERTEX_POINT ( 'NONE', #20833 ) ;
#14410=PLANE ( 'NONE',  #11019 ) ;
#14411=LINE ( 'NONE', #23592, #78 ) ;
#14412=VECTOR ( 'NONE', #21027, 1000.000000000000000 ) ;
#14420=VECTOR ( 'NONE', #26742, 1000.000000000000000 ) ;
#14421=ORIENTED_EDGE ( 'NONE', *, *, #14816, .T. ) ;
#14424=CARTESIAN_POINT ( 'NONE',  ( 143.6922820468854525, -10.00000000000000355, -32.39392330124607611 ) ) ;
#14425=DIRECTION ( 'NONE',  ( -0.5877852522924731371, -1.586114251531760728E-16, -0.8090169943749474513 ) ) ;
#14427=DIRECTION ( 'NONE',  ( 0.9510565162951535312, 2.566386769018988816E-16, -0.3090169943749475623 ) ) ;
#14428=VECTOR ( 'NONE', #9685, 1000.000000000000000 ) ;
#14429=ORIENTED_EDGE ( 'NONE', *, *, #19896, .F. ) ;
#14430=DIRECTION ( 'NONE',  ( -0.8090169943749474513, -2.183098979609982436E-16, 0.5877852522924731371 ) ) ;
#14432=VECTOR ( 'NONE', #29581, 1000.000000000000000 ) ;
#14434=ORIENTED_EDGE ( 'NONE', *, *, #28068, .T. ) ;
#14435=EDGE_CURVE ( 'NONE', #10636, #28125, #8931, .T. ) ;
#14436=VECTOR ( 'NONE', #7066, 1000.000000000000000 ) ;
#14437=CARTESIAN_POINT ( 'NONE',  ( 162.0152310637604387, -4.999999999999973355, 1.702185954127501066 ) ) ;
#14438=DIRECTION ( 'NONE',  ( 0.9510565162951535312, 2.566386769018988816E-16, -0.3090169943749475623 ) ) ;
#14439=EDGE_CURVE ( 'NONE', #11101, #3398, #28055, .T. ) ;
#14440=EDGE_CURVE ( 'NONE', #28379, #26554, #29776, .T. ) ;
#14443=EDGE_CURVE ( 'NONE', #1194, #8663, #11378, .T. ) ;
#14448=DIRECTION ( 'NONE',  ( 1.110223024625156540E-16, 2.995891024602366092E-32, 1.000000000000000000 ) ) ;
#14449=ORIENTED_EDGE ( 'NONE', *, *, #5603, .T. ) ;
#14450=PLANE ( 'NONE',  #15946 ) ;
#14455=VECTOR ( 'NONE', #6487, 1000.000000000000000 ) ;
#14456=FACE_OUTER_BOUND ( 'NONE', #19260, .T. ) ;
#14457=CARTESIAN_POINT ( 'NONE',  ( 152.2287565553229740, -1.999999999999975353, -12.16987298107780369 ) ) ;
#14458=DIRECTION ( 'NONE',  ( -0.5877852522924731371, 0.000000000000000000, 0.8090169943749474513 ) ) ;
#14459=CIRCLE ( 'NONE', #18372, 5.999999999999977796 ) ;
#14460=VECTOR ( 'NONE', #8182, 1000.000000000000000 ) ;
#14461=EDGE_LOOP ( 'NONE', ( #28248, #17522, #5497, #29077 ) ) ;
#14462=CARTESIAN_POINT ( 'NONE',  ( 162.0152310637604955, -1.999999999999972244, -26.04193191628311155 ) ) ;
#14463=FACE_OUTER_BOUND ( 'NONE', #28518, .T. ) ;
#14464=VECTOR ( 'NONE', #10576, 1000.000000000000000 ) ;
#14465=ORIENTED_EDGE ( 'NONE', *, *, #27246, .F. ) ;
#14466=LINE ( 'NONE', #7171, #8304 ) ;
#14467=CARTESIAN_POINT ( 'NONE',  ( 157.2287565553229172, -1.999999999999974465, -3.509618943233403510 ) ) ;
#14469=FACE_OUTER_BOUND ( 'NONE', #28613, .T. ) ;
#14471=VERTEX_POINT ( 'NONE', #9078 ) ;
#14473=EDGE_CURVE ( 'NONE', #23755, #2694, #18405, .T. ) ;
#14474=DIRECTION ( 'NONE',  ( -0.5877852522924731371, -1.586114251531760235E-16, 0.8090169943749474513 ) ) ;
#14475=VECTOR ( 'NONE', #3847, 1000.000000000000000 ) ;
#14477=EDGE_CURVE ( 'NONE', #13095, #9877, #25432, .T. ) ;
#14479=CARTESIAN_POINT ( 'NONE',  ( 152.2287565553230309, -4.999999999999976019, -29.49038105676660848 ) ) ;
#14481=ORIENTED_EDGE ( 'NONE', *, *, #28067, .T. ) ;
#14484=CARTESIAN_POINT ( 'NONE',  ( 104.1536536346199426, -4.999999999999989342, -75.67205881269151746 ) ) ;
#14486=DIRECTION ( 'NONE',  ( 0.3090169943749475623, 8.338696094058001131E-17, 0.9510565162951536422 ) ) ;
#14487=ORIENTED_EDGE ( 'NONE', *, *, #234, .F. ) ;
#14489=ORIENTED_EDGE ( 'NONE', *, *, #25176, .F. ) ;
#14491=ORIENTED_EDGE ( 'NONE', *, *, #28246, .F. ) ;
#14496=ORIENTED_EDGE ( 'NONE', *, *, #29567, .F. ) ;
#14497=LINE ( 'NONE', #12213, #3321 ) ;
#14502=VECTOR ( 'NONE', #15547, 1000.000000000000000 ) ;
#14503=CARTESIAN_POINT ( 'NONE',  ( 132.0152310637605808, -10.00000000000000711, -6.958068083716893781 ) ) ;
#14504=ADVANCED_FACE ( 'NONE', ( #9986 ), #14410, .T. ) ;
#14505=DIRECTION ( 'NONE',  ( 0.5877852522924731371, 0.000000000000000000, 0.8090169943749474513 ) ) ;
#14506=VECTOR ( 'NONE', #13603, 1000.000000000000000 ) ;
#14507=CARTESIAN_POINT ( 'NONE',  ( 166.1922820468853388, -4.999999999999973355, -10.74328820663507678 ) ) ;
#14508=CARTESIAN_POINT ( 'NONE',  ( 75.37105117200049165, -4.999999999999997335, 54.76027405692665440 ) ) ;
#14509=CARTESIAN_POINT ( 'NONE',  ( 174.5152310637603819, -1.999999999999970024, -4.391296821672111328 ) ) ;
#14510=LINE ( 'NONE', #9785, #9496 ) ;
#14512=CARTESIAN_POINT ( 'NONE',  ( 141.1922820468854525, -1.999999999999978684, -22.25671179336495697 ) ) ;
#14513=LINE ( 'NONE', #19108, #24710 ) ;
#14514=VERTEX_POINT ( 'NONE', #23591 ) ;
#14516=EDGE_LOOP ( 'NONE', ( #15151, #28608, #3473, #10425, #21044 ) ) ;
#14519=CARTESIAN_POINT ( 'NONE',  ( 161.1922820468853956, -9.999999999999998224, -30.91696583120936026 ) ) ;
#14520=LINE ( 'NONE', #12240, #20800 ) ;
#14521=DIRECTION ( 'NONE',  ( -2.698458740408365879E-16, 1.000000000000000000, 0.000000000000000000 ) ) ;
#14525=ORIENTED_EDGE ( 'NONE', *, *, #14542, .T. ) ;
#14526=AXIS2_PLACEMENT_3D ( 'NONE', #1542, #23044, #15554 ) ;
#14529=CARTESIAN_POINT ( 'NONE',  ( 152.2287565553230024, -1.999999999999974909, -20.83012701892220520 ) ) ;
#14532=ORIENTED_EDGE ( 'NONE', *, *, #8919, .T. ) ;
#14533=AXIS2_PLACEMENT_3D ( 'NONE', #17507, #26861, #8197 ) ;
#14534=DIRECTION ( 'NONE',  ( 1.000000000000000000, 2.891205793294675861E-16, 0.000000000000000000 ) ) ;
#14537=DIRECTION ( 'NONE',  ( -2.698458740408365879E-16, 1.000000000000000000, 0.000000000000000000 ) ) ;
#14538=ORIENTED_EDGE ( 'NONE', *, *, #18943, .T. ) ;
#14539=ORIENTED_EDGE ( 'NONE', *, *, #21862, .F. ) ;
#14541=CARTESIAN_POINT ( 'NONE',  ( 132.2287565553230024, -1.999999999999981348, -29.49038105676660138 ) ) ;
#14542=EDGE_CURVE ( 'NONE', #8702, #14190, #850, .T. ) ;
#14543=DIRECTION ( 'NONE',  ( 0.3090169943749475623, 8.338696094058001131E-17, 0.9510565162951536422 ) ) ;
#14544=DIRECTION ( 'NONE',  ( 1.000000000000000000, 2.698458740408365879E-16, -1.110223024625156540E-16 ) ) ;
#14545=PLANE ( 'NONE',  #26280 ) ;
#14546=DIRECTION ( 'NONE',  ( 3.166185380091481561E-16, -0.7071067811865493491, 0.7071067811865456854 ) ) ;
#14553=DIRECTION ( 'NONE',  ( -2.698458740408366372E-16, 1.000000000000000000, 0.000000000000000000 ) ) ;
#14554=DIRECTION ( 'NONE',  ( -2.698458740408365879E-16, 1.000000000000000000, 0.000000000000000000 ) ) ;
#14559=VERTEX_POINT ( 'NONE', #23911 ) ;
#14563=LINE ( 'NONE', #28970, #4456 ) ;
#14566=ORIENTED_EDGE ( 'NONE', *, *, #442, .T. ) ;
#14571=VECTOR ( 'NONE', #16584, 1000.000000000000000 ) ;
#14573=EDGE_CURVE ( 'NONE', #5728, #19562, #3006, .T. ) ;
#14574=EDGE_CURVE ( 'NONE', #18591, #23239, #19156, .T. ) ;
#14575=EDGE_CURVE ( 'NONE', #11550, #6495, #253, .T. ) ;
#14576=EDGE_LOOP ( 'NONE', ( #14875, #26034, #29638, #16297 ) ) ;
#14577=EDGE_CURVE ( 'NONE', #17358, #15701, #18853, .T. ) ;
#14578=CARTESIAN_POINT ( 'NONE',  ( 95.11637572886448311, -4.999999999999991118, 69.10609207675695131 ) ) ;
#14580=ORIENTED_EDGE ( 'NONE', *, *, #24076, .F. ) ;
#14581=CARTESIAN_POINT ( 'NONE',  ( 130.7287565553229456, -9.999999999999982236, 0.5000000000000052180 ) ) ;
#14582=FACE_OUTER_BOUND ( 'NONE', #14106, .T. ) ;
#14586=DIRECTION ( 'NONE',  ( -0.8090169943749474513, -2.183098979609982436E-16, 0.5877852522924731371 ) ) ;
#14587=LINE ( 'NONE', #16890, #1237 ) ;
#14588=AXIS2_PLACEMENT_3D ( 'NONE', #10835, #20143, #24288 ) ;
#14590=CARTESIAN_POINT ( 'NONE',  ( 168.6922820468853672, -1.999999999999971800, -23.73366926340167282 ) ) ;
#14591=EDGE_LOOP ( 'NONE', ( #3744, #15505, #3731, #3170, #23250, #28482, #3189, #17263 ) ) ;
#14593=ORIENTED_EDGE ( 'NONE', *, *, #11617, .T. ) ;
#14594=CARTESIAN_POINT ( 'NONE',  ( 159.7287565553230024, -9.999999999999998224, -33.82050807568879947 ) ) ;
#14595=CARTESIAN_POINT ( 'NONE',  ( 147.2287565553229740, -10.00000000000000355, -3.509618943233403510 ) ) ;
#14596=ORIENTED_EDGE ( 'NONE', *, *, #4323, .T. ) ;
#14597=VERTEX_POINT ( 'NONE', #17169 ) ;
#14602=DIRECTION ( 'NONE',  ( 0.3090169943749475623, 8.338696094058001131E-17, 0.9510565162951536422 ) ) ;
#14604=DIRECTION ( 'NONE',  ( -0.8090169943749474513, -2.183098979609982436E-16, -0.5877852522924731371 ) ) ;
#14605=VECTOR ( 'NONE', #20091, 1000.000000000000000 ) ;
#14607=AXIS2_PLACEMENT_3D ( 'NONE', #27888, #4946, #4794 ) ;
#14609=ADVANCED_FACE ( 'NONE', ( #19010 ), #21747, .T. ) ;
#14610=ORIENTED_EDGE ( 'NONE', *, *, #4327, .T. ) ;
#14611=AXIS2_PLACEMENT_3D ( 'NONE', #16432, #12299, #21617 ) ;
#14612=CARTESIAN_POINT ( 'NONE',  ( 15.92573302067464702, -5.000000000000013323, -49.01436633517871400 ) ) ;
#14613=LINE ( 'NONE', #739, #23537 ) ;
#14615=DIRECTION ( 'NONE',  ( -0.8090169943749474513, -2.183098979609982436E-16, -0.5877852522924731371 ) ) ;
#14616=CARTESIAN_POINT ( 'NONE',  ( 172.0152310637604387, -1.999999999999970468, -6.958068083716895558 ) ) ;
#14619=LINE ( 'NONE', #19927, #30229 ) ;
#14620=CARTESIAN_POINT ( 'NONE',  ( 151.1922820468853672, -10.00000000000000178, -4.936203717676158398 ) ) ;
#14622=VECTOR ( 'NONE', #16521, 1000.000000000000000 ) ;
#14628=ORIENTED_EDGE ( 'NONE', *, *, #7022, .F. ) ;
#14634=CARTESIAN_POINT ( 'NONE',  ( 97.60856866274521337, -4.999999999999991118, -70.91677623121574925 ) ) ;
#14635=EDGE_LOOP ( 'NONE', ( #3124, #20787, #9356, #8743, #11941 ) ) ;
#14636=PLANE ( 'NONE',  #2320 ) ;
#14637=VERTEX_POINT ( 'NONE', #7422 ) ;
#14639=ORIENTED_EDGE ( 'NONE', *, *, #11755, .F. ) ;
#14645=DIRECTION ( 'NONE',  ( 0.5877852522924731371, 1.586114251531760728E-16, -0.8090169943749474513 ) ) ;
#14648=AXIS2_PLACEMENT_3D ( 'NONE', #6371, #15507, #15351 ) ;
#14650=ADVANCED_FACE ( 'NONE', ( #7713 ), #16569, .T. ) ;
#14651=EDGE_CURVE ( 'NONE', #4252, #7125, #14714, .T. ) ;
#14652=EDGE_CURVE ( 'NONE', #17128, #29523, #559, .T. ) ;
#14653=CARTESIAN_POINT ( 'NONE',  ( 133.6922820468854241, -4.999999999999981348, -15.07341522555727309 ) ) ;
#14654=ADVANCED_FACE ( 'NONE', ( #14259 ), #24056, .T. ) ;
#14655=DIRECTION ( 'NONE',  ( -0.8090169943749474513, -2.183098979609982436E-16, -0.5877852522924731371 ) ) ;
#14656=FACE_OUTER_BOUND ( 'NONE', #14295, .T. ) ;
#14657=LINE ( 'NONE', #24004, #26240 ) ;
#14658=DIRECTION ( 'NONE',  ( -2.698458740408365879E-16, 1.000000000000000000, 0.000000000000000000 ) ) ;
#14659=CARTESIAN_POINT ( 'NONE',  ( 175.7287565553229456, -9.999999999999994671, -10.89389676854971967 ) ) ;
#14661=PLANE ( 'NONE',  #22642 ) ;
#14662=VECTOR ( 'NONE', #26682, 1000.000000000000000 ) ;
#14664=ORIENTED_EDGE ( 'NONE', *, *, #20404, .T. ) ;
#14665=AXIS2_PLACEMENT_3D ( 'NONE', #24645, #29890, #24804 ) ;
#14667=ORIENTED_EDGE ( 'NONE', *, *, #30029, .T. ) ;
#14670=DIRECTION ( 'NONE',  ( -0.5877852522924731371, -1.586114251531760728E-16, -0.8090169943749474513 ) ) ;
#14671=FACE_OUTER_BOUND ( 'NONE', #26317, .T. ) ;
#14675=ADVANCED_FACE ( 'NONE', ( #2555 ), #5275, .T. ) ;
#14681=PLANE ( 'NONE',  #10112 ) ;
#14683=ORIENTED_EDGE ( 'NONE', *, *, #25396, .T. ) ;
#14684=CARTESIAN_POINT ( 'NONE',  ( 172.7287565553229456, -3.999999999999989786, -33.50000000000000000 ) ) ;
#14688=DIRECTION ( 'NONE',  ( -2.698458740408365879E-16, 1.000000000000000000, 0.000000000000000000 ) ) ;
#14690=ORIENTED_EDGE ( 'NONE', *, *, #19238, .T. ) ;
#14691=EDGE_CURVE ( 'NONE', #10866, #3794, #1013, .T. ) ;
#14692=ORIENTED_EDGE ( 'NONE', *, *, #24186, .F. ) ;
#14693=CARTESIAN_POINT ( 'NONE',  ( 142.0152310637605240, -4.999999999999979572, -0.06116980274991495881 ) ) ;
#14695=DIRECTION ( 'NONE',  ( 0.9510565162951535312, 2.566386769018988816E-16, -0.3090169943749475623 ) ) ;
#14696=CYLINDRICAL_SURFACE ( 'NONE', #17473, 8.000000000000007105 ) ;
#14702=VERTEX_POINT ( 'NONE', #5884 ) ;
#14704=DIRECTION ( 'NONE',  ( -0.5877852522924731371, 0.000000000000000000, 0.8090169943749474513 ) ) ;
#14705=LINE ( 'NONE', #5873, #13604 ) ;
#14708=LINE ( 'NONE', #10284, #3496 ) ;
#14709=CARTESIAN_POINT ( 'NONE',  ( 163.6922820468853388, -9.999999999999998224, -17.92658477444275889 ) ) ;
#14711=CARTESIAN_POINT ( 'NONE',  ( 110.6334351267569502, -4.999999999999987566, 80.37989563891109412 ) ) ;
#14713=ADVANCED_FACE ( 'NONE', ( #13039 ), #8005, .T. ) ;
#14714=LINE ( 'NONE', #26197, #28128 ) ;
#14715=CARTESIAN_POINT ( 'NONE',  ( 136.1922820468854241, -1.999999999999980460, -30.91696583120935671 ) ) ;
#14723=EDGE_LOOP ( 'NONE', ( #5396, #6991, #6815, #17291, #29903, #25657 ) ) ;
#14724=VECTOR ( 'NONE', #21950, 1000.000000000000000 ) ;
#14725=LINE ( 'NONE', #24067, #23054 ) ;
#14726=DIRECTION ( 'NONE',  ( -0.5877852522924731371, -1.586114251531760235E-16, 0.8090169943749474513 ) ) ;
#14728=DIRECTION ( 'NONE',  ( -2.698458740408365879E-16, 1.000000000000000000, 0.000000000000000000 ) ) ;
#14730=DIRECTION ( 'NONE',  ( 0.5877852522924731371, 1.586114251531760728E-16, 0.8090169943749474513 ) ) ;
#14733=VECTOR ( 'NONE', #19350, 1000.000000000000000 ) ;
#14734=DIRECTION ( 'NONE',  ( -2.908569913943826047E-16, 1.000000000000000000, 6.826925868028084813E-18 ) ) ;
#14737=DIRECTION ( 'NONE',  ( 0.9510565162951536422, 0.000000000000000000, -0.3090169943749475623 ) ) ;
#14738=EDGE_LOOP ( 'NONE', ( #16585, #21418, #20698, #15448 ) ) ;
#14739=PLANE ( 'NONE',  #23680 ) ;
#14740=EDGE_CURVE ( 'NONE', #22282, #11673, #13191, .T. ) ;
#14741=ADVANCED_FACE ( 'NONE', ( #15164 ), #24500, .T. ) ;
#14742=ORIENTED_EDGE ( 'NONE', *, *, #16372, .T. ) ;
#14745=ADVANCED_FACE ( 'NONE', ( #29583 ), #10891, .T. ) ;
#14747=AXIS2_PLACEMENT_3D ( 'NONE', #14424, #28527, #7577 ) ;
#14749=EDGE_CURVE ( 'NONE', #4536, #18131, #24803, .T. ) ;
#14750=ORIENTED_EDGE ( 'NONE', *, *, #9235, .T. ) ;
#14755=CARTESIAN_POINT ( 'NONE',  ( 162.0152310637604671, -4.999999999999974243, -6.958068083716895558 ) ) ;
#14756=DIRECTION ( 'NONE',  ( 0.9510565162951536422, 0.000000000000000000, -0.3090169943749475623 ) ) ;
#14757=PLANE ( 'NONE',  #12295 ) ;
#14758=CARTESIAN_POINT ( 'NONE',  ( 154.5152310637604955, -10.00000000000000000, -13.05155085951651195 ) ) ;
#14759=PLANE ( 'NONE',  #21604 ) ;
#14760=FACE_OUTER_BOUND ( 'NONE', #3417, .T. ) ;
#14761=PLANE ( 'NONE',  #7360 ) ;
#14762=DIRECTION ( 'NONE',  ( 0.5877852522924731371, 1.586114251531760728E-16, 0.8090169943749474513 ) ) ;
#14766=ORIENTED_EDGE ( 'NONE', *, *, #4909, .F. ) ;
#14770=FACE_BOUND ( 'NONE', #10886, .T. ) ;
#14771=ORIENTED_EDGE ( 'NONE', *, *, #5974, .T. ) ;
#14772=EDGE_CURVE ( 'NONE', #23292, #21455, #29270, .T. ) ;
#14773=ORIENTED_EDGE ( 'NONE', *, *, #4063, .T. ) ;
#14775=CARTESIAN_POINT ( 'NONE',  ( 132.0152310637605808, -10.00000000000000711, -24.27857615940569147 ) ) ;
#14779=DIRECTION ( 'NONE',  ( 0.3090169943749472292, 8.338696094057992503E-17, -0.9510565162951536422 ) ) ;
#14781=EDGE_LOOP ( 'NONE', ( #3808, #29382, #6375, #19189 ) ) ;
#14782=DIRECTION ( 'NONE',  ( -0.8090169943749474513, -2.183098979609982436E-16, 0.5877852522924731371 ) ) ;
#14783=EDGE_LOOP ( 'NONE', ( #2399, #25641, #10454, #24943, #23616 ) ) ;
#14785=ORIENTED_EDGE ( 'NONE', *, *, #13693, .F. ) ;
#14789=DIRECTION ( 'NONE',  ( -2.698458740408365879E-16, 1.000000000000000000, 0.000000000000000000 ) ) ;
#14790=VECTOR ( 'NONE', #2303, 1000.000000000000114 ) ;
#14791=VERTEX_POINT ( 'NONE', #1163 ) ;
#14794=VERTEX_POINT ( 'NONE', #24351 ) ;
#14797=VERTEX_POINT ( 'NONE', #1313 ) ;
#14798=VERTEX_POINT ( 'NONE', #29439 ) ;
#14799=FACE_BOUND ( 'NONE', #11913, .T. ) ;
#14801=CARTESIAN_POINT ( 'NONE',  ( 146.1922820468854241, -4.999999999999978684, -10.74328820663507678 ) ) ;
#14803=LINE ( 'NONE', #16808, #749 ) ;
#14804=AXIS2_PLACEMENT_3D ( 'NONE', #22981, #235, #16090 ) ;
#14807=DIRECTION ( 'NONE',  ( -2.698458740408365879E-16, 1.000000000000000000, 0.000000000000000000 ) ) ;
#14808=ORIENTED_EDGE ( 'NONE', *, *, #4059, .T. ) ;
#14811=EDGE_CURVE ( 'NONE', #7033, #17358, #8462, .T. ) ;
#14813=DIRECTION ( 'NONE',  ( 0.5877852522924731371, 1.586114251531760728E-16, 0.8090169943749474513 ) ) ;
#14814=DIRECTION ( 'NONE',  ( -2.698458740408365879E-16, 1.000000000000000000, 0.000000000000000000 ) ) ;
#14815=ADVANCED_FACE ( 'NONE', ( #13197 ), #3595, .T. ) ;
#14816=EDGE_CURVE ( 'NONE', #14597, #25113, #8312, .T. ) ;
#14820=ORIENTED_EDGE ( 'NONE', *, *, #16054, .T. ) ;
#14821=LINE ( 'NONE', #965, #29624 ) ;
#14822=EDGE_CURVE ( 'NONE', #26115, #24045, #21749, .T. ) ;
#14823=ORIENTED_EDGE ( 'NONE', *, *, #11814, .F. ) ;
#14827=ORIENTED_EDGE ( 'NONE', *, *, #13891, .T. ) ;
#14828=FACE_OUTER_BOUND ( 'NONE', #20774, .T. ) ;
#14830=ORIENTED_EDGE ( 'NONE', *, *, #13069, .F. ) ;
#14835=ORIENTED_EDGE ( 'NONE', *, *, #12144, .F. ) ;
#14836=VERTEX_POINT ( 'NONE', #10757 ) ;
#14837=DIRECTION ( 'NONE',  ( -0.8090169943749474513, -2.183098979609982436E-16, -0.5877852522924731371 ) ) ;
#14842=PLANE ( 'NONE',  #25098 ) ;
#14847=DIRECTION ( 'NONE',  ( -0.9510565162951536422, 0.000000000000000000, -0.3090169943749472292 ) ) ;
#14848=LINE ( 'NONE', #1147, #25785 ) ;
#14849=DIRECTION ( 'NONE',  ( -2.698458740408365879E-16, 1.000000000000000000, 0.000000000000000000 ) ) ;
#14852=VECTOR ( 'NONE', #20742, 1000.000000000000000 ) ;
#14853=DIRECTION ( 'NONE',  ( -1.000000000000000000, -2.698458740408365879E-16, 1.779203565104417375E-16 ) ) ;
#14854=DIRECTION ( 'NONE',  ( 0.9510565162951536422, 2.566386769018988816E-16, 0.3090169943749472292 ) ) ;
#14855=EDGE_CURVE ( 'NONE', #3793, #7383, #4045, .T. ) ;
#14857=VERTEX_POINT ( 'NONE', #3745 ) ;
#14859=EDGE_CURVE ( 'NONE', #6140, #10971, #22363, .T. ) ;
#14861=ORIENTED_EDGE ( 'NONE', *, *, #86, .F. ) ;
#14863=CARTESIAN_POINT ( 'NONE',  ( 7.975443363961738363, -5.000000000000015987, 24.54589074293864925 ) ) ;
#14866=VERTEX_POINT ( 'NONE', #19605 ) ;
#14868=VECTOR ( 'NONE', #23469, 1000.000000000000000 ) ;
#14873=CARTESIAN_POINT ( 'NONE',  ( 144.5152310637606092, -10.00000000000000178, -28.60870317832789311 ) ) ;
#14875=ORIENTED_EDGE ( 'NONE', *, *, #6785, .F. ) ;
#14876=LINE ( 'NONE', #21916, #9131 ) ;
#14877=CARTESIAN_POINT ( 'NONE',  ( 172.0152310637605240, -9.999999999999994671, -32.93883019725009120 ) ) ;
#14879=VECTOR ( 'NONE', #24680, 1000.000000000000000 ) ;
#14885=FACE_OUTER_BOUND ( 'NONE', #7301, .T. ) ;
#14887=DIRECTION ( 'NONE',  ( -2.698458740408365879E-16, 1.000000000000000000, 0.000000000000000000 ) ) ;
#14889=VECTOR ( 'NONE', #23908, 1000.000000000000000 ) ;
#14890=CARTESIAN_POINT ( 'NONE',  ( 152.0152310637604671, -4.999999999999976907, -1.687708096207001986E-14 ) ) ;
#14892=ORIENTED_EDGE ( 'NONE', *, *, #11109, .F. ) ;
#14894=CARTESIAN_POINT ( 'NONE',  ( 166.1922820468853672, -1.999999999999972689, -19.40354224447947473 ) ) ;
#14895=VERTEX_POINT ( 'NONE', #27286 ) ;
#14896=ORIENTED_EDGE ( 'NONE', *, *, #5897, .T. ) ;
#14901=CARTESIAN_POINT ( 'NONE',  ( 168.6922820468853672, -1.999999999999970468, -23.73366926340167637 ) ) ;
#14902=DIRECTION ( 'NONE',  ( 1.110223024625156540E-16, 2.995891024602366092E-32, 1.000000000000000000 ) ) ;
#14903=LINE ( 'NONE', #17356, #1127 ) ;
#14904=VECTOR ( 'NONE', #17907, 1000.000000000000000 ) ;
#14905=VERTEX_POINT ( 'NONE', #6336 ) ;
#14906=CARTESIAN_POINT ( 'NONE',  ( 130.7287565553229456, -10.00000000000000888, -4.785595155761466657 ) ) ;
#14907=EDGE_CURVE ( 'NONE', #4252, #12812, #15632, .T. ) ;
#14909=EDGE_CURVE ( 'NONE', #20491, #22518, #5738, .T. ) ;
#14911=VECTOR ( 'NONE', #2207, 1000.000000000000000 ) ;
#14913=CARTESIAN_POINT ( 'NONE',  ( 108.2065456726138848, -4.999999999999987566, 78.61665723970844510 ) ) ;
#14915=DIRECTION ( 'NONE',  ( -2.698458740408365879E-16, 1.000000000000000000, 0.000000000000000000 ) ) ;
#14918=EDGE_LOOP ( 'NONE', ( #20268, #28719, #16782, #27836 ) ) ;
#14923=FACE_BOUND ( 'NONE', #17165, .T. ) ;
#14924=ORIENTED_EDGE ( 'NONE', *, *, #6229, .T. ) ;
#14928=CARTESIAN_POINT ( 'NONE',  ( 19.98223898111942276, -5.000000000000012434, -61.49900794809289550 ) ) ;
#14929=ORIENTED_EDGE ( 'NONE', *, *, #16143, .T. ) ;
#14933=ORIENTED_EDGE ( 'NONE', *, *, #22628, .T. ) ;
#14934=CARTESIAN_POINT ( 'NONE',  ( 164.7287565553229456, -9.999999999999998224, -25.16025403784440329 ) ) ;
#14935=EDGE_LOOP ( 'NONE', ( #2076, #4036, #22124, #3523 ) ) ;
#14938=VECTOR ( 'NONE', #18742, 1000.000000000000000 ) ;
#14941=LINE ( 'NONE', #24276, #20348 ) ;
#14944=PRODUCT_CONTEXT ( 'NONE', #12001, 'mechanical' ) ;
#14947=DIRECTION ( 'NONE',  ( -2.698458740408365879E-16, 1.000000000000000000, 0.000000000000000000 ) ) ;
#14948=CARTESIAN_POINT ( 'NONE',  ( 133.6922820468854241, -4.999999999999982236, -6.413161187712875133 ) ) ;
#14949=EDGE_CURVE ( 'NONE', #28404, #11106, #26816, .T. ) ;
#14950=EDGE_CURVE ( 'NONE', #20965, #7377, #15172, .T. ) ;
#14951=VECTOR ( 'NONE', #15119, 1000.000000000000000 ) ;
#14952=EDGE_CURVE ( 'NONE', #23002, #1908, #18369, .T. ) ;
#14953=CARTESIAN_POINT ( 'NONE',  ( 149.7287565553230309, -10.00000000000000178, -25.16025403784440329 ) ) ;
#14954=DIRECTION ( 'NONE',  ( -2.698458740408365879E-16, 1.000000000000000000, 0.000000000000000000 ) ) ;
#14956=VECTOR ( 'NONE', #2285, 1000.000000000000000 ) ;
#14957=ORIENTED_EDGE ( 'NONE', *, *, #23837, .T. ) ;
#14961=DIRECTION ( 'NONE',  ( -0.9510565162951536422, -2.566386769018988323E-16, 0.3090169943749475623 ) ) ;
#14964=VERTEX_POINT ( 'NONE', #13640 ) ;
#14967=LINE ( 'NONE', #22307, #5725 ) ;
#14968=CARTESIAN_POINT ( 'NONE',  ( 172.7287565553229456, -1.999999999999970468, 0.5000000000000029976 ) ) ;
#14969=DIRECTION ( 'NONE',  ( 0.9510565162951536422, 2.566386769018988816E-16, 0.3090169943749472292 ) ) ;
#14970=VERTEX_POINT ( 'NONE', #11489 ) ;
#14974=EDGE_LOOP ( 'NONE', ( #17939, #5762, #28895, #19400 ) ) ;
#14983=VECTOR ( 'NONE', #19831, 1000.000000000000000 ) ;
#14985=ORIENTED_EDGE ( 'NONE', *, *, #29649, .T. ) ;
#14987=CARTESIAN_POINT ( 'NONE',  ( 161.1922820468853672, -4.999999999999973355, -19.40354224447947828 ) ) ;
#14988=EDGE_CURVE ( 'NONE', #15011, #6983, #25545, .T. ) ;
#14989=ADVANCED_FACE ( 'NONE', ( #13785 ), #70, .T. ) ;
#14991=DIRECTION ( 'NONE',  ( -0.5877852522924731371, 0.000000000000000000, 0.8090169943749474513 ) ) ;
#14992=ADVANCED_FACE ( 'NONE', ( #2372 ), #20654, .T. ) ;
#14993=CARTESIAN_POINT ( 'NONE',  ( 162.0152310637604955, -1.999999999999972689, -15.61832212156129707 ) ) ;
#14994=LINE ( 'NONE', #24329, #15045 ) ;
#14995=CARTESIAN_POINT ( 'NONE',  ( 172.7287565553229456, -3.999999999999989786, 8.500000000000003553 ) ) ;
#14996=VECTOR ( 'NONE', #2228, 999.9999999999998863 ) ;
#14997=VERTEX_POINT ( 'NONE', #11645 ) ;
#15001=ORIENTED_EDGE ( 'NONE', *, *, #20326, .F. ) ;
#15004=CARTESIAN_POINT ( 'NONE',  ( 167.0152310637605240, -9.999999999999996447, -34.70218595412750773 ) ) ;
#15005=DIRECTION ( 'NONE',  ( 0.3090169943749472292, 8.338696094057992503E-17, -0.9510565162951536422 ) ) ;
#15007=CARTESIAN_POINT ( 'NONE',  ( 143.6922820468854241, -10.00000000000000355, -6.413161187712876909 ) ) ;
#15010=VERTEX_POINT ( 'NONE', #23409 ) ;
#15011=VERTEX_POINT ( 'NONE', #13490 ) ;
#15015=CARTESIAN_POINT ( 'NONE',  ( 134.7287565553230024, -10.00000000000000711, 0.8205080756887930260 ) ) ;
#15016=CARTESIAN_POINT ( 'NONE',  ( 130.7287565553229456, -4.999999999999983125, 3.500000000000003109 ) ) ;
#15027=ADVANCED_FACE ( 'NONE', ( #4192 ), #25403, .T. ) ;
#15028=EDGE_CURVE ( 'NONE', #19562, #1114, #22817, .T. ) ;
#15029=LINE ( 'NONE', #26827, #22594 ) ;
#15030=EDGE_CURVE ( 'NONE', #17600, #28689, #6788, .T. ) ;
#15031=AXIS2_PLACEMENT_3D ( 'NONE', #9061, #15942, #29761 ) ;
#15032=ORIENTED_EDGE ( 'NONE', *, *, #24524, .T. ) ;
#15034=DIRECTION ( 'NONE',  ( 0.7071067811865460184, -0.7071067811865490160, -5.772398745160920240E-16 ) ) ;
#15035=LINE ( 'NONE', #21616, #1691 ) ;
#15039=FACE_OUTER_BOUND ( 'NONE', #1448, .T. ) ;
#15040=DIRECTION ( 'NONE',  ( -2.698458740408365879E-16, 1.000000000000000000, 0.000000000000000000 ) ) ;
#15042=DIRECTION ( 'NONE',  ( -0.9510565162951536422, -2.566386769018988323E-16, 0.3090169943749475623 ) ) ;
#15043=DIRECTION ( 'NONE',  ( 0.9510565162951535312, 2.566386769018988816E-16, -0.3090169943749475623 ) ) ;
#15044=ORIENTED_EDGE ( 'NONE', *, *, #1553, .F. ) ;
#15045=VECTOR ( 'NONE', #3422, 1000.000000000000000 ) ;
#15047=CARTESIAN_POINT ( 'NONE',  ( 166.1922820468853672, -9.999999999999998224, -19.40354224447947828 ) ) ;
#15048=PLANE ( 'NONE',  #7352 ) ;
#15050=VECTOR ( 'NONE', #8144, 1000.000000000000000 ) ;
#15051=VERTEX_POINT ( 'NONE', #23112 ) ;
#15055=DIRECTION ( 'NONE',  ( 0.9510565162951535312, 2.566386769018988816E-16, -0.3090169943749475623 ) ) ;
#15056=CARTESIAN_POINT ( 'NONE',  ( 163.6922820468853104, -1.999999999999973133, -9.266330736598359152 ) ) ;
#15057=PLANE ( 'NONE',  #20106 ) ;
#15058=ORIENTED_EDGE ( 'NONE', *, *, #4572, .F. ) ;
#15059=DIRECTION ( 'NONE',  ( -0.9510565162951536422, -2.566386769018988816E-16, -0.3090169943749472292 ) ) ;
#15061=VECTOR ( 'NONE', #4730, 1000.000000000000000 ) ;
#15065=DIRECTION ( 'NONE',  ( -0.5877852522924731371, 0.000000000000000000, 0.8090169943749474513 ) ) ;
#15066=DIRECTION ( 'NONE',  ( -2.698458740408365879E-16, 1.000000000000000000, 0.000000000000000000 ) ) ;
#15067=VECTOR ( 'NONE', #2264, 1000.000000000000000 ) ;
#15070=ORIENTED_EDGE ( 'NONE', *, *, #26191, .T. ) ;
#15074=FACE_BOUND ( 'NONE', #19968, .T. ) ;
#15075=ORIENTED_EDGE ( 'NONE', *, *, #16998, .T. ) ;
#15076=ORIENTED_EDGE ( 'NONE', *, *, #12756, .T. ) ;
#15077=CARTESIAN_POINT ( 'NONE',  ( 99.54732812125345731, -4.999999999999990230, 72.32536742939463181 ) ) ;
#15079=CARTESIAN_POINT ( 'NONE',  ( 138.6922820468854241, -1.999999999999980016, -32.39392330124607611 ) ) ;
#15080=ORIENTED_EDGE ( 'NONE', *, *, #647, .F. ) ;
#15081=DIRECTION ( 'NONE',  ( -2.698458740408365879E-16, 1.000000000000000000, 0.000000000000000000 ) ) ;
#15082=ORIENTED_EDGE ( 'NONE', *, *, #19893, .T. ) ;
#15085=EDGE_CURVE ( 'NONE', #8261, #7790, #11200, .T. ) ;
#15086=ORIENTED_EDGE ( 'NONE', *, *, #10100, .T. ) ;
#15088=VECTOR ( 'NONE', #15042, 999.9999999999998863 ) ;
#15092=CARTESIAN_POINT ( 'NONE',  ( 164.5152310637604671, -4.999999999999973355, -11.28819510263909542 ) ) ;
#15094=VECTOR ( 'NONE', #23463, 1000.000000000000000 ) ;
#15095=VECTOR ( 'NONE', #6645, 1000.000000000000000 ) ;
#15098=EDGE_LOOP ( 'NONE', ( #3832, #25447, #16541, #9481 ) ) ;
#15102=FACE_BOUND ( 'NONE', #30231, .T. ) ;
#15105=DIRECTION ( 'NONE',  ( -2.698458740408365879E-16, 1.000000000000000000, 0.000000000000000000 ) ) ;
#15108=CARTESIAN_POINT ( 'NONE',  ( 129.5152310637605808, -10.00000000000000888, -28.60870317832789311 ) ) ;
#15109=ORIENTED_EDGE ( 'NONE', *, *, #1975, .F. ) ;
#15112=CARTESIAN_POINT ( 'NONE',  ( 157.0152310637604955, -10.00000000000000000, -6.958068083716895558 ) ) ;
#15113=ORIENTED_EDGE ( 'NONE', *, *, #15375, .F. ) ;
#15114=FACE_OUTER_BOUND ( 'NONE', #21522, .T. ) ;
#15119=DIRECTION ( 'NONE',  ( 0.5877852522924731371, 1.586114251531760728E-16, -0.8090169943749474513 ) ) ;
#15120=EDGE_LOOP ( 'NONE', ( #20808, #2956, #22147, #16435 ) ) ;
#15121=DIRECTION ( 'NONE',  ( -0.9510565162951536422, 0.000000000000000000, -0.3090169943749472292 ) ) ;
#15122=ORIENTED_EDGE ( 'NONE', *, *, #23050, .T. ) ;
#15124=VECTOR ( 'NONE', #29312, 1000.000000000000000 ) ;
#15125=EDGE_CURVE ( 'NONE', #5854, #27422, #18527, .T. ) ;
#15126=ADVANCED_FACE ( 'NONE', ( #29746 ), #27882, .T. ) ;
#15136=MECHANICAL_DESIGN_GEOMETRIC_PRESENTATION_REPRESENTATION('',(#21489),#29347);
#15141=CARTESIAN_POINT ( 'NONE',  ( 164.7287565553229740, -4.999999999999973355, -25.16025403784441394 ) ) ;
#15142=FACE_OUTER_BOUND ( 'NONE', #3775, .T. ) ;
#15144=CARTESIAN_POINT ( 'NONE',  ( 180.7287565553229456, -3.999999999999995559, -33.50000000000000000 ) ) ;
#15145=CARTESIAN_POINT ( 'NONE',  ( 172.7287565553229456, -3.999999999999989786, -41.50000000000000711 ) ) ;
#15146=AXIS2_PLACEMENT_3D ( 'NONE', #22056, #5580, #10292 ) ;
#15147=LINE ( 'NONE', #22036, #8505 ) ;
#15151=ORIENTED_EDGE ( 'NONE', *, *, #27551, .T. ) ;
#15152=DIRECTION ( 'NONE',  ( 0.5877852522924731371, 1.586114251531760728E-16, -0.8090169943749474513 ) ) ;
#15153=LINE ( 'NONE', #17302, #27293 ) ;
#15155=DIRECTION ( 'NONE',  ( -1.110223024625156540E-16, 0.000000000000000000, -1.000000000000000000 ) ) ;
#15156=LINE ( 'NONE', #20495, #518 ) ;
#15157=PLANE ( 'NONE',  #36 ) ;
#15159=ORIENTED_EDGE ( 'NONE', *, *, #7980, .T. ) ;
#15161=CARTESIAN_POINT ( 'NONE',  ( 143.6922820468854525, -10.00000000000000355, -23.73366926340167282 ) ) ;
#15163=EDGE_CURVE ( 'NONE', #16411, #8141, #7393, .T. ) ;
#15164=FACE_OUTER_BOUND ( 'NONE', #8, .T. ) ;
#15165=PLANE ( 'NONE',  #15146 ) ;
#15166=EDGE_CURVE ( 'NONE', #13813, #14224, #527, .T. ) ;
#15168=CARTESIAN_POINT ( 'NONE',  ( 169.5152310637604387, -9.999999999999996447, -2.627941064794695691 ) ) ;
#15169=ADVANCED_FACE ( 'NONE', ( #16537 ), #668, .T. ) ;
#15171=ORIENTED_EDGE ( 'NONE', *, *, #16448, .T. ) ;
#15172=LINE ( 'NONE', #25257, #18364 ) ;
#15174=VECTOR ( 'NONE', #7704, 1000.000000000000000 ) ;
#15176=ORIENTED_EDGE ( 'NONE', *, *, #6530, .F. ) ;
#15177=DIRECTION ( 'NONE',  ( -0.9510565162951536422, -2.566386769018988816E-16, -0.3090169943749472292 ) ) ;
#15179=PLANE ( 'NONE',  #21611 ) ;
#15180=ORIENTED_EDGE ( 'NONE', *, *, #13347, .F. ) ;
#15181=VERTEX_POINT ( 'NONE', #814 ) ;
#15184=LINE ( 'NONE', #27299, #9957 ) ;
#15190=CARTESIAN_POINT ( 'NONE',  ( 132.0152310637605808, -4.999999999999982236, -32.93883019725009120 ) ) ;
#15192=CARTESIAN_POINT ( 'NONE',  ( 22.52742378339506502, -5.000000000000011546, -69.33228131312529285 ) ) ;
#15195=CARTESIAN_POINT ( 'NONE',  ( 175.7287565553229456, -9.999999999999994671, -19.55415080639412650 ) ) ;
#15197=CARTESIAN_POINT ( 'NONE',  ( 142.0152310637605808, -10.00000000000000355, -26.04193191628310800 ) ) ;
#15198=ORIENTED_EDGE ( 'NONE', *, *, #7872, .T. ) ;
#15200=CARTESIAN_POINT ( 'NONE',  ( 156.1922820468853672, -1.999999999999974909, -10.74328820663507678 ) ) ;
#15201=EDGE_CURVE ( 'NONE', #29523, #24484, #12253, .T. ) ;
#15202=EDGE_CURVE ( 'NONE', #6861, #25565, #14231, .T. ) ;
#15203=LINE ( 'NONE', #3187, #19507 ) ;
#15204=ORIENTED_EDGE ( 'NONE', *, *, #15932, .F. ) ;
#15205=ORIENTED_EDGE ( 'NONE', *, *, #19721, .T. ) ;
#15207=ORIENTED_EDGE ( 'NONE', *, *, #8413, .T. ) ;
#15212=CARTESIAN_POINT ( 'NONE',  ( 139.5152310637605524, -4.999999999999980460, -1.548930218128858365E-14 ) ) ;
#15213=PLANE ( 'NONE',  #21867 ) ;
#15214=AXIS2_PLACEMENT_3D ( 'NONE', #15556, #6418, #13573 ) ;
#15215=LINE ( 'NONE', #8355, #19122 ) ;
#15216=EDGE_LOOP ( 'NONE', ( #19184, #23787, #22273, #7297, #16378 ) ) ;
#15217=LINE ( 'NONE', #5933, #19165 ) ;
#15219=VECTOR ( 'NONE', #7307, 1000.000000000000000 ) ;
#15221=DIRECTION ( 'NONE',  ( -2.698458740408365879E-16, 1.000000000000000000, 0.000000000000000000 ) ) ;
#15224=ORIENTED_EDGE ( 'NONE', *, *, #2234, .T. ) ;
#15226=ORIENTED_EDGE ( 'NONE', *, *, #1975, .T. ) ;
#15227=VECTOR ( 'NONE', #21636, 1000.000000000000000 ) ;
#15230=FACE_BOUND ( 'NONE', #26357, .T. ) ;
#15231=ORIENTED_EDGE ( 'NONE', *, *, #12592, .T. ) ;
#15234=CARTESIAN_POINT ( 'NONE',  ( 137.0152310637605808, -10.00000000000000533, -8.721423840594312082 ) ) ;
#15235=EDGE_CURVE ( 'NONE', #18145, #22282, #7627, .T. ) ;
#15237=LINE ( 'NONE', #3366, #22798 ) ;
#15238=EDGE_LOOP ( 'NONE', ( #17385, #23432, #2170, #21993, #11330, #11389 ) ) ;
#15239=VERTEX_POINT ( 'NONE', #18983 ) ;
#15241=DIRECTION ( 'NONE',  ( 0.3090169943749475623, 8.338696094058001131E-17, 0.9510565162951536422 ) ) ;
#15243=ADVANCED_FACE ( 'NONE', ( #11798 ), #19126, .T. ) ;
#15248=ORIENTED_EDGE ( 'NONE', *, *, #9714, .T. ) ;
#15250=ORIENTED_EDGE ( 'NONE', *, *, #20854, .T. ) ;
#15251=DIRECTION ( 'NONE',  ( -0.5877852522924731371, -1.586114251531760728E-16, -0.8090169943749474513 ) ) ;
#15253=VECTOR ( 'NONE', #8616, 1000.000000000000000 ) ;
#15254=CARTESIAN_POINT ( 'NONE',  ( 167.0152310637604103, -4.999999999999972466, -1.854241549900774836E-14 ) ) ;
#15255=FACE_BOUND ( 'NONE', #29221, .T. ) ;
#15256=ORIENTED_EDGE ( 'NONE', *, *, #9505, .F. ) ;
#15260=PLANE ( 'NONE',  #5324 ) ;
#15263=VERTEX_POINT ( 'NONE', #26165 ) ;
#15264=CARTESIAN_POINT ( 'NONE',  ( 175.7287565553229456, -4.999999999999970690, -19.55415080639412295 ) ) ;
#15265=EDGE_LOOP ( 'NONE', ( #12343, #17079, #26064, #24107, #8077 ) ) ;
#15268=AXIS2_PLACEMENT_3D ( 'NONE', #3282, #14543, #24035 ) ;
#15270=PLANE ( 'NONE',  #26381 ) ;
#15273=ORIENTED_EDGE ( 'NONE', *, *, #27360, .F. ) ;
#15277=VERTEX_POINT ( 'NONE', #28181 ) ;
#15278=ORIENTED_EDGE ( 'NONE', *, *, #1667, .F. ) ;
#15279=CARTESIAN_POINT ( 'NONE',  ( 154.5152310637604671, -4.999999999999976019, -1.715463671822630899E-14 ) ) ;
#15281=CARTESIAN_POINT ( 'NONE',  ( 134.5152310637605524, -4.999999999999981348, -4.391296821672111328 ) ) ;
#15286=ORIENTED_EDGE ( 'NONE', *, *, #2681, .T. ) ;
#15287=LINE ( 'NONE', #15449, #18609 ) ;
#15288=CARTESIAN_POINT ( 'NONE',  ( 158.6922820468853672, -10.00000000000000000, -15.07341522555727664 ) ) ;
#15289=VECTOR ( 'NONE', #8205, 1000.000000000000000 ) ;
#15290=LINE ( 'NONE', #5860, #27990 ) ;
#15291=EDGE_CURVE ( 'NONE', #590, #22963, #16689, .T. ) ;
#15292=CARTESIAN_POINT ( 'NONE',  ( 156.1922820468853388, -1.999999999999974909, -2.083034168790677043 ) ) ;
#15293=PLANE ( 'NONE',  #20412 ) ;
#15295=DIRECTION ( 'NONE',  ( -2.698458740408365879E-16, 1.000000000000000000, 0.000000000000000000 ) ) ;
#15299=ORIENTED_EDGE ( 'NONE', *, *, #29241, .F. ) ;
#15301=CARTESIAN_POINT ( 'NONE',  ( 146.1922820468854525, -4.999999999999977796, -19.40354224447947828 ) ) ;
#15302=EDGE_LOOP ( 'NONE', ( #18975, #26758, #1388, #5132 ) ) ;
#15303=LINE ( 'NONE', #19738, #25431 ) ;
#15304=FACE_OUTER_BOUND ( 'NONE', #8893, .T. ) ;
#15305=DIRECTION ( 'NONE',  ( -2.698458740408365879E-16, 1.000000000000000000, 0.000000000000000000 ) ) ;
#15308=ORIENTED_EDGE ( 'NONE', *, *, #13141, .F. ) ;
#15311=DIRECTION ( 'NONE',  ( 0.000000000000000000, -0.000000000000000000, 1.000000000000000000 ) ) ;
#15312=DIRECTION ( 'NONE',  ( -2.698458740408365879E-16, 1.000000000000000000, 0.000000000000000000 ) ) ;
#15315=VECTOR ( 'NONE', #8621, 1000.000000000000000 ) ;
#15316=DIRECTION ( 'NONE',  ( 6.938893903907227392E-16, -0.000000000000000000, 1.000000000000000000 ) ) ;
#15318=EDGE_LOOP ( 'NONE', ( #93, #18025, #9689, #25954 ) ) ;
#15319=CARTESIAN_POINT ( 'NONE',  ( 152.0152310637604671, -10.00000000000000178, -0.06116980274991495881 ) ) ;
#15320=ORIENTED_EDGE ( 'NONE', *, *, #18557, .T. ) ;
#15324=ORIENTED_EDGE ( 'NONE', *, *, #2925, .T. ) ;
#15326=LINE ( 'NONE', #24666, #5530 ) ;
#15328=ADVANCED_FACE ( 'NONE', ( #5241 ), #5092, .F. ) ;
#15329=CARTESIAN_POINT ( 'NONE',  ( 138.6922820468854525, -1.999999999999979572, -26.58683881228715506 ) ) ;
#15332=CARTESIAN_POINT ( 'NONE',  ( 171.1922820468853388, -9.999999999999996447, -19.40354224447947828 ) ) ;
#15333=VECTOR ( 'NONE', #11621, 1000.000000000000000 ) ;
#15339=CARTESIAN_POINT ( 'NONE',  ( 169.7287565553229456, -4.999999999999971578, -25.16025403784439973 ) ) ;
#15342=CARTESIAN_POINT ( 'NONE',  ( 149.5152310637605808, -10.00000000000000178, -30.37205893520531319 ) ) ;
#15344=DIRECTION ( 'NONE',  ( -0.8090169943749474513, -2.183098979609982436E-16, -0.5877852522924731371 ) ) ;
#15348=VECTOR ( 'NONE', #7887, 1000.000000000000000 ) ;
#15349=VERTEX_POINT ( 'NONE', #17726 ) ;
#15350=DIRECTION ( 'NONE',  ( 0.5877852522924731371, 0.000000000000000000, 0.8090169943749474513 ) ) ;
#15351=DIRECTION ( 'NONE',  ( 0.9510565162951536422, 0.000000000000000000, -0.3090169943749475623 ) ) ;
#15352=FACE_OUTER_BOUND ( 'NONE', #8876, .T. ) ;
#15358=CARTESIAN_POINT ( 'NONE',  ( 167.0152310637605240, -9.999999999999996447, -24.27857615940569502 ) ) ;
#15359=FACE_OUTER_BOUND ( 'NONE', #15302, .T. ) ;
#15360=AXIS2_PLACEMENT_3D ( 'NONE', #1248, #29057, #17703 ) ;
#15362=CARTESIAN_POINT ( 'NONE',  ( 157.0152310637605808, -1.999999999999973133, -32.93883019725009120 ) ) ;
#15363=EDGE_CURVE ( 'NONE', #3275, #4291, #3271, .T. ) ;
#15364=VERTEX_POINT ( 'NONE', #20026 ) ;
#15365=FACE_OUTER_BOUND ( 'NONE', #29837, .T. ) ;
#15366=AXIS2_PLACEMENT_3D ( 'NONE', #22225, #24831, #12758 ) ;
#15367=EDGE_CURVE ( 'NONE', #19109, #15010, #21868, .T. ) ;
#15368=DIRECTION ( 'NONE',  ( -2.698458740408365879E-16, 1.000000000000000000, 0.000000000000000000 ) ) ;
#15369=ORIENTED_EDGE ( 'NONE', *, *, #26053, .F. ) ;
#15370=ORIENTED_EDGE ( 'NONE', *, *, #6087, .T. ) ;
#15371=ADVANCED_FACE ( 'NONE', ( #12852 ), #27245, .T. ) ;
#15372=LINE ( 'NONE', #13541, #18543 ) ;
#15374=VECTOR ( 'NONE', #27637, 1000.000000000000000 ) ;
#15375=EDGE_CURVE ( 'NONE', #7486, #12010, #29086, .T. ) ;
#15380=ORIENTED_EDGE ( 'NONE', *, *, #28071, .F. ) ;
#15381=VECTOR ( 'NONE', #20938, 1000.000000000000000 ) ;
#15383=EDGE_LOOP ( 'NONE', ( #6938, #19439, #12720, #25476 ) ) ;
#15384=VECTOR ( 'NONE', #838, 1000.000000000000000 ) ;
#15387=FACE_BOUND ( 'NONE', #8347, .T. ) ;
#15388=VECTOR ( 'NONE', #30048, 999.9999999999998863 ) ;
#15389=ORIENTED_EDGE ( 'NONE', *, *, #11572, .F. ) ;
#15390=DIRECTION ( 'NONE',  ( 0.5877852522924731371, 1.586114251531760728E-16, 0.8090169943749474513 ) ) ;
#15393=DIRECTION ( 'NONE',  ( -0.9510565162951536422, 0.000000000000000000, -0.3090169943749472292 ) ) ;
#15394=ORIENTED_EDGE ( 'NONE', *, *, #10653, .T. ) ;
#15396=VERTEX_POINT ( 'NONE', #6145 ) ;
#15399=VECTOR ( 'NONE', #26042, 1000.000000000000000 ) ;
#15400=CARTESIAN_POINT ( 'NONE',  ( 168.6922820468852819, -9.999999999999998224, 2.247092850131519715 ) ) ;
#15401=VERTEX_POINT ( 'NONE', #24771 ) ;
#15402=LINE ( 'NONE', #22444, #9350 ) ;
#15405=VECTOR ( 'NONE', #24000, 1000.000000000000000 ) ;
#15406=DIRECTION ( 'NONE',  ( 0.9510565162951535312, 2.566386769018988816E-16, -0.3090169943749475623 ) ) ;
#15407=FACE_BOUND ( 'NONE', #17471, .T. ) ;
#15408=EDGE_CURVE ( 'NONE', #21374, #2754, #24464, .T. ) ;
#15409=ORIENTED_EDGE ( 'NONE', *, *, #5813, .T. ) ;
#15415=EDGE_LOOP ( 'NONE', ( #4443, #20541, #24917, #26120 ) ) ;
#15416=EDGE_LOOP ( 'NONE', ( #4181, #23361, #23477, #12663, #16504 ) ) ;
#15417=FACE_OUTER_BOUND ( 'NONE', #20006, .T. ) ;
#15418=AXIS2_PLACEMENT_3D ( 'NONE', #14379, #23716, #14534 ) ;
#15421=CARTESIAN_POINT ( 'NONE',  ( 141.1922820468854525, -10.00000000000000533, -28.06379628232387446 ) ) ;
#15422=VERTEX_POINT ( 'NONE', #19571 ) ;
#15423=AXIS2_PLACEMENT_3D ( 'NONE', #25537, #28326, #660 ) ;
#15425=ORIENTED_EDGE ( 'NONE', *, *, #5333, .T. ) ;
#15430=ORIENTED_EDGE ( 'NONE', *, *, #22704, .F. ) ;
#15432=ORIENTED_EDGE ( 'NONE', *, *, #4609, .F. ) ;
#15436=ORIENTED_EDGE ( 'NONE', *, *, #25290, .T. ) ;
#15439=LINE ( 'NONE', #19712, #23299 ) ;
#15440=DIRECTION ( 'NONE',  ( -2.698458740408365879E-16, 1.000000000000000000, 0.000000000000000000 ) ) ;
#15442=EDGE_CURVE ( 'NONE', #16324, #20167, #29236, .T. ) ;
#15446=ORIENTED_EDGE ( 'NONE', *, *, #18382, .F. ) ;
#15448=ORIENTED_EDGE ( 'NONE', *, *, #194, .F. ) ;
#15449=CARTESIAN_POINT ( 'NONE',  ( 85.18867862981259975, -4.999999999999993783, 61.89319792914030671 ) ) ;
#15450=VECTOR ( 'NONE', #19823, 1000.000000000000000 ) ;
#15452=CARTESIAN_POINT ( 'NONE',  ( 167.2287565553228887, -4.999999999999972466, -3.509618943233414168 ) ) ;
#15453=CARTESIAN_POINT ( 'NONE',  ( 167.0152310637605240, -9.999999999999996447, -34.70218595412750773 ) ) ;
#15455=DIRECTION ( 'NONE',  ( -2.698458740408365879E-16, 1.000000000000000000, 0.000000000000000000 ) ) ;
#15458=LINE ( 'NONE', #8587, #15576 ) ;
#15459=LINE ( 'NONE', #24944, #7612 ) ;
#15462=CARTESIAN_POINT ( 'NONE',  ( 167.0152310637604955, -1.999999999999970912, -26.04193191628311155 ) ) ;
#15464=LINE ( 'NONE', #10431, #12673 ) ;
#15467=ORIENTED_EDGE ( 'NONE', *, *, #28149, .T. ) ;
#15468=CARTESIAN_POINT ( 'NONE',  ( 152.0152310637604671, -4.999999999999976907, -1.687708096207001986E-14 ) ) ;
#15471=DIRECTION ( 'NONE',  ( -0.8090169943749474513, -2.183098979609982436E-16, 0.5877852522924731371 ) ) ;
#15473=EDGE_LOOP ( 'NONE', ( #26878, #19257, #8189, #25216 ) ) ;
#15475=CARTESIAN_POINT ( 'NONE',  ( 118.9351296419579995, -4.999999999999985789, -86.41142975871350984 ) ) ;
#15477=ORIENTED_EDGE ( 'NONE', *, *, #11476, .F. ) ;
#15479=EDGE_CURVE ( 'NONE', #21374, #24767, #8270, .T. ) ;
#15480=ORIENTED_EDGE ( 'NONE', *, *, #5290, .F. ) ;
#15481=( NAMED_UNIT ( * ) PLANE_ANGLE_UNIT ( ) SI_UNIT ( $, .RADIAN. ) );
#15484=ORIENTED_EDGE ( 'NONE', *, *, #9162, .F. ) ;
#15486=AXIS2_PLACEMENT_3D ( 'NONE', #21208, #4886, #14181 ) ;
#15487=DIRECTION ( 'NONE',  ( 0.9510565162951536422, 0.000000000000000000, -0.3090169943749475623 ) ) ;
#15489=DIRECTION ( 'NONE',  ( -0.9510565162951536422, -2.566386769018988816E-16, -0.3090169943749472292 ) ) ;
#15491=LINE ( 'NONE', #6351, #20361 ) ;
#15492=DIRECTION ( 'NONE',  ( 0.5877852522924731371, 1.586114251531760728E-16, 0.8090169943749474513 ) ) ;
#15497=DIRECTION ( 'NONE',  ( -0.9510565162951536422, 0.000000000000000000, -0.3090169943749472292 ) ) ;
#15499=CARTESIAN_POINT ( 'NONE',  ( 141.1922820468854525, -10.00000000000000533, -22.25671179336495697 ) ) ;
#15503=CARTESIAN_POINT ( 'NONE',  ( 154.5152310637605808, -4.999999999999976019, -28.60870317832789667 ) ) ;
#15505=ORIENTED_EDGE ( 'NONE', *, *, #18265, .F. ) ;
#15506=LINE ( 'NONE', #27002, #22719 ) ;
#15507=DIRECTION ( 'NONE',  ( 0.3090169943749475623, 8.338696094058001131E-17, 0.9510565162951536422 ) ) ;
#15508=ORIENTED_EDGE ( 'NONE', *, *, #15201, .F. ) ;
#15511=ORIENTED_EDGE ( 'NONE', *, *, #7240, .F. ) ;
#15514=ADVANCED_FACE ( 'NONE', ( #5699 ), #12702, .T. ) ;
#15515=ADVANCED_FACE ( 'NONE', ( #26777 ), #1428, .T. ) ;
#15518=EDGE_CURVE ( 'NONE', #23642, #12834, #22023, .T. ) ;
#15520=DIRECTION ( 'NONE',  ( -2.698458740408365879E-16, 1.000000000000000000, 0.000000000000000000 ) ) ;
#15521=DIRECTION ( 'NONE',  ( -0.8090169943749474513, -2.183098979609982436E-16, 0.5877852522924731371 ) ) ;
#15523=VECTOR ( 'NONE', #18749, 999.9999999999998863 ) ;
#15526=ORIENTED_EDGE ( 'NONE', *, *, #3036, .T. ) ;
#15527=ORIENTED_EDGE ( 'NONE', *, *, #8149, .T. ) ;
#15532=FACE_OUTER_BOUND ( 'NONE', #10016, .T. ) ;
#15535=VECTOR ( 'NONE', #17801, 1000.000000000000000 ) ;
#15538=ORIENTED_EDGE ( 'NONE', *, *, #8168, .F. ) ;
#15541=LINE ( 'NONE', #2280, #23887 ) ;
#15542=VECTOR ( 'NONE', #4576, 1000.000000000000000 ) ;
#15543=VECTOR ( 'NONE', #17579, 1000.000000000000000 ) ;
#15545=CARTESIAN_POINT ( 'NONE',  ( 134.7287565553230024, -1.999999999999980460, -33.82050807568879947 ) ) ;
#15547=DIRECTION ( 'NONE',  ( -1.110223024625156540E-16, 0.000000000000000000, -1.000000000000000000 ) ) ;
#15548=FACE_OUTER_BOUND ( 'NONE', #28778, .T. ) ;
#15553=EDGE_CURVE ( 'NONE', #14407, #20918, #13605, .T. ) ;
#15554=DIRECTION ( 'NONE',  ( 0.5877852522924731371, 0.000000000000000000, 0.8090169943749474513 ) ) ;
#15556=CARTESIAN_POINT ( 'NONE',  ( 172.0152310637604955, -9.999999999999994671, -24.27857615940569502 ) ) ;
#15557=VECTOR ( 'NONE', #18192, 1000.000000000000000 ) ;
#15559=EDGE_CURVE ( 'NONE', #8863, #2025, #4605, .T. ) ;
#15561=CARTESIAN_POINT ( 'NONE',  ( 153.6922820468854525, -10.00000000000000000, -35.24709285013155835 ) ) ;
#15562=DIRECTION ( 'NONE',  ( -2.698458740408365879E-16, 1.000000000000000000, 0.000000000000000000 ) ) ;
#15564=CARTESIAN_POINT ( 'NONE',  ( 166.1922820468853672, -9.999999999999996447, -28.06379628232387802 ) ) ;
#15566=DIRECTION ( 'NONE',  ( 0.3090169943749472292, 8.338696094057992503E-17, -0.9510565162951536422 ) ) ;
#15567=ORIENTED_EDGE ( 'NONE', *, *, #548, .F. ) ;
#15568=DIRECTION ( 'NONE',  ( 0.5877852522924731371, 0.000000000000000000, 0.8090169943749474513 ) ) ;
#15572=VECTOR ( 'NONE', #19363, 1000.000000000000000 ) ;
#15576=VECTOR ( 'NONE', #4316, 1000.000000000000000 ) ;
#15578=DIRECTION ( 'NONE',  ( 0.9510565162951536422, 2.566386769018988816E-16, 0.3090169943749472292 ) ) ;
#15579=DIRECTION ( 'NONE',  ( -0.9510565162951536422, -2.566386769018988323E-16, 0.3090169943749475623 ) ) ;
#15580=ORIENTED_EDGE ( 'NONE', *, *, #11954, .T. ) ;
#15582=DIRECTION ( 'NONE',  ( -0.9510565162951536422, -2.566386769018988323E-16, 0.3090169943749475623 ) ) ;
#15591=EDGE_CURVE ( 'NONE', #25090, #7345, #13305, .T. ) ;
#15592=LINE ( 'NONE', #13156, #10182 ) ;
#15593=EDGE_CURVE ( 'NONE', #20384, #12010, #23221, .T. ) ;
#15599=CARTESIAN_POINT ( 'NONE',  ( 157.0152310637605240, -4.999999999999975131, -15.61832212156129707 ) ) ;
#15600=VECTOR ( 'NONE', #18398, 1000.000000000000000 ) ;
#15601=CARTESIAN_POINT ( 'NONE',  ( 149.7287565553230309, -1.999999999999975353, -33.82050807568879947 ) ) ;
#15602=DIRECTION ( 'NONE',  ( 0.000000000000000000, 0.000000000000000000, -1.000000000000000000 ) ) ;
#15603=DIRECTION ( 'NONE',  ( -0.9510565162951536422, 0.000000000000000000, -0.3090169943749472292 ) ) ;
#15610=AXIS2_PLACEMENT_3D ( 'NONE', #5156, #12312, #30252 ) ;
#15611=ORIENTED_EDGE ( 'NONE', *, *, #29040, .F. ) ;
#15612=LINE ( 'NONE', #17746, #25659 ) ;
#15614=ORIENTED_EDGE ( 'NONE', *, *, #19722, .T. ) ;
#15617=PLANE ( 'NONE',  #24768 ) ;
#15619=PLANE ( 'NONE',  #10299 ) ;
#15621=ORIENTED_EDGE ( 'NONE', *, *, #22743, .T. ) ;
#15622=ORIENTED_EDGE ( 'NONE', *, *, #24836, .T. ) ;
#15623=CARTESIAN_POINT ( 'NONE',  ( 131.1922820468854241, -4.999999999999982236, -2.083034168790677043 ) ) ;
#15626=DIRECTION ( 'NONE',  ( -2.698458740408365879E-16, 1.000000000000000000, 0.000000000000000000 ) ) ;
#15630=EDGE_LOOP ( 'NONE', ( #5998, #27849, #10359, #11189, #20023 ) ) ;
#15631=ADVANCED_FACE ( 'NONE', ( #27400 ), #18330, .T. ) ;
#15632=LINE ( 'NONE', #29589, #29133 ) ;
#15633=ORIENTED_EDGE ( 'NONE', *, *, #13686, .T. ) ;
#15637=VERTEX_POINT ( 'NONE', #1727 ) ;
#15638=VECTOR ( 'NONE', #28390, 1000.000000000000000 ) ;
#15640=VECTOR ( 'NONE', #1345, 1000.000000000000000 ) ;
#15641=DIRECTION ( 'NONE',  ( -0.9510565162951536422, 0.000000000000000000, -0.3090169943749472292 ) ) ;
#15644=LINE ( 'NONE', #20366, #13145 ) ;
#15645=DIRECTION ( 'NONE',  ( 0.3090169943749472292, 8.338696094057992503E-17, -0.9510565162951536422 ) ) ;
#15646=CARTESIAN_POINT ( 'NONE',  ( 137.0152310637606092, -1.999999999999979572, -15.61832212156129351 ) ) ;
#15650=EDGE_CURVE ( 'NONE', #3131, #24567, #25065, .T. ) ;
#15656=LINE ( 'NONE', #18092, #16843 ) ;
#15658=DIRECTION ( 'NONE',  ( -2.698458740408365879E-16, 1.000000000000000000, 0.000000000000000000 ) ) ;
#15659=DIRECTION ( 'NONE',  ( 0.9510565162951536422, 0.000000000000000000, -0.3090169943749475623 ) ) ;
#15662=VECTOR ( 'NONE', #7234, 999.9999999999998863 ) ;
#15663=DIRECTION ( 'NONE',  ( 1.000000000000000000, 2.168404344971006896E-16, 0.000000000000000000 ) ) ;
#15665=DIRECTION ( 'NONE',  ( -0.5877852522924731371, 0.000000000000000000, 0.8090169943749474513 ) ) ;
#15677=DIRECTION ( 'NONE',  ( 0.5877852522924731371, 1.586114251531760728E-16, 0.8090169943749474513 ) ) ;
#15678=VERTEX_POINT ( 'NONE', #24925 ) ;
#15679=FACE_OUTER_BOUND ( 'NONE', #5240, .T. ) ;
#15680=PLANE ( 'NONE',  #7013 ) ;
#15682=CARTESIAN_POINT ( 'NONE',  ( 149.5152310637605808, -4.999999999999976907, -1.659952520591374334E-14 ) ) ;
#15683=EDGE_CURVE ( 'NONE', #19711, #8784, #27541, .T. ) ;
#15689=EDGE_CURVE ( 'NONE', #21114, #24657, #8871, .T. ) ;
#15691=PLANE ( 'NONE',  #11364 ) ;
#15693=CYLINDRICAL_SURFACE ( 'NONE', #20435, 3.000000000000002665 ) ;
#15694=ORIENTED_EDGE ( 'NONE', *, *, #21900, .F. ) ;
#15695=DIRECTION ( 'NONE',  ( 0.5877852522924731371, 1.586114251531760728E-16, 0.8090169943749474513 ) ) ;
#15699=VERTEX_POINT ( 'NONE', #15885 ) ;
#15701=VERTEX_POINT ( 'NONE', #18489 ) ;
#15705=ORIENTED_EDGE ( 'NONE', *, *, #27930, .T. ) ;
#15706=DIRECTION ( 'NONE',  ( -0.9510565162951536422, -2.566386769018988816E-16, -0.3090169943749472292 ) ) ;
#15707=CARTESIAN_POINT ( 'NONE',  ( 132.2287565553230024, -10.00000000000000888, -29.49038105676660138 ) ) ;
#15709=VECTOR ( 'NONE', #4865, 999.9999999999998863 ) ;
#15710=CARTESIAN_POINT ( 'NONE',  ( 176.1922820468852535, -9.999999999999994671, -2.083034168790677043 ) ) ;
#15712=VECTOR ( 'NONE', #29786, 1000.000000000000000 ) ;
#15713=ORIENTED_EDGE ( 'NONE', *, *, #5510, .F. ) ;
#15715=EDGE_CURVE ( 'NONE', #12381, #17616, #13750, .T. ) ;
#15716=CARTESIAN_POINT ( 'NONE',  ( 154.5152310637604955, -4.999999999999976019, -13.05155085951651195 ) ) ;
#15717=DIRECTION ( 'NONE',  ( 1.000000000000000000, 2.891205793294675861E-16, 0.000000000000000000 ) ) ;
#15719=EDGE_CURVE ( 'NONE', #22060, #11457, #11453, .T. ) ;
#15721=CARTESIAN_POINT ( 'NONE',  ( 143.6922820468854241, -1.999999999999978018, -6.413161187712876909 ) ) ;
#15726=ORIENTED_EDGE ( 'NONE', *, *, #14952, .T. ) ;
#15730=CARTESIAN_POINT ( 'NONE',  ( 167.0152310637604671, -4.999999999999972466, -1.854241549900775467E-14 ) ) ;
#15731=VERTEX_POINT ( 'NONE', #25514 ) ;
#15732=CARTESIAN_POINT ( 'NONE',  ( 126.7486941615241989, -4.999999999999984013, -92.08831667749211647 ) ) ;
#15737=EDGE_LOOP ( 'NONE', ( #2217, #1312, #9541, #8001 ) ) ;
#15739=AXIS2_PLACEMENT_3D ( 'NONE', #29161, #29639, #6078 ) ;
#15744=ORIENTED_EDGE ( 'NONE', *, *, #11879, .F. ) ;
#15745=CARTESIAN_POINT ( 'NONE',  ( 146.1922820468854241, -1.999999999999977573, -13.59645775552055902 ) ) ;
#15746=LINE ( 'NONE', #15897, #13497 ) ;
#15747=PLANE ( 'NONE',  #8233 ) ;
#15749=DIRECTION ( 'NONE',  ( 0.9510565162951536422, 2.566386769018988816E-16, 0.3090169943749472292 ) ) ;
#15752=ADVANCED_FACE ( 'NONE', ( #16496 ), #9773, .T. ) ;
#15753=EDGE_CURVE ( 'NONE', #23552, #9765, #28444, .T. ) ;
#15755=EDGE_CURVE ( 'NONE', #11857, #29468, #11907, .T. ) ;
#15757=ORIENTED_EDGE ( 'NONE', *, *, #29864, .T. ) ;
#15758=CYLINDRICAL_SURFACE ( 'NONE', #6668, 8.000000000000007105 ) ;
#15759=ORIENTED_EDGE ( 'NONE', *, *, #681, .T. ) ;
#15761=PLANE ( 'NONE',  #15486 ) ;
#15763=CARTESIAN_POINT ( 'NONE',  ( 130.4440631633587202, -4.999999999999982236, -94.77315941399760391 ) ) ;
#15764=CARTESIAN_POINT ( 'NONE',  ( 149.5152310637605808, -4.999999999999976907, -30.37205893520531319 ) ) ;
#15766=VERTEX_POINT ( 'NONE', #4752 ) ;
#15767=EDGE_LOOP ( 'NONE', ( #755, #8072, #30034, #25994 ) ) ;
#15768=CARTESIAN_POINT ( 'NONE',  ( 146.1922820468854525, -1.999999999999977129, -30.91696583120935671 ) ) ;
#15771=DIRECTION ( 'NONE',  ( 0.5877852522924731371, 1.586114251531760728E-16, -0.8090169943749474513 ) ) ;
#15775=ORIENTED_EDGE ( 'NONE', *, *, #12511, .F. ) ;
#15783=CARTESIAN_POINT ( 'NONE',  ( 134.5152310637605524, -4.999999999999981348, -1.493419066897600538E-14 ) ) ;
#15784=CARTESIAN_POINT ( 'NONE',  ( 134.5152310637605524, -4.999999999999981348, -21.71180489736090991 ) ) ;
#15785=DIRECTION ( 'NONE',  ( 0.000000000000000000, 0.000000000000000000, -1.000000000000000000 ) ) ;
#15786=DIRECTION ( 'NONE',  ( -0.9510565162951536422, -2.566386769018988816E-16, -0.3090169943749472292 ) ) ;
#15787=EDGE_CURVE ( 'NONE', #22258, #117, #5362, .T. ) ;
#15788=PLANE ( 'NONE',  #10440 ) ;
#15789=EDGE_CURVE ( 'NONE', #16318, #18472, #7495, .T. ) ;
#15791=EDGE_CURVE ( 'NONE', #9240, #3706, #2933, .T. ) ;
#15797=VECTOR ( 'NONE', #9399, 1000.000000000000000 ) ;
#15799=DIRECTION ( 'NONE',  ( -2.698458740408365879E-16, 1.000000000000000000, 0.000000000000000000 ) ) ;
#15801=CARTESIAN_POINT ( 'NONE',  ( 162.2287565553229456, -9.999999999999998224, -20.83012701892220520 ) ) ;
#15802=ORIENTED_EDGE ( 'NONE', *, *, #15166, .T. ) ;
#15805=EDGE_LOOP ( 'NONE', ( #110, #25194, #459, #11392, #7343 ) ) ;
#15806=DIRECTION ( 'NONE',  ( -0.9510565162951536422, 0.000000000000000000, -0.3090169943749472292 ) ) ;
#15807=CARTESIAN_POINT ( 'NONE',  ( 139.5152310637606092, -1.999999999999978684, -28.60870317832789311 ) ) ;
#15808=DIRECTION ( 'NONE',  ( -0.8090169943749474513, -2.183098979609982436E-16, -0.5877852522924731371 ) ) ;
#15810=VECTOR ( 'NONE', #4765, 1000.000000000000000 ) ;
#15811=ORIENTED_EDGE ( 'NONE', *, *, #12035, .F. ) ;
#15816=LINE ( 'NONE', #6383, #16202 ) ;
#15820=ORIENTED_EDGE ( 'NONE', *, *, #20289, .T. ) ;
#15822=CARTESIAN_POINT ( 'NONE',  ( 113.6585242177747972, -4.999999999999986677, -82.57775151454063689 ) ) ;
#15823=ORIENTED_EDGE ( 'NONE', *, *, #7117, .T. ) ;
#15824=LINE ( 'NONE', #1821, #26863 ) ;
#15828=ORIENTED_EDGE ( 'NONE', *, *, #15854, .T. ) ;
#15830=VERTEX_POINT ( 'NONE', #19833 ) ;
#15831=LINE ( 'NONE', #25162, #6873 ) ;
#15832=LINE ( 'NONE', #3180, #7976 ) ;
#15834=PLANE ( 'NONE',  #16568 ) ;
#15835=ORIENTED_EDGE ( 'NONE', *, *, #6915, .F. ) ;
#15836=LINE ( 'NONE', #25319, #13436 ) ;
#15838=LINE ( 'NONE', #29814, #1986 ) ;
#15839=DIRECTION ( 'NONE',  ( -0.8090169943749474513, -2.183098979609982436E-16, -0.5877852522924731371 ) ) ;
#15840=EDGE_LOOP ( 'NONE', ( #11273, #6033, #26893, #1537 ) ) ;
#15841=ORIENTED_EDGE ( 'NONE', *, *, #22911, .F. ) ;
#15842=ORIENTED_EDGE ( 'NONE', *, *, #25287, .T. ) ;
#15843=CARTESIAN_POINT ( 'NONE',  ( 157.0152310637605524, -4.999999999999975131, -34.70218595412750773 ) ) ;
#15846=EDGE_LOOP ( 'NONE', ( #13033, #26463, #1214, #13901, #6286 ) ) ;
#15850=CARTESIAN_POINT ( 'NONE',  ( 173.6922820468853672, -9.999999999999994671, -32.39392330124607611 ) ) ;
#15851=DIRECTION ( 'NONE',  ( 0.9510565162951535312, 2.566386769018988816E-16, -0.3090169943749475623 ) ) ;
#15853=EDGE_CURVE ( 'NONE', #22258, #13830, #26901, .T. ) ;
#15854=EDGE_CURVE ( 'NONE', #16825, #6890, #5962, .T. ) ;
#15856=DIRECTION ( 'NONE',  ( -0.5877852522924731371, -1.586114251531760235E-16, 0.8090169943749474513 ) ) ;
#15858=VECTOR ( 'NONE', #14807, 1000.000000000000000 ) ;
#15860=ORIENTED_EDGE ( 'NONE', *, *, #21558, .T. ) ;
#15861=CARTESIAN_POINT ( 'NONE',  ( 146.1922820468854525, -10.00000000000000178, -19.40354224447947828 ) ) ;
#15865=ORIENTED_EDGE ( 'NONE', *, *, #18168, .T. ) ;
#15866=CARTESIAN_POINT ( 'NONE',  ( 133.7287565553229172, -9.999999999999980460, -33.50000000000000000 ) ) ;
#15870=ORIENTED_EDGE ( 'NONE', *, *, #23847, .F. ) ;
#15871=PLANE ( 'NONE',  #13719 ) ;
#15874=CARTESIAN_POINT ( 'NONE',  ( 153.6922820468854241, -4.999999999999976019, -23.73366926340167637 ) ) ;
#15875=CARTESIAN_POINT ( 'NONE',  ( 154.5152310637605524, -4.999999999999976019, -30.37205893520531319 ) ) ;
#15876=ORIENTED_EDGE ( 'NONE', *, *, #26528, .F. ) ;
#15880=VECTOR ( 'NONE', #26526, 1000.000000000000000 ) ;
#15885=CARTESIAN_POINT ( 'NONE',  ( 134.5152310637605808, -1.999999999999980460, -28.60870317832789311 ) ) ;
#15889=ADVANCED_FACE ( 'NONE', ( #1391 ), #24278, .T. ) ;
#15891=EDGE_CURVE ( 'NONE', #27920, #25350, #15402, .T. ) ;
#15893=EDGE_CURVE ( 'NONE', #20965, #22051, #17100, .T. ) ;
#15894=ORIENTED_EDGE ( 'NONE', *, *, #4697, .T. ) ;
#15896=AXIS2_PLACEMENT_3D ( 'NONE', #12887, #22061, #10444 ) ;
#15897=CARTESIAN_POINT ( 'NONE',  ( 153.6922820468853672, -10.00000000000000178, -9.266330736598359152 ) ) ;
#15898=FACE_OUTER_BOUND ( 'NONE', #6763, .T. ) ;
#15899=VECTOR ( 'NONE', #11636, 1000.000000000000000 ) ;
#15901=VECTOR ( 'NONE', #4426, 1000.000000000000000 ) ;
#15905=CARTESIAN_POINT ( 'NONE',  ( 151.1922820468853672, -1.999999999999976241, -2.083034168790677043 ) ) ;
#15906=ORIENTED_EDGE ( 'NONE', *, *, #24246, .T. ) ;
#15909=LINE ( 'NONE', #25389, #12190 ) ;
#15910=LINE ( 'NONE', #4326, #17988 ) ;
#15912=EDGE_LOOP ( 'NONE', ( #21949, #3130, #4247, #28737 ) ) ;
#15913=VERTEX_POINT ( 'NONE', #5512 ) ;
#15914=CARTESIAN_POINT ( 'NONE',  ( 152.0152310637604955, -10.00000000000000178, -8.721423840594312082 ) ) ;
#15919=CARTESIAN_POINT ( 'NONE',  ( 168.6922820468853956, -9.999999999999996447, -32.39392330124607611 ) ) ;
#15921=DIRECTION ( 'NONE',  ( -2.698458740408365879E-16, 1.000000000000000000, 0.000000000000000000 ) ) ;
#15923=ORIENTED_EDGE ( 'NONE', *, *, #15553, .T. ) ;
#15926=VECTOR ( 'NONE', #21328, 1000.000000000000000 ) ;
#15928=EDGE_CURVE ( 'NONE', #28006, #20351, #10223, .T. ) ;
#15931=EDGE_CURVE ( 'NONE', #3131, #4293, #2000, .T. ) ;
#15932=EDGE_CURVE ( 'NONE', #11734, #11863, #29516, .T. ) ;
#15933=EDGE_LOOP ( 'NONE', ( #6787, #25506, #13202, #10879 ) ) ;
#15934=ORIENTED_EDGE ( 'NONE', *, *, #18379, .F. ) ;
#15937=CARTESIAN_POINT ( 'NONE',  ( 163.6922820468853388, -1.999999999999973133, -23.73366926340167282 ) ) ;
#15938=PLANE ( 'NONE',  #5861 ) ;
#15939=CARTESIAN_POINT ( 'NONE',  ( 139.5152310637605808, -1.999999999999978684, -30.37205893520530964 ) ) ;
#15942=DIRECTION ( 'NONE',  ( 1.000000000000000000, 2.698458740408365879E-16, -1.110223024625156540E-16 ) ) ;
#15946=AXIS2_PLACEMENT_3D ( 'NONE', #23788, #22198, #19909 ) ;
#15951=DIRECTION ( 'NONE',  ( 0.3090169943749475623, 8.338696094058001131E-17, 0.9510565162951536422 ) ) ;
#15952=EDGE_LOOP ( 'NONE', ( #14985, #20616, #17171, #25653 ) ) ;
#15957=CARTESIAN_POINT ( 'NONE',  ( 152.0152310637605808, -10.00000000000000000, -34.70218595412750773 ) ) ;
#15958=DIRECTION ( 'NONE',  ( 0.9510565162951536422, 0.000000000000000000, -0.3090169943749475623 ) ) ;
#15959=ORIENTED_EDGE ( 'NONE', *, *, #14574, .F. ) ;
#15960=ORIENTED_EDGE ( 'NONE', *, *, #25246, .T. ) ;
#15965=EDGE_CURVE ( 'NONE', #2298, #21422, #20587, .T. ) ;
#15967=ADVANCED_FACE ( 'NONE', ( #27209 ), #29969, .T. ) ;
#15968=VECTOR ( 'NONE', #1683, 1000.000000000000000 ) ;
#15969=EDGE_CURVE ( 'NONE', #27920, #2723, #11133, .T. ) ;
#15971=EDGE_CURVE ( 'NONE', #3306, #18890, #4424, .T. ) ;
#15973=VECTOR ( 'NONE', #28442, 1000.000000000000000 ) ;
#15974=EDGE_LOOP ( 'NONE', ( #14596, #26109, #536, #21734 ) ) ;
#15977=ORIENTED_EDGE ( 'NONE', *, *, #5010, .F. ) ;
#15979=CARTESIAN_POINT ( 'NONE',  ( 153.6922820468854241, -1.999999999999974909, -26.58683881228715862 ) ) ;
#15983=ORIENTED_EDGE ( 'NONE', *, *, #8242, .T. ) ;
#15988=CARTESIAN_POINT ( 'NONE',  ( 172.7287565553229456, -1.999999999999970468, 0.5000000000000029976 ) ) ;
#15989=DIRECTION ( 'NONE',  ( -0.9510565162951536422, -2.566386769018988816E-16, -0.3090169943749472292 ) ) ;
#15990=ORIENTED_EDGE ( 'NONE', *, *, #19896, .T. ) ;
#15991=AXIS2_PLACEMENT_3D ( 'NONE', #7902, #5621, #5470 ) ;
#15992=DIRECTION ( 'NONE',  ( 0.3090169943749472292, 8.338696094057992503E-17, -0.9510565162951536422 ) ) ;
#15993=DIRECTION ( 'NONE',  ( -0.9510565162951536422, -2.566386769018988816E-16, -0.3090169943749472292 ) ) ;
#15994=ORIENTED_EDGE ( 'NONE', *, *, #15363, .F. ) ;
#15996=LINE ( 'NONE', #4264, #17386 ) ;
#15997=VECTOR ( 'NONE', #5471, 1000.000000000000000 ) ;
#16003=LINE ( 'NONE', #13415, #27738 ) ;
#16004=EDGE_CURVE ( 'NONE', #10540, #24599, #20282, .T. ) ;
#16005=DIRECTION ( 'NONE',  ( -0.9510565162951536422, -2.566386769018988816E-16, -0.3090169943749472292 ) ) ;
#16006=ADVANCED_FACE ( 'NONE', ( #13718 ), #4273, .F. ) ;
#16007=VERTEX_POINT ( 'NONE', #8683 ) ;
#16010=LINE ( 'NONE', #8539, #9358 ) ;
#16012=VECTOR ( 'NONE', #20333, 1000.000000000000000 ) ;
#16013=AXIS2_PLACEMENT_3D ( 'NONE', #26094, #453, #16310 ) ;
#16015=CARTESIAN_POINT ( 'NONE',  ( 14.97564302476352971, -5.000000000000013323, 46.09028999592811005 ) ) ;
#16016=FACE_OUTER_BOUND ( 'NONE', #9831, .T. ) ;
#16017=ORIENTED_EDGE ( 'NONE', *, *, #25044, .T. ) ;
#16018=ORIENTED_EDGE ( 'NONE', *, *, #30122, .T. ) ;
#16019=LINE ( 'NONE', #18009, #20714 ) ;
#16022=CARTESIAN_POINT ( 'NONE',  ( 172.0152310637605240, -1.999999999999969358, -32.93883019725009120 ) ) ;
#16023=ORIENTED_EDGE ( 'NONE', *, *, #18448, .F. ) ;
#16024=EDGE_CURVE ( 'NONE', #30179, #17865, #18148, .T. ) ;
#16025=VERTEX_POINT ( 'NONE', #8536 ) ;
#16029=DIRECTION ( 'NONE',  ( -0.8090169943749474513, -2.183098979609982436E-16, 0.5877852522924731371 ) ) ;
#16030=LINE ( 'NONE', #1712, #2814 ) ;
#16032=VERTEX_POINT ( 'NONE', #20137 ) ;
#16034=VECTOR ( 'NONE', #27702, 1000.000000000000000 ) ;
#16037=ORIENTED_EDGE ( 'NONE', *, *, #2235, .T. ) ;
#16038=DIRECTION ( 'NONE',  ( -0.5877852522924731371, 0.000000000000000000, 0.8090169943749474513 ) ) ;
#16039=AXIS2_PLACEMENT_3D ( 'NONE', #17876, #4013, #29411 ) ;
#16040=DIRECTION ( 'NONE',  ( -2.698458740408365879E-16, 1.000000000000000000, 0.000000000000000000 ) ) ;
#16044=ORIENTED_EDGE ( 'NONE', *, *, #14160, .T. ) ;
#16045=CARTESIAN_POINT ( 'NONE',  ( 161.1922820468853388, -4.999999999999973355, -13.59645775552055902 ) ) ;
#16046=ORIENTED_EDGE ( 'NONE', *, *, #10517, .F. ) ;
#16047=LINE ( 'NONE', #25522, #1856 ) ;
#16048=VECTOR ( 'NONE', #13286, 1000.000000000000000 ) ;
#16049=DIRECTION ( 'NONE',  ( -2.698458740408365879E-16, 1.000000000000000000, 0.000000000000000000 ) ) ;
#16050=DIRECTION ( 'NONE',  ( 0.5877852522924731371, 0.000000000000000000, 0.8090169943749474513 ) ) ;
#16054=EDGE_CURVE ( 'NONE', #16025, #1829, #13416, .T. ) ;
#16055=ADVANCED_FACE ( 'NONE', ( #11421 ), #17991, .T. ) ;
#16058=EDGE_LOOP ( 'NONE', ( #9716, #6620, #22526, #23949 ) ) ;
#16060=ADVANCED_FACE ( 'NONE', ( #8977 ), #2294, .T. ) ;
#16062=DIRECTION ( 'NONE',  ( -0.9510565162951536422, -2.566386769018988323E-16, 0.3090169943749475623 ) ) ;
#16063=CARTESIAN_POINT ( 'NONE',  ( 144.7287565553230309, -1.999999999999977129, -25.16025403784439973 ) ) ;
#16064=EDGE_CURVE ( 'NONE', #16652, #11518, #1692, .T. ) ;
#16065=LINE ( 'NONE', #30178, #18529 ) ;
#16066=ORIENTED_EDGE ( 'NONE', *, *, #7837, .T. ) ;
#16067=ORIENTED_EDGE ( 'NONE', *, *, #18138, .F. ) ;
#16068=LINE ( 'NONE', #27717, #7120 ) ;
#16071=CARTESIAN_POINT ( 'NONE',  ( 132.0152310637605808, -1.999999999999981348, -24.27857615940569147 ) ) ;
#16072=FACE_OUTER_BOUND ( 'NONE', #20911, .T. ) ;
#16078=AXIS2_PLACEMENT_3D ( 'NONE', #19483, #26844, #19627 ) ;
#16081=VECTOR ( 'NONE', #16996, 1000.000000000000000 ) ;
#16082=VECTOR ( 'NONE', #23773, 1000.000000000000000 ) ;
#16083=ORIENTED_EDGE ( 'NONE', *, *, #14439, .F. ) ;
#16085=CARTESIAN_POINT ( 'NONE',  ( 152.0152310637604955, -4.999999999999976907, -8.721423840594312082 ) ) ;
#16086=ORIENTED_EDGE ( 'NONE', *, *, #28876, .F. ) ;
#16087=CARTESIAN_POINT ( 'NONE',  ( 167.2287565553229172, -9.999999999999998224, -12.16987298107780369 ) ) ;
#16088=VECTOR ( 'NONE', #207, 999.9999999999998863 ) ;
#16089=LINE ( 'NONE', #2082, #5765 ) ;
#16090=DIRECTION ( 'NONE',  ( 0.9510565162951536422, 0.000000000000000000, -0.3090169943749475623 ) ) ;
#16091=DIRECTION ( 'NONE',  ( -0.9510565162951536422, 0.000000000000000000, -0.3090169943749472292 ) ) ;
#16096=VECTOR ( 'NONE', #19652, 1000.000000000000000 ) ;
#16097=CARTESIAN_POINT ( 'NONE',  ( 154.5152310637604671, -1.999999999999975353, -4.391296821672111328 ) ) ;
#16099=EDGE_CURVE ( 'NONE', #6302, #29149, #28552, .T. ) ;
#16100=EDGE_CURVE ( 'NONE', #20699, #28260, #26088, .T. ) ;
#16101=FACE_OUTER_BOUND ( 'NONE', #15952, .T. ) ;
#16102=CARTESIAN_POINT ( 'NONE',  ( 14.97081799254939050, -5.000000000000013323, -46.07544007371636496 ) ) ;
#16103=EDGE_CURVE ( 'NONE', #4171, #17166, #7308, .T. ) ;
#16106=ORIENTED_EDGE ( 'NONE', *, *, #18692, .F. ) ;
#16107=DIRECTION ( 'NONE',  ( -2.698458740408365879E-16, 1.000000000000000000, 0.000000000000000000 ) ) ;
#16109=ORIENTED_EDGE ( 'NONE', *, *, #6265, .F. ) ;
#16110=CARTESIAN_POINT ( 'NONE',  ( 141.1922820468854525, -10.00000000000000533, -13.59645775552055902 ) ) ;
#16111=CARTESIAN_POINT ( 'NONE',  ( 174.5152310637604955, -1.999999999999968914, -28.60870317832789667 ) ) ;
#16113=DIRECTION ( 'NONE',  ( 1.000000000000000000, 2.698458740408365879E-16, -1.110223024625156540E-16 ) ) ;
#16114=ORIENTED_EDGE ( 'NONE', *, *, #1969, .F. ) ;
#16117=AXIS2_PLACEMENT_3D ( 'NONE', #20388, #20238, #15958 ) ;
#16119=VECTOR ( 'NONE', #325, 1000.000000000000000 ) ;
#16121=CARTESIAN_POINT ( 'NONE',  ( 149.5152310637605240, -1.999999999999976241, -13.05155085951651195 ) ) ;
#16125=EDGE_CURVE ( 'NONE', #21788, #8702, #2595, .T. ) ;
#16126=CARTESIAN_POINT ( 'NONE',  ( 137.0152310637605808, -10.00000000000000533, -26.04193191628310800 ) ) ;
#16127=ORIENTED_EDGE ( 'NONE', *, *, #19880, .T. ) ;
#16131=LINE ( 'NONE', #15682, #4395 ) ;
#16133=AXIS2_PLACEMENT_3D ( 'NONE', #27281, #6626, #17760 ) ;
#16135=ORIENTED_EDGE ( 'NONE', *, *, #10213, .T. ) ;
#16137=EDGE_CURVE ( 'NONE', #19023, #19635, #9276, .T. ) ;
#16140=ADVANCED_FACE ( 'NONE', ( #28097 ), #25933, .T. ) ;
#16142=CARTESIAN_POINT ( 'NONE',  ( 148.6922820468854525, -10.00000000000000178, -35.24709285013155835 ) ) ;
#16143=EDGE_CURVE ( 'NONE', #4706, #1754, #4711, .T. ) ;
#16144=ORIENTED_EDGE ( 'NONE', *, *, #11954, .F. ) ;
#16145=CARTESIAN_POINT ( 'NONE',  ( 172.2287565553229456, -4.999999999999970690, -20.83012701892220164 ) ) ;
#16146=ORIENTED_EDGE ( 'NONE', *, *, #11110, .F. ) ;
#16147=LINE ( 'NONE', #11268, #14412 ) ;
#16150=ORIENTED_EDGE ( 'NONE', *, *, #24705, .T. ) ;
#16155=DIRECTION ( 'NONE',  ( -0.8090169943749474513, -2.183098979609982436E-16, 0.5877852522924731371 ) ) ;
#16156=CARTESIAN_POINT ( 'NONE',  ( 13.61739406634275618, -5.000000000000014211, -41.91002953721110202 ) ) ;
#16157=CARTESIAN_POINT ( 'NONE',  ( 153.6922820468854525, -1.999999999999974465, -35.24709285013155835 ) ) ;
#16162=CARTESIAN_POINT ( 'NONE',  ( 137.0152310637606092, -1.999999999999979572, -32.93883019725009120 ) ) ;
#16163=LINE ( 'NONE', #20440, #1115 ) ;
#16166=LINE ( 'NONE', #11730, #19009 ) ;
#16170=CARTESIAN_POINT ( 'NONE',  ( 82.76178917566952009, -4.999999999999994671, 60.12995952993764348 ) ) ;
#16171=ORIENTED_EDGE ( 'NONE', *, *, #1415, .T. ) ;
#16174=CARTESIAN_POINT ( 'NONE',  ( 147.0152310637604955, -1.999999999999977573, -0.06116980274991495881 ) ) ;
#16175=AXIS2_PLACEMENT_3D ( 'NONE', #8388, #17692, #27053 ) ;
#16179=EDGE_CURVE ( 'NONE', #28260, #7113, #23959, .T. ) ;
#16181=ORIENTED_EDGE ( 'NONE', *, *, #270, .T. ) ;
#16182=ORIENTED_EDGE ( 'NONE', *, *, #19880, .F. ) ;
#16185=FACE_OUTER_BOUND ( 'NONE', #6252, .T. ) ;
#16186=CARTESIAN_POINT ( 'NONE',  ( 143.6922820468853956, -10.00000000000000533, -0.6060766987539614181 ) ) ;
#16187=ORIENTED_EDGE ( 'NONE', *, *, #27289, .F. ) ;
#16188=ORIENTED_EDGE ( 'NONE', *, *, #19614, .T. ) ;
#16190=VERTEX_POINT ( 'NONE', #23487 ) ;
#16194=VECTOR ( 'NONE', #4466, 1000.000000000000000 ) ;
#16195=ORIENTED_EDGE ( 'NONE', *, *, #7085, .F. ) ;
#16201=ORIENTED_EDGE ( 'NONE', *, *, #22669, .T. ) ;
#16202=VECTOR ( 'NONE', #25143, 1000.000000000000000 ) ;
#16204=ADVANCED_FACE ( 'NONE', ( #7461 ), #4859, .T. ) ;
#16205=DIRECTION ( 'NONE',  ( 0.9510565162951535312, 2.566386769018988816E-16, -0.3090169943749475623 ) ) ;
#16207=LINE ( 'NONE', #4165, #15557 ) ;
#16212=ORIENTED_EDGE ( 'NONE', *, *, #817, .T. ) ;
#16213=CARTESIAN_POINT ( 'NONE',  ( 162.0152310637604955, -4.999999999999973355, -15.61832212156129707 ) ) ;
#16214=ORIENTED_EDGE ( 'NONE', *, *, #28616, .F. ) ;
#16216=VECTOR ( 'NONE', #13970, 1000.000000000000000 ) ;
#16218=DIRECTION ( 'NONE',  ( -2.698458740408365879E-16, 1.000000000000000000, 0.000000000000000000 ) ) ;
#16219=LINE ( 'NONE', #1751, #7653 ) ;
#16221=ORIENTED_EDGE ( 'NONE', *, *, #14402, .T. ) ;
#16222=VERTEX_POINT ( 'NONE', #20881 ) ;
#16223=LINE ( 'NONE', #23866, #8581 ) ;
#16225=ORIENTED_EDGE ( 'NONE', *, *, #1553, .T. ) ;
#16229=PLANE ( 'NONE',  #26211 ) ;
#16231=VERTEX_POINT ( 'NONE', #294 ) ;
#16232=DIRECTION ( 'NONE',  ( -0.8090169943749474513, -2.183098979609982436E-16, -0.5877852522924731371 ) ) ;
#16237=LINE ( 'NONE', #2225, #2474 ) ;
#16238=EDGE_CURVE ( 'NONE', #6539, #24548, #5015, .T. ) ;
#16239=VECTOR ( 'NONE', #27130, 1000.000000000000000 ) ;
#16240=DIRECTION ( 'NONE',  ( 0.5877852522924731371, 0.000000000000000000, 0.8090169943749474513 ) ) ;
#16241=CARTESIAN_POINT ( 'NONE',  ( 132.0152310637605524, -1.999999999999981348, -26.04193191628310800 ) ) ;
#16242=CARTESIAN_POINT ( 'NONE',  ( 157.0152310637605240, -10.00000000000000000, -15.61832212156129707 ) ) ;
#16248=DIRECTION ( 'NONE',  ( -0.5877852522924731371, -1.586114251531760728E-16, -0.8090169943749474513 ) ) ;
#16249=CARTESIAN_POINT ( 'NONE',  ( 131.1922820468854241, -1.999999999999982236, -13.59645775552055547 ) ) ;
#16252=VERTEX_POINT ( 'NONE', #18903 ) ;
#16257=CARTESIAN_POINT ( 'NONE',  ( 159.5152310637605240, -1.999999999999973133, -19.94844914048349693 ) ) ;
#16259=VECTOR ( 'NONE', #18611, 1000.000000000000000 ) ;
#16260=EDGE_LOOP ( 'NONE', ( #8606, #12535, #27234, #25536 ) ) ;
#16262=ORIENTED_EDGE ( 'NONE', *, *, #5811, .F. ) ;
#16267=EDGE_CURVE ( 'NONE', #28698, #29509, #7011, .T. ) ;
#16268=EDGE_CURVE ( 'NONE', #4554, #18145, #12021, .T. ) ;
#16269=VERTEX_POINT ( 'NONE', #21494 ) ;
#16271=DIRECTION ( 'NONE',  ( 0.9510565162951536422, 0.000000000000000000, -0.3090169943749475623 ) ) ;
#16273=ORIENTED_EDGE ( 'NONE', *, *, #10448, .T. ) ;
#16280=VERTEX_POINT ( 'NONE', #5474 ) ;
#16282=CARTESIAN_POINT ( 'NONE',  ( 161.1922820468853104, -1.999999999999974021, -4.936203717676158398 ) ) ;
#16285=LINE ( 'NONE', #9711, #18989 ) ;
#16286=FACE_OUTER_BOUND ( 'NONE', #6106, .T. ) ;
#16288=DIRECTION ( 'NONE',  ( -2.698458740408365879E-16, 1.000000000000000000, 0.000000000000000000 ) ) ;
#16290=ORIENTED_EDGE ( 'NONE', *, *, #1458, .T. ) ;
#16291=DIRECTION ( 'NONE',  ( -0.5877852522924731371, -1.586114251531760728E-16, -0.8090169943749474513 ) ) ;
#16292=ORIENTED_EDGE ( 'NONE', *, *, #23952, .F. ) ;
#16294=ORIENTED_EDGE ( 'NONE', *, *, #1346, .F. ) ;
#16297=ORIENTED_EDGE ( 'NONE', *, *, #18366, .T. ) ;
#16299=LINE ( 'NONE', #25614, #8672 ) ;
#16301=VECTOR ( 'NONE', #29416, 1000.000000000000000 ) ;
#16305=EDGE_CURVE ( 'NONE', #23467, #29073, #21947, .T. ) ;
#16306=ADVANCED_FACE ( 'NONE', ( #6074 ), #14757, .T. ) ;
#16308=EDGE_CURVE ( 'NONE', #24567, #27103, #26862, .T. ) ;
#16309=DIRECTION ( 'NONE',  ( -2.698458740408365879E-16, 1.000000000000000000, 0.000000000000000000 ) ) ;
#16310=DIRECTION ( 'NONE',  ( -0.9510565162951536422, 0.000000000000000000, -0.3090169943749472292 ) ) ;
#16311=CARTESIAN_POINT ( 'NONE',  ( 162.0152310637605240, -4.999999999999974243, -1.798730398669518271E-14 ) ) ;
#16314=FACE_OUTER_BOUND ( 'NONE', #8947, .T. ) ;
#16316=ORIENTED_EDGE ( 'NONE', *, *, #13008, .F. ) ;
#16318=VERTEX_POINT ( 'NONE', #24245 ) ;
#16319=DIRECTION ( 'NONE',  ( 0.5877852522924731371, 1.586114251531760728E-16, 0.8090169943749474513 ) ) ;
#16320=VECTOR ( 'NONE', #9749, 1000.000000000000000 ) ;
#16324=VERTEX_POINT ( 'NONE', #15362 ) ;
#16325=ORIENTED_EDGE ( 'NONE', *, *, #8357, .T. ) ;
#16328=LINE ( 'NONE', #16, #27735 ) ;
#16330=DIRECTION ( 'NONE',  ( -2.698458740408365879E-16, 1.000000000000000000, 0.000000000000000000 ) ) ;
#16331=CARTESIAN_POINT ( 'NONE',  ( 175.7287565553229456, -4.999999999999970690, -22.10610323145030520 ) ) ;
#16332=ORIENTED_EDGE ( 'NONE', *, *, #5089, .T. ) ;
#16334=ORIENTED_EDGE ( 'NONE', *, *, #26256, .T. ) ;
#16336=ORIENTED_EDGE ( 'NONE', *, *, #26361, .F. ) ;
#16339=PLANE ( 'NONE',  #23791 ) ;
#16344=ADVANCED_FACE ( 'NONE', ( #22247 ), #12473, .T. ) ;
#16347=EDGE_CURVE ( 'NONE', #8301, #27211, #19792, .T. ) ;
#16348=EDGE_CURVE ( 'NONE', #5191, #27103, #14903, .T. ) ;
#16349=EDGE_LOOP ( 'NONE', ( #6455, #12539, #13570, #20995 ) ) ;
#16350=LINE ( 'NONE', #25981, #28923 ) ;
#16351=VECTOR ( 'NONE', #4964, 1000.000000000000000 ) ;
#16352=LINE ( 'NONE', #11770, #27727 ) ;
#16353=CARTESIAN_POINT ( 'NONE',  ( 168.6922820468853672, -9.999999999999996447, -26.58683881228715862 ) ) ;
#16354=LINE ( 'NONE', #13761, #15333 ) ;
#16355=AXIS2_PLACEMENT_3D ( 'NONE', #14594, #16601, #19041 ) ;
#16357=LINE ( 'NONE', #2954, #14113 ) ;
#16358=ORIENTED_EDGE ( 'NONE', *, *, #14203, .F. ) ;
#16359=CARTESIAN_POINT ( 'NONE',  ( 175.7287565553229456, -4.999999999999969802, -13.44584919360591257 ) ) ;
#16360=ORIENTED_EDGE ( 'NONE', *, *, #16445, .T. ) ;
#16361=VECTOR ( 'NONE', #4485, 1000.000000000000000 ) ;
#16363=ORIENTED_EDGE ( 'NONE', *, *, #7736, .F. ) ;
#16364=VECTOR ( 'NONE', #23972, 1000.000000000000000 ) ;
#16366=DIRECTION ( 'NONE',  ( -2.698458740408365879E-16, 1.000000000000000000, 0.000000000000000000 ) ) ;
#16369=ORIENTED_EDGE ( 'NONE', *, *, #12802, .T. ) ;
#16370=DIRECTION ( 'NONE',  ( -0.5877852522924731371, -1.586114251531760235E-16, 0.8090169943749474513 ) ) ;
#16372=EDGE_CURVE ( 'NONE', #18739, #2712, #1059, .T. ) ;
#16373=VECTOR ( 'NONE', #9969, 1000.000000000000000 ) ;
#16376=CARTESIAN_POINT ( 'NONE',  ( 171.1922820468853104, -1.999999999999970912, -13.59645775552055902 ) ) ;
#16378=ORIENTED_EDGE ( 'NONE', *, *, #19646, .T. ) ;
#16379=DIRECTION ( 'NONE',  ( 0.3090169943749472292, 8.338696094057992503E-17, -0.9510565162951536422 ) ) ;
#16383=AXIS2_PLACEMENT_3D ( 'NONE', #12740, #17766, #10602 ) ;
#16385=EDGE_CURVE ( 'NONE', #29420, #22008, #17216, .T. ) ;
#16386=ORIENTED_EDGE ( 'NONE', *, *, #6642, .F. ) ;
#16387=EDGE_CURVE ( 'NONE', #6140, #20355, #24394, .T. ) ;
#16388=ORIENTED_EDGE ( 'NONE', *, *, #25246, .F. ) ;
#16391=VECTOR ( 'NONE', #21678, 1000.000000000000000 ) ;
#16392=PLANE ( 'NONE',  #26024 ) ;
#16393=CARTESIAN_POINT ( 'NONE',  ( 154.7287565553230309, -4.999999999999975131, -33.82050807568879947 ) ) ;
#16395=CARTESIAN_POINT ( 'NONE',  ( 144.7287565553230309, -1.999999999999977129, -16.50000000000000355 ) ) ;
#16403=CARTESIAN_POINT ( 'NONE',  ( 2.407616245347821593, -5.000000000000016875, 7.409880882142680036 ) ) ;
#16404=CARTESIAN_POINT ( 'NONE',  ( 152.0152310637604955, -10.00000000000000178, 1.702185954127501066 ) ) ;
#16405=CARTESIAN_POINT ( 'NONE',  ( 149.5152310637605524, -10.00000000000000178, -11.28819510263909542 ) ) ;
#16407=VERTEX_POINT ( 'NONE', #10336 ) ;
#16408=CARTESIAN_POINT ( 'NONE',  ( 129.5152310637605808, -10.00000000000000888, -19.94844914048349338 ) ) ;
#16410=EDGE_CURVE ( 'NONE', #16190, #11956, #1356, .T. ) ;
#16411=VERTEX_POINT ( 'NONE', #29011 ) ;
#16412=VECTOR ( 'NONE', #3998, 1000.000000000000000 ) ;
#16414=FACE_OUTER_BOUND ( 'NONE', #17885, .T. ) ;
#16416=VECTOR ( 'NONE', #20590, 1000.000000000000000 ) ;
#16421=VECTOR ( 'NONE', #7986, 1000.000000000000000 ) ;
#16424=ORIENTED_EDGE ( 'NONE', *, *, #823, .T. ) ;
#16428=DIRECTION ( 'NONE',  ( 0.3090169943749475623, 8.338696094058001131E-17, 0.9510565162951536422 ) ) ;
#16430=ORIENTED_EDGE ( 'NONE', *, *, #24105, .T. ) ;
#16431=DIRECTION ( 'NONE',  ( -0.8090169943749474513, -2.183098979609982436E-16, -0.5877852522924731371 ) ) ;
#16432=CARTESIAN_POINT ( 'NONE',  ( 171.1922820468852819, -9.999999999999996447, -4.936203717676158398 ) ) ;
#16435=ORIENTED_EDGE ( 'NONE', *, *, #16410, .F. ) ;
#16436=FACE_OUTER_BOUND ( 'NONE', #24238, .T. ) ;
#16439=LINE ( 'NONE', #9411, #11175 ) ;
#16441=ADVANCED_FACE ( 'NONE', ( #10187 ), #15057, .T. ) ;
#16443=ORIENTED_EDGE ( 'NONE', *, *, #11755, .T. ) ;
#16445=EDGE_CURVE ( 'NONE', #15239, #2318, #8198, .T. ) ;
#16448=EDGE_CURVE ( 'NONE', #29689, #27920, #15215, .T. ) ;
#16459=PLANE ( 'NONE',  #24013 ) ;
#16461=VECTOR ( 'NONE', #25644, 1000.000000000000000 ) ;
#16462=CARTESIAN_POINT ( 'NONE',  ( 177.2287565553229172, -1.999999999999968026, -29.49038105676660493 ) ) ;
#16467=VECTOR ( 'NONE', #23179, 1000.000000000000000 ) ;
#16468=ORIENTED_EDGE ( 'NONE', *, *, #6826, .T. ) ;
#16470=ORIENTED_EDGE ( 'NONE', *, *, #25580, .F. ) ;
#16471=LINE ( 'NONE', #7329, #16320 ) ;
#16474=CARTESIAN_POINT ( 'NONE',  ( 149.5152310637605524, -1.999999999999976241, -11.28819510263909542 ) ) ;
#16475=ORIENTED_EDGE ( 'NONE', *, *, #28801, .F. ) ;
#16476=VECTOR ( 'NONE', #25792, 1000.000000000000000 ) ;
#16477=ORIENTED_EDGE ( 'NONE', *, *, #25146, .T. ) ;
#16479=CARTESIAN_POINT ( 'NONE',  ( 144.5152310637606092, -10.00000000000000178, -19.94844914048349693 ) ) ;
#16480=EDGE_CURVE ( 'NONE', #18591, #8784, #28708, .T. ) ;
#16482=DIRECTION ( 'NONE',  ( 0.3090169943749472292, 8.338696094057992503E-17, -0.9510565162951536422 ) ) ;
#16483=PLANE ( 'NONE',  #7677 ) ;
#16484=EDGE_CURVE ( 'NONE', #16977, #8387, #25297, .T. ) ;
#16485=EDGE_LOOP ( 'NONE', ( #2355, #17969, #9802, #21534 ) ) ;
#16486=FACE_OUTER_BOUND ( 'NONE', #166, .T. ) ;
#16487=ORIENTED_EDGE ( 'NONE', *, *, #23729, .F. ) ;
#16492=ORIENTED_EDGE ( 'NONE', *, *, #4323, .F. ) ;
#16493=ORIENTED_EDGE ( 'NONE', *, *, #18555, .F. ) ;
#16494=VECTOR ( 'NONE', #5648, 1000.000000000000000 ) ;
#16495=DIRECTION ( 'NONE',  ( 0.9510565162951536422, 0.000000000000000000, -0.3090169943749475623 ) ) ;
#16496=FACE_OUTER_BOUND ( 'NONE', #9753, .T. ) ;
#16498=CIRCLE ( 'NONE', #3355, 8.000000000000007105 ) ;
#16500=VECTOR ( 'NONE', #29703, 1000.000000000000000 ) ;
#16501=VERTEX_POINT ( 'NONE', #10799 ) ;
#16502=FACE_OUTER_BOUND ( 'NONE', #10198, .T. ) ;
#16503=AXIS2_PLACEMENT_3D ( 'NONE', #25942, #18232, #8916 ) ;
#16504=ORIENTED_EDGE ( 'NONE', *, *, #24814, .T. ) ;
#16505=FACE_OUTER_BOUND ( 'NONE', #6663, .T. ) ;
#16507=LINE ( 'NONE', #3101, #22170 ) ;
#16510=DIRECTION ( 'NONE',  ( 0.5877852522924731371, 1.586114251531760728E-16, 0.8090169943749474513 ) ) ;
#16512=VECTOR ( 'NONE', #25075, 1000.000000000000000 ) ;
#16513=DIRECTION ( 'NONE',  ( -2.698458740408365879E-16, 1.000000000000000000, 0.000000000000000000 ) ) ;
#16514=VERTEX_POINT ( 'NONE', #25006 ) ;
#16516=ORIENTED_EDGE ( 'NONE', *, *, #11031, .F. ) ;
#16517=EDGE_CURVE ( 'NONE', #25397, #9138, #6226, .T. ) ;
#16518=EDGE_CURVE ( 'NONE', #6555, #30249, #20550, .T. ) ;
#16521=DIRECTION ( 'NONE',  ( -2.698458740408365879E-16, 1.000000000000000000, 0.000000000000000000 ) ) ;
#16522=CARTESIAN_POINT ( 'NONE',  ( 157.0152310637605240, -4.999999999999975131, -26.04193191628311155 ) ) ;
#16523=EDGE_CURVE ( 'NONE', #25751, #18805, #27166, .T. ) ;
#16526=VECTOR ( 'NONE', #2998, 1000.000000000000000 ) ;
#16527=ORIENTED_EDGE ( 'NONE', *, *, #17916, .F. ) ;
#16529=EDGE_CURVE ( 'NONE', #19537, #18724, #27473, .T. ) ;
#16531=ORIENTED_EDGE ( 'NONE', *, *, #28393, .F. ) ;
#16533=DIRECTION ( 'NONE',  ( 0.000000000000000000, -1.000000000000000000, 0.000000000000000000 ) ) ;
#16536=ORIENTED_EDGE ( 'NONE', *, *, #16480, .F. ) ;
#16537=FACE_OUTER_BOUND ( 'NONE', #2844, .T. ) ;
#16541=ORIENTED_EDGE ( 'NONE', *, *, #4274, .F. ) ;
#16542=ORIENTED_EDGE ( 'NONE', *, *, #12623, .F. ) ;
#16543=ORIENTED_EDGE ( 'NONE', *, *, #20161, .F. ) ;
#16546=VECTOR ( 'NONE', #23230, 1000.000000000000000 ) ;
#16549=EDGE_CURVE ( 'NONE', #29920, #29503, #1662, .T. ) ;
#16557=CARTESIAN_POINT ( 'NONE',  ( 158.6922820468854241, -4.999999999999975131, -35.24709285013155835 ) ) ;
#16558=CARTESIAN_POINT ( 'NONE',  ( 166.1922820468853104, -1.999999999999972689, -4.936203717676158398 ) ) ;
#16560=CARTESIAN_POINT ( 'NONE',  ( 172.0152310637604955, -9.999999999999994671, -24.27857615940569502 ) ) ;
#16562=ORIENTED_EDGE ( 'NONE', *, *, #18980, .F. ) ;
#16564=CARTESIAN_POINT ( 'NONE',  ( 163.6922820468852819, -9.999999999999998224, 2.247092850131519715 ) ) ;
#16565=EDGE_CURVE ( 'NONE', #8011, #6528, #22406, .T. ) ;
#16568=AXIS2_PLACEMENT_3D ( 'NONE', #16142, #11547, #25165 ) ;
#16569=CYLINDRICAL_SURFACE ( 'NONE', #6155, 8.000000000000007105 ) ;
#16574=ORIENTED_EDGE ( 'NONE', *, *, #11576, .T. ) ;
#16578=EDGE_LOOP ( 'NONE', ( #4851, #15299, #5978, #4076 ) ) ;
#16580=VECTOR ( 'NONE', #19253, 1000.000000000000000 ) ;
#16581=ORIENTED_EDGE ( 'NONE', *, *, #26747, .T. ) ;
#16582=LINE ( 'NONE', #2570, #16216 ) ;
#16584=DIRECTION ( 'NONE',  ( 0.9510565162951535312, 2.566386769018988816E-16, -0.3090169943749475623 ) ) ;
#16585=ORIENTED_EDGE ( 'NONE', *, *, #18689, .T. ) ;
#16586=VECTOR ( 'NONE', #13346, 999.9999999999998863 ) ;
#16587=CARTESIAN_POINT ( 'NONE',  ( 23.16277852942019067, -5.000000000000011546, -71.28770215523300635 ) ) ;
#16588=LINE ( 'NONE', #16884, #15094 ) ;
#16593=LINE ( 'NONE', #718, #9004 ) ;
#16595=LINE ( 'NONE', #12308, #26837 ) ;
#16596=PLANE ( 'NONE',  #14391 ) ;
#16597=AXIS2_PLACEMENT_3D ( 'NONE', #14595, #11860, #2585 ) ;
#16598=ORIENTED_EDGE ( 'NONE', *, *, #28841, .F. ) ;
#16600=VECTOR ( 'NONE', #23207, 999.9999999999998863 ) ;
#16601=DIRECTION ( 'NONE',  ( -0.8090169943749474513, -2.183098979609982436E-16, 0.5877852522924731371 ) ) ;
#16607=VECTOR ( 'NONE', #28877, 1000.000000000000000 ) ;
#16610=CARTESIAN_POINT ( 'NONE',  ( 97.54326518300754856, -4.999999999999991118, 70.86933047595960034 ) ) ;
#16612=CARTESIAN_POINT ( 'NONE',  ( 7.419037233917861407, -5.000000000000015987, 22.83344875651922123 ) ) ;
#16614=CARTESIAN_POINT ( 'NONE',  ( 146.1922820468854525, -10.00000000000000178, -22.25671179336496053 ) ) ;
#16617=ADVANCED_FACE ( 'NONE', ( #30079 ), #18110, .T. ) ;
#16618=DIRECTION ( 'NONE',  ( 2.908569913943826047E-16, -1.000000000000000000, 6.826925868028107924E-18 ) ) ;
#16619=EDGE_CURVE ( 'NONE', #14364, #10452, #15816, .T. ) ;
#16621=DIRECTION ( 'NONE',  ( -2.698458740408365879E-16, 1.000000000000000000, 0.000000000000000000 ) ) ;
#16623=PLANE ( 'NONE',  #16503 ) ;
#16625=ORIENTED_EDGE ( 'NONE', *, *, #2896, .T. ) ;
#16627=VERTEX_POINT ( 'NONE', #22859 ) ;
#16628=LINE ( 'NONE', #19209, #22187 ) ;
#16631=DIRECTION ( 'NONE',  ( -1.000000000000000000, -2.908569913943825554E-16, 0.000000000000000000 ) ) ;
#16632=ORIENTED_EDGE ( 'NONE', *, *, #15931, .T. ) ;
#16634=VERTEX_POINT ( 'NONE', #6676 ) ;
#16635=ORIENTED_EDGE ( 'NONE', *, *, #16267, .T. ) ;
#16637=CARTESIAN_POINT ( 'NONE',  ( 21.09505124120717667, -5.000000000000011546, -64.92389192093176575 ) ) ;
#16639=CARTESIAN_POINT ( 'NONE',  ( 152.0152310637605524, -1.999999999999974909, -26.04193191628311155 ) ) ;
#16640=ORIENTED_EDGE ( 'NONE', *, *, #3444, .T. ) ;
#16641=CARTESIAN_POINT ( 'NONE',  ( 148.6922820468854241, -1.999999999999976685, -17.92658477444275889 ) ) ;
#16644=VECTOR ( 'NONE', #30057, 1000.000000000000000 ) ;
#16645=ORIENTED_EDGE ( 'NONE', *, *, #27323, .F. ) ;
#16650=EDGE_LOOP ( 'NONE', ( #15320, #16386, #29603, #28835 ) ) ;
#16651=CARTESIAN_POINT ( 'NONE',  ( 166.1922820468853672, -9.999999999999998224, -19.40354224447947828 ) ) ;
#16652=VERTEX_POINT ( 'NONE', #17804 ) ;
#16656=ORIENTED_EDGE ( 'NONE', *, *, #14988, .T. ) ;
#16657=FACE_BOUND ( 'NONE', #19907, .T. ) ;
#16658=EDGE_CURVE ( 'NONE', #15913, #12566, #1961, .T. ) ;
#16662=VECTOR ( 'NONE', #9033, 1000.000000000000000 ) ;
#16663=DIRECTION ( 'NONE',  ( 0.000000000000000000, 0.000000000000000000, 1.000000000000000000 ) ) ;
#16664=CARTESIAN_POINT ( 'NONE',  ( 152.0152310637604955, -1.999999999999976241, 1.702185954127501066 ) ) ;
#16667=LINE ( 'NONE', #7510, #4127 ) ;
#16669=DIRECTION ( 'NONE',  ( -0.9510565162951536422, -2.566386769018988816E-16, -0.3090169943749472292 ) ) ;
#16670=ORIENTED_EDGE ( 'NONE', *, *, #7774, .F. ) ;
#16672=EDGE_LOOP ( 'NONE', ( #168, #6972, #4082, #16037, #24590 ) ) ;
#16675=LINE ( 'NONE', #28468, #28832 ) ;
#16679=DIRECTION ( 'NONE',  ( 0.9510565162951535312, 2.566386769018988816E-16, -0.3090169943749475623 ) ) ;
#16684=CARTESIAN_POINT ( 'NONE',  ( 142.0152310637606092, -10.00000000000000355, -32.93883019725009120 ) ) ;
#16685=VECTOR ( 'NONE', #22742, 1000.000000000000000 ) ;
#16689=LINE ( 'NONE', #23565, #19818 ) ;
#16690=EDGE_CURVE ( 'NONE', #12383, #16269, #29635, .T. ) ;
#16696=ORIENTED_EDGE ( 'NONE', *, *, #19061, .F. ) ;
#16697=CARTESIAN_POINT ( 'NONE',  ( 134.5152310637605524, -1.999999999999980460, -21.71180489736090991 ) ) ;
#16699=EDGE_CURVE ( 'NONE', #17686, #2910, #4532, .T. ) ;
#16701=EDGE_CURVE ( 'NONE', #28698, #209, #7685, .T. ) ;
#16702=ADVANCED_FACE ( 'NONE', ( #672 ), #10115, .T. ) ;
#16703=CARTESIAN_POINT ( 'NONE',  ( 175.7287565553229456, -9.999999999999971578, -33.50000000000000000 ) ) ;
#16704=EDGE_CURVE ( 'NONE', #5689, #1554, #21423, .T. ) ;
#16705=FACE_OUTER_BOUND ( 'NONE', #17317, .T. ) ;
#16706=CARTESIAN_POINT ( 'NONE',  ( 157.0152310637605240, -9.999999999999998224, -26.04193191628311155 ) ) ;
#16708=AXIS2_PLACEMENT_3D ( 'NONE', #5402, #28631, #2823 ) ;
#16715=FACE_OUTER_BOUND ( 'NONE', #4654, .T. ) ;
#16716=DIRECTION ( 'NONE',  ( -0.5877852522924731371, -1.586114251531760235E-16, 0.8090169943749474513 ) ) ;
#16719=ORIENTED_EDGE ( 'NONE', *, *, #30194, .T. ) ;
#16720=CARTESIAN_POINT ( 'NONE',  ( 82.33896265977239182, -4.999999999999994671, 59.82275808417004015 ) ) ;
#16723=CARTESIAN_POINT ( 'NONE',  ( 164.7287565553229740, -4.999999999999972466, -33.82050807568879947 ) ) ;
#16726=ORIENTED_EDGE ( 'NONE', *, *, #29988, .T. ) ;
#16731=VECTOR ( 'NONE', #23799, 1000.000000000000000 ) ;
#16733=EDGE_CURVE ( 'NONE', #11366, #9707, #28487, .T. ) ;
#16734=ORIENTED_EDGE ( 'NONE', *, *, #23958, .F. ) ;
#16735=VERTEX_POINT ( 'NONE', #16121 ) ;
#16738=EDGE_CURVE ( 'NONE', #9954, #11059, #21714, .T. ) ;
#16739=DIRECTION ( 'NONE',  ( -2.698458740408365879E-16, 1.000000000000000000, 0.000000000000000000 ) ) ;
#16740=FACE_OUTER_BOUND ( 'NONE', #11664, .T. ) ;
#16741=ORIENTED_EDGE ( 'NONE', *, *, #9965, .T. ) ;
#16744=SHAPE_REPRESENTATION ( 'Ergonomic Serrated Toe Peg', ( #13190 ), #7783 ) ;
#16747=LINE ( 'NONE', #2578, #26359 ) ;
#16748=LINE ( 'NONE', #582, #19726 ) ;
#16751=LINE ( 'NONE', #21781, #30076 ) ;
#16752=EDGE_LOOP ( 'NONE', ( #30219, #1154, #20916, #7430 ) ) ;
#16754=CARTESIAN_POINT ( 'NONE',  ( 151.1922820468853956, -1.999999999999976241, -10.74328820663507678 ) ) ;
#16755=ORIENTED_EDGE ( 'NONE', *, *, #11615, .T. ) ;
#16756=DIRECTION ( 'NONE',  ( -2.698458740408365879E-16, 1.000000000000000000, 0.000000000000000000 ) ) ;
#16759=EDGE_CURVE ( 'NONE', #23759, #23604, #28791, .T. ) ;
#16761=ORIENTED_EDGE ( 'NONE', *, *, #22631, .T. ) ;
#16765=CARTESIAN_POINT ( 'NONE',  ( 166.1922820468853672, -1.999999999999971800, -22.25671179336496053 ) ) ;
#16766=VECTOR ( 'NONE', #6878, 1000.000000000000000 ) ;
#16767=DIRECTION ( 'NONE',  ( 0.9510565162951536422, 2.566386769018988816E-16, 0.3090169943749472292 ) ) ;
#16770=CARTESIAN_POINT ( 'NONE',  ( 171.1922820468853672, -4.999999999999970690, -28.06379628232387802 ) ) ;
#16771=CARTESIAN_POINT ( 'NONE',  ( 176.1922820468853104, -9.999999999999994671, -19.40354224447947828 ) ) ;
#16772=CARTESIAN_POINT ( 'NONE',  ( 22.68532101535755885, -5.000000000000011546, -69.81823902450180697 ) ) ;
#16774=LINE ( 'NONE', #26098, #18951 ) ;
#16776=ORIENTED_EDGE ( 'NONE', *, *, #3148, .F. ) ;
#16781=DIRECTION ( 'NONE',  ( -1.110223024625156540E-16, 0.000000000000000000, -1.000000000000000000 ) ) ;
#16782=ORIENTED_EDGE ( 'NONE', *, *, #2114, .F. ) ;
#16785=AXIS2_PLACEMENT_3D ( 'NONE', #9702, #10159, #26517 ) ;
#16787=CARTESIAN_POINT ( 'NONE',  ( 161.1922820468853672, -1.999999999999973133, -22.25671179336496053 ) ) ;
#16788=EDGE_LOOP ( 'NONE', ( #2607, #22027, #1431, #29374 ) ) ;
#16789=CARTESIAN_POINT ( 'NONE',  ( 169.7287565553229172, -1.999999999999970468, -16.50000000000000355 ) ) ;
#16797=EDGE_CURVE ( 'NONE', #5129, #26933, #534, .T. ) ;
#16798=PLANE ( 'NONE',  #30183 ) ;
#16802=FACE_BOUND ( 'NONE', #13707, .T. ) ;
#16803=VECTOR ( 'NONE', #4763, 1000.000000000000000 ) ;
#16806=LINE ( 'NONE', #28156, #1437 ) ;
#16807=ORIENTED_EDGE ( 'NONE', *, *, #2179, .F. ) ;
#16808=CARTESIAN_POINT ( 'NONE',  ( 10.84018844833751594, -5.000000000000015099, 33.36266952732570701 ) ) ;
#16811=VERTEX_POINT ( 'NONE', #7835 ) ;
#16812=CARTESIAN_POINT ( 'NONE',  ( 139.5152310637605808, -1.999999999999978684, -21.71180489736090991 ) ) ;
#16813=ORIENTED_EDGE ( 'NONE', *, *, #5294, .F. ) ;
#16817=CARTESIAN_POINT ( 'NONE',  ( 137.0152310637606092, -1.999999999999979572, -6.958068083716895558 ) ) ;
#16818=CARTESIAN_POINT ( 'NONE',  ( 159.5152310637604955, -9.999999999999998224, -11.28819510263909542 ) ) ;
#16819=ORIENTED_EDGE ( 'NONE', *, *, #270, .F. ) ;
#16821=ORIENTED_EDGE ( 'NONE', *, *, #30194, .F. ) ;
#16822=DIRECTION ( 'NONE',  ( -0.9510565162951536422, 0.000000000000000000, -0.3090169943749472292 ) ) ;
#16825=VERTEX_POINT ( 'NONE', #23147 ) ;
#16829=EDGE_CURVE ( 'NONE', #23355, #22122, #20844, .T. ) ;
#16830=VECTOR ( 'NONE', #3386, 1000.000000000000000 ) ;
#16831=CARTESIAN_POINT ( 'NONE',  ( 174.5152310637603819, -9.999999999999994671, -4.391296821672111328 ) ) ;
#16833=EDGE_CURVE ( 'NONE', #27200, #22368, #21575, .T. ) ;
#16836=DIRECTION ( 'NONE',  ( -0.8090169943749474513, -2.183098979609982436E-16, -0.5877852522924731371 ) ) ;
#16839=ORIENTED_EDGE ( 'NONE', *, *, #20441, .F. ) ;
#16840=DIRECTION ( 'NONE',  ( -2.698458740408365879E-16, 1.000000000000000000, 0.000000000000000000 ) ) ;
#16841=EDGE_LOOP ( 'NONE', ( #22676, #12055, #23926, #2069 ) ) ;
#16842=EDGE_LOOP ( 'NONE', ( #16017, #13608, #14692, #19364 ) ) ;
#16843=VECTOR ( 'NONE', #6657, 1000.000000000000000 ) ;
#16844=DIRECTION ( 'NONE',  ( 0.5877852522924731371, 1.586114251531760728E-16, 0.8090169943749474513 ) ) ;
#16846=CARTESIAN_POINT ( 'NONE',  ( 149.5152310637605524, -1.999999999999976241, -11.28819510263909542 ) ) ;
#16847=DIRECTION ( 'NONE',  ( -2.698458740408365879E-16, 1.000000000000000000, 0.000000000000000000 ) ) ;
#16848=CARTESIAN_POINT ( 'NONE',  ( 175.7287565553229456, -9.999999999999971578, 3.500000000000003109 ) ) ;
#16850=CARTESIAN_POINT ( 'NONE',  ( 176.1922820468852819, -9.999999999999994671, -10.74328820663507678 ) ) ;
#16856=ORIENTED_EDGE ( 'NONE', *, *, #25973, .F. ) ;
#16857=LINE ( 'NONE', #26185, #20733 ) ;
#16859=DIRECTION ( 'NONE',  ( -2.698458740408365879E-16, 1.000000000000000000, -0.000000000000000000 ) ) ;
#16862=LINE ( 'NONE', #14107, #12969 ) ;
#16864=DIRECTION ( 'NONE',  ( -1.000000000000000000, 0.000000000000000000, 0.000000000000000000 ) ) ;
#16866=ADVANCED_FACE ( 'NONE', ( #7397 ), #16912, .T. ) ;
#16867=VECTOR ( 'NONE', #6665, 1000.000000000000000 ) ;
#16869=EDGE_CURVE ( 'NONE', #10367, #29995, #7908, .T. ) ;
#16870=EDGE_CURVE ( 'NONE', #2694, #10208, #5779, .T. ) ;
#16881=CARTESIAN_POINT ( 'NONE',  ( 133.7287565553229172, -1.999999999999988010, -33.50000000000000000 ) ) ;
#16882=CARTESIAN_POINT ( 'NONE',  ( 153.6922820468853388, -1.999999999999975353, -15.07341522555727309 ) ) ;
#16884=CARTESIAN_POINT ( 'NONE',  ( 175.7287565553229456, -9.999999999999971578, 3.500000000000003109 ) ) ;
#16886=AXIS2_PLACEMENT_3D ( 'NONE', #19258, #5078, #16822 ) ;
#16890=CARTESIAN_POINT ( 'NONE',  ( 133.6922820468854241, -1.999999999999981348, -0.6060766987539614181 ) ) ;
#16893=CARTESIAN_POINT ( 'NONE',  ( 172.0152310637604103, -9.999999999999996447, -8.721423840594312082 ) ) ;
#16894=VERTEX_POINT ( 'NONE', #10188 ) ;
#16896=EDGE_CURVE ( 'NONE', #2945, #28540, #2899, .T. ) ;
#16897=EDGE_CURVE ( 'NONE', #6558, #8041, #5170, .T. ) ;
#16898=DIRECTION ( 'NONE',  ( -0.9510565162951536422, -2.566386769018988323E-16, 0.3090169943749475623 ) ) ;
#16899=VERTEX_POINT ( 'NONE', #19053 ) ;
#16900=EDGE_CURVE ( 'NONE', #4823, #23552, #5626, .T. ) ;
#16901=EDGE_LOOP ( 'NONE', ( #9616, #3945, #26704, #8066 ) ) ;
#16902=EDGE_CURVE ( 'NONE', #17958, #10367, #7757, .T. ) ;
#16907=LINE ( 'NONE', #3490, #10639 ) ;
#16908=CARTESIAN_POINT ( 'NONE',  ( 132.0152310637605808, -10.00000000000000711, -15.61832212156129351 ) ) ;
#16910=VECTOR ( 'NONE', #10059, 1000.000000000000000 ) ;
#16911=EDGE_LOOP ( 'NONE', ( #27671, #24967, #8250, #13669 ) ) ;
#16912=PLANE ( 'NONE',  #6469 ) ;
#16914=CARTESIAN_POINT ( 'NONE',  ( 164.7287565553229172, -4.999999999999973355, -16.50000000000000000 ) ) ;
#16915=DIRECTION ( 'NONE',  ( 0.5877852522924731371, 1.586114251531760728E-16, 0.8090169943749474513 ) ) ;
#16916=DIRECTION ( 'NONE',  ( -2.698458740408365879E-16, 1.000000000000000000, 0.000000000000000000 ) ) ;
#16918=EDGE_CURVE ( 'NONE', #5616, #18859, #29014, .T. ) ;
#16919=PLANE ( 'NONE',  #20875 ) ;
#16921=ORIENTED_EDGE ( 'NONE', *, *, #21862, .T. ) ;
#16923=LINE ( 'NONE', #9899, #18280 ) ;
#16924=VECTOR ( 'NONE', #29507, 1000.000000000000000 ) ;
#16927=FACE_BOUND ( 'NONE', #15805, .T. ) ;
#16928=VERTEX_POINT ( 'NONE', #14906 ) ;
#16929=ORIENTED_EDGE ( 'NONE', *, *, #11687, .T. ) ;
#16930=AXIS2_PLACEMENT_3D ( 'NONE', #369, #7525, #21566 ) ;
#16932=DIRECTION ( 'NONE',  ( -0.5877852522924731371, 0.000000000000000000, 0.8090169943749474513 ) ) ;
#16934=CARTESIAN_POINT ( 'NONE',  ( 171.1922820468853672, -9.999999999999994671, -30.91696583120936026 ) ) ;
#16935=EDGE_LOOP ( 'NONE', ( #7443, #15176, #9826, #28772 ) ) ;
#16936=EDGE_CURVE ( 'NONE', #14997, #19874, #24250, .T. ) ;
#16937=FACE_OUTER_BOUND ( 'NONE', #15098, .T. ) ;
#16938=ORIENTED_EDGE ( 'NONE', *, *, #25610, .F. ) ;
#16939=EDGE_CURVE ( 'NONE', #4559, #27662, #28554, .T. ) ;
#16941=ORIENTED_EDGE ( 'NONE', *, *, #6263, .T. ) ;
#16942=VECTOR ( 'NONE', #788, 1000.000000000000000 ) ;
#16946=VERTEX_POINT ( 'NONE', #601 ) ;
#16947=CARTESIAN_POINT ( 'NONE',  ( 130.7287565553229172, -4.999999999999983125, -30.76635726929465875 ) ) ;
#16948=VERTEX_POINT ( 'NONE', #24398 ) ;
#16954=ORIENTED_EDGE ( 'NONE', *, *, #8271, .T. ) ;
#16956=FACE_BOUND ( 'NONE', #24569, .T. ) ;
#16957=VECTOR ( 'NONE', #5807, 1000.000000000000000 ) ;
#16958=VERTEX_POINT ( 'NONE', #9886 ) ;
#16959=EDGE_CURVE ( 'NONE', #26148, #4081, #3495, .T. ) ;
#16960=DIRECTION ( 'NONE',  ( 0.5877852522924731371, 0.000000000000000000, 0.8090169943749474513 ) ) ;
#16962=VECTOR ( 'NONE', #10532, 1000.000000000000000 ) ;
#16963=CARTESIAN_POINT ( 'NONE',  ( 162.0152310637604955, -9.999999999999998224, -15.61832212156129707 ) ) ;
#16964=CARTESIAN_POINT ( 'NONE',  ( 162.0152310637604387, -9.999999999999998224, -8.721423840594312082 ) ) ;
#16966=CARTESIAN_POINT ( 'NONE',  ( 151.1922820468853956, -4.999999999999976907, -13.59645775552055902 ) ) ;
#16967=VERTEX_POINT ( 'NONE', #7607 ) ;
#16968=CARTESIAN_POINT ( 'NONE',  ( 143.6922820468853956, -1.999999999999978684, -0.6060766987539614181 ) ) ;
#16969=ORIENTED_EDGE ( 'NONE', *, *, #19315, .T. ) ;
#16971=ORIENTED_EDGE ( 'NONE', *, *, #15971, .T. ) ;
#16974=DIRECTION ( 'NONE',  ( 0.9510565162951536422, 0.000000000000000000, -0.3090169943749475623 ) ) ;
#16976=DIRECTION ( 'NONE',  ( -0.9510565162951536422, -2.566386769018988816E-16, -0.3090169943749472292 ) ) ;
#16977=VERTEX_POINT ( 'NONE', #9736 ) ;
#16980=ORIENTED_EDGE ( 'NONE', *, *, #20240, .F. ) ;
#16981=VECTOR ( 'NONE', #932, 1000.000000000000000 ) ;
#16984=DIRECTION ( 'NONE',  ( -2.698458740408365879E-16, 1.000000000000000000, 0.000000000000000000 ) ) ;
#16986=ORIENTED_EDGE ( 'NONE', *, *, #19852, .T. ) ;
#16987=DIRECTION ( 'NONE',  ( -0.5877852522924731371, 0.000000000000000000, 0.8090169943749474513 ) ) ;
#16989=VECTOR ( 'NONE', #2908, 1000.000000000000000 ) ;
#16994=ORIENTED_EDGE ( 'NONE', *, *, #20511, .F. ) ;
#16995=EDGE_LOOP ( 'NONE', ( #9611, #13969, #1532, #4265 ) ) ;
#16996=DIRECTION ( 'NONE',  ( -2.698458740408365879E-16, 1.000000000000000000, 0.000000000000000000 ) ) ;
#16997=LINE ( 'NONE', #538, #27007 ) ;
#16998=EDGE_CURVE ( 'NONE', #1088, #19198, #3347, .T. ) ;
#16999=EDGE_CURVE ( 'NONE', #23759, #28590, #5322, .T. ) ;
#17001=VECTOR ( 'NONE', #29097, 1000.000000000000000 ) ;
#17004=CARTESIAN_POINT ( 'NONE',  ( 169.5152310637604671, -4.999999999999971578, -1.881997125516404380E-14 ) ) ;
#17005=EDGE_CURVE ( 'NONE', #28689, #3516, #12323, .T. ) ;
#17011=ORIENTED_EDGE ( 'NONE', *, *, #15789, .F. ) ;
#17013=DIRECTION ( 'NONE',  ( -0.8090169943749474513, -2.183098979609982436E-16, -0.5877852522924731371 ) ) ;
#17014=CARTESIAN_POINT ( 'NONE',  ( 134.5152310637605524, -1.999999999999980460, -13.05155085951650840 ) ) ;
#17017=CARTESIAN_POINT ( 'NONE',  ( 167.0152310637605524, -1.999999999999970468, -32.93883019725009120 ) ) ;
#17019=ORIENTED_EDGE ( 'NONE', *, *, #26018, .F. ) ;
#17020=CARTESIAN_POINT ( 'NONE',  ( 153.6922820468853672, -1.999999999999975797, -9.266330736598359152 ) ) ;
#17022=DIRECTION ( 'NONE',  ( 0.9510565162951535312, 2.566386769018988816E-16, -0.3090169943749475623 ) ) ;
#17026=ORIENTED_EDGE ( 'NONE', *, *, #12035, .T. ) ;
#17028=VECTOR ( 'NONE', #4616, 1000.000000000000000 ) ;
#17031=AXIS2_PLACEMENT_3D ( 'NONE', #23461, #28382, #7437 ) ;
#17032=EDGE_LOOP ( 'NONE', ( #494, #13738, #27832, #5224 ) ) ;
#17034=ORIENTED_EDGE ( 'NONE', *, *, #19173, .T. ) ;
#17035=ADVANCED_FACE ( 'NONE', ( #738 ), #10033, .T. ) ;
#17038=ADVANCED_FACE ( 'NONE', ( #3198 ), #12476, .T. ) ;
#17039=EDGE_CURVE ( 'NONE', #14997, #18781, #8200, .T. ) ;
#17041=EDGE_CURVE ( 'NONE', #14797, #2212, #17511, .T. ) ;
#17044=VECTOR ( 'NONE', #23353, 1000.000000000000000 ) ;
#17048=CARTESIAN_POINT ( 'NONE',  ( 79.91207320562929795, -4.999999999999995559, 58.05951968496736981 ) ) ;
#17050=CARTESIAN_POINT ( 'NONE',  ( 136.1922820468854241, -10.00000000000000533, -19.40354224447947473 ) ) ;
#17051=DIRECTION ( 'NONE',  ( -0.5877852522924731371, -1.586114251531760235E-16, 0.8090169943749474513 ) ) ;
#17052=VERTEX_POINT ( 'NONE', #10946 ) ;
#17053=CARTESIAN_POINT ( 'NONE',  ( 138.6922820468854525, -10.00000000000000533, -17.92658477444275533 ) ) ;
#17054=CARTESIAN_POINT ( 'NONE',  ( 149.5152310637606092, -4.999999999999976907, -28.60870317832789667 ) ) ;
#17058=ORIENTED_EDGE ( 'NONE', *, *, #6601, .F. ) ;
#17060=ORIENTED_EDGE ( 'NONE', *, *, #29864, .F. ) ;
#17063=DIRECTION ( 'NONE',  ( -0.8090169943749474513, -2.183098979609982436E-16, 0.5877852522924731371 ) ) ;
#17064=CARTESIAN_POINT ( 'NONE',  ( 174.5152310637604103, -9.999999999999994671, -2.627941064794695691 ) ) ;
#17065=DIRECTION ( 'NONE',  ( -2.698458740408365879E-16, 1.000000000000000000, 0.000000000000000000 ) ) ;
#17066=AXIS2_PLACEMENT_3D ( 'NONE', #17050, #15344, #8339 ) ;
#17067=DIRECTION ( 'NONE',  ( 0.5877852522924731371, 1.586114251531760728E-16, 0.8090169943749474513 ) ) ;
#17068=DIRECTION ( 'NONE',  ( 0.5877852522924731371, 0.000000000000000000, 0.8090169943749474513 ) ) ;
#17070=EDGE_CURVE ( 'NONE', #2926, #4706, #3637, .T. ) ;
#17071=CARTESIAN_POINT ( 'NONE',  ( 171.1922820468853672, -9.999999999999994671, -28.06379628232387802 ) ) ;
#17072=CARTESIAN_POINT ( 'NONE',  ( 127.1715206774213840, -4.999999999999983125, -92.39551812325976243 ) ) ;
#17073=EDGE_CURVE ( 'NONE', #29440, #12783, #15217, .T. ) ;
#17074=EDGE_CURVE ( 'NONE', #5150, #25448, #25147, .T. ) ;
#17076=VECTOR ( 'NONE', #28080, 1000.000000000000000 ) ;
#17079=ORIENTED_EDGE ( 'NONE', *, *, #26474, .T. ) ;
#17080=VECTOR ( 'NONE', #2202, 999.9999999999998863 ) ;
#17082=CARTESIAN_POINT ( 'NONE',  ( 96.02733224039648974, -4.999999999999991118, -69.76794072354836374 ) ) ;
#17085=FACE_BOUND ( 'NONE', #7419, .T. ) ;
#17086=VERTEX_POINT ( 'NONE', #26867 ) ;
#17088=CARTESIAN_POINT ( 'NONE',  ( 162.0152310637604671, -9.999999999999998224, -17.38167787843871182 ) ) ;
#17092=DIRECTION ( 'NONE',  ( -0.9510565162951536422, 0.000000000000000000, -0.3090169943749472292 ) ) ;
#17093=ORIENTED_EDGE ( 'NONE', *, *, #1661, .T. ) ;
#17095=ORIENTED_EDGE ( 'NONE', *, *, #9341, .T. ) ;
#17100=LINE ( 'NONE', #26427, #3048 ) ;
#17101=VECTOR ( 'NONE', #17195, 1000.000000000000000 ) ;
#17103=ORIENTED_EDGE ( 'NONE', *, *, #26527, .F. ) ;
#17105=AXIS2_PLACEMENT_3D ( 'NONE', #4296, #22922, #25647 ) ;
#17107=DIRECTION ( 'NONE',  ( -0.5877852522924731371, -1.586114251531760728E-16, -0.8090169943749474513 ) ) ;
#17109=ADVANCED_FACE ( 'NONE', ( #15365 ), #27022, .T. ) ;
#17110=ADVANCED_FACE ( 'NONE', ( #8508 ), #19797, .T. ) ;
#17112=FACE_OUTER_BOUND ( 'NONE', #12287, .T. ) ;
#17114=EDGE_LOOP ( 'NONE', ( #7676, #23916, #19900, #1524, #17477 ) ) ;
#17117=DIRECTION ( 'NONE',  ( 0.5877852522924731371, 0.000000000000000000, 0.8090169943749474513 ) ) ;
#17118=VECTOR ( 'NONE', #2683, 999.9999999999998863 ) ;
#17119=CARTESIAN_POINT ( 'NONE',  ( 6.385173589811359740, -5.000000000000015987, 19.65154363936862936 ) ) ;
#17120=ORIENTED_EDGE ( 'NONE', *, *, #9372, .T. ) ;
#17123=ORIENTED_EDGE ( 'NONE', *, *, #30222, .T. ) ;
#17125=DIRECTION ( 'NONE',  ( 0.9510565162951535312, 2.566386769018988816E-16, -0.3090169943749475623 ) ) ;
#17127=FACE_OUTER_BOUND ( 'NONE', #25851, .T. ) ;
#17128=VERTEX_POINT ( 'NONE', #27332 ) ;
#17129=DIRECTION ( 'NONE',  ( 0.3090169943749472292, 8.338696094057992503E-17, -0.9510565162951536422 ) ) ;
#17130=ORIENTED_EDGE ( 'NONE', *, *, #29204, .F. ) ;
#17135=ORIENTED_EDGE ( 'NONE', *, *, #21722, .T. ) ;
#17137=DIRECTION ( 'NONE',  ( 0.000000000000000000, 0.000000000000000000, -1.000000000000000000 ) ) ;
#17139=ORIENTED_EDGE ( 'NONE', *, *, #21094, .F. ) ;
#17141=EDGE_CURVE ( 'NONE', #29995, #20158, #22251, .T. ) ;
#17144=VERTEX_POINT ( 'NONE', #1359 ) ;
#17148=EDGE_CURVE ( 'NONE', #23355, #13222, #24706, .T. ) ;
#17149=PLANE ( 'NONE',  #15268 ) ;
#17151=DIRECTION ( 'NONE',  ( 0.9510565162951535312, 2.566386769018988816E-16, -0.3090169943749475623 ) ) ;
#17152=VECTOR ( 'NONE', #2668, 1000.000000000000000 ) ;
#17162=CARTESIAN_POINT ( 'NONE',  ( 142.2287565553230309, -1.999999999999978018, -20.83012701892220164 ) ) ;
#17165=EDGE_LOOP ( 'NONE', ( #26155, #8358, #23868, #17912, #8398 ) ) ;
#17166=VERTEX_POINT ( 'NONE', #13386 ) ;
#17169=CARTESIAN_POINT ( 'NONE',  ( 174.7287565553228887, -1.999999999999969358, -16.50000000000000355 ) ) ;
#17170=FACE_OUTER_BOUND ( 'NONE', #18783, .T. ) ;
#17171=ORIENTED_EDGE ( 'NONE', *, *, #11992, .F. ) ;
#17174=ORIENTED_EDGE ( 'NONE', *, *, #12511, .T. ) ;
#17177=ORIENTED_EDGE ( 'NONE', *, *, #28836, .F. ) ;
#17179=EDGE_CURVE ( 'NONE', #21366, #19068, #18113, .T. ) ;
#17180=VECTOR ( 'NONE', #7314, 1000.000000000000000 ) ;
#17182=EDGE_LOOP ( 'NONE', ( #5778, #1385, #3437, #1728 ) ) ;
#17185=VECTOR ( 'NONE', #8800, 1000.000000000000000 ) ;
#17186=PLANE ( 'NONE',  #14747 ) ;
#17187=ORIENTED_EDGE ( 'NONE', *, *, #17366, .T. ) ;
#17188=FACE_OUTER_BOUND ( 'NONE', #5081, .T. ) ;
#17190=DIRECTION ( 'NONE',  ( -1.110223024625156540E-16, 0.000000000000000000, -1.000000000000000000 ) ) ;
#17194=VECTOR ( 'NONE', #15105, 1000.000000000000000 ) ;
#17195=DIRECTION ( 'NONE',  ( 0.5877852522924731371, 1.586114251531760728E-16, 0.8090169943749474513 ) ) ;
#17196=DIRECTION ( 'NONE',  ( -0.5877852522924731371, 0.000000000000000000, 0.8090169943749474513 ) ) ;
#17199=CARTESIAN_POINT ( 'NONE',  ( 138.6922820468854525, -1.999999999999979128, -15.07341522555727309 ) ) ;
#17200=ORIENTED_EDGE ( 'NONE', *, *, #20775, .T. ) ;
#17201=LINE ( 'NONE', #21930, #8080 ) ;
#17202=LINE ( 'NONE', #12460, #24921 ) ;
#17203=CARTESIAN_POINT ( 'NONE',  ( 159.5152310637604955, -9.999999999999998224, -21.71180489736091346 ) ) ;
#17204=VECTOR ( 'NONE', #3795, 1000.000000000000000 ) ;
#17205=EDGE_LOOP ( 'NONE', ( #19946, #11767, #29793, #26110 ) ) ;
#17206=ORIENTED_EDGE ( 'NONE', *, *, #14822, .T. ) ;
#17207=VERTEX_POINT ( 'NONE', #8359 ) ;
#17211=EDGE_CURVE ( 'NONE', #22328, #23642, #24856, .T. ) ;
#17213=DIRECTION ( 'NONE',  ( 0.5877852522924731371, 1.586114251531760728E-16, -0.8090169943749474513 ) ) ;
#17214=CARTESIAN_POINT ( 'NONE',  ( 141.1922820468854241, -10.00000000000000533, -4.936203717676158398 ) ) ;
#17216=LINE ( 'NONE', #17660, #4030 ) ;
#17218=CARTESIAN_POINT ( 'NONE',  ( 167.0152310637605240, -4.999999999999972466, -1.854241549900776098E-14 ) ) ;
#17219=DIRECTION ( 'NONE',  ( -0.9510565162951536422, -2.566386769018988816E-16, -0.3090169943749472292 ) ) ;
#17220=CARTESIAN_POINT ( 'NONE',  ( 161.1922820468853104, -1.999999999999973577, -2.083034168790677043 ) ) ;
#17221=EDGE_LOOP ( 'NONE', ( #2188, #23391, #25586, #13427, #29556 ) ) ;
#17222=CARTESIAN_POINT ( 'NONE',  ( 133.6922820468854241, -10.00000000000000711, -17.92658477444275533 ) ) ;
#17223=CARTESIAN_POINT ( 'NONE',  ( 137.0152310637606092, -10.00000000000000533, -15.61832212156129351 ) ) ;
#17227=ORIENTED_EDGE ( 'NONE', *, *, #6947, .T. ) ;
#17231=FACE_BOUND ( 'NONE', #1475, .T. ) ;
#17232=EDGE_CURVE ( 'NONE', #17842, #2137, #8652, .T. ) ;
#17233=ORIENTED_EDGE ( 'NONE', *, *, #6410, .T. ) ;
#17234=LINE ( 'NONE', #14928, #6264 ) ;
#17236=CARTESIAN_POINT ( 'NONE',  ( 149.5152310637605240, -10.00000000000000178, -2.627941064794695691 ) ) ;
#17237=ORIENTED_EDGE ( 'NONE', *, *, #487, .F. ) ;
#17241=ORIENTED_EDGE ( 'NONE', *, *, #2859, .F. ) ;
#17246=EDGE_CURVE ( 'NONE', #29174, #11438, #1964, .T. ) ;
#17248=EDGE_CURVE ( 'NONE', #17495, #14294, #11390, .T. ) ;
#17249=ADVANCED_FACE ( 'NONE', ( #28229 ), #6682, .T. ) ;
#17254=CARTESIAN_POINT ( 'NONE',  ( 172.0152310637603819, -1.999999999999970912, -0.06116980274991495881 ) ) ;
#17255=DIRECTION ( 'NONE',  ( -1.110223024625156540E-16, 0.000000000000000000, -1.000000000000000000 ) ) ;
#17256=CARTESIAN_POINT ( 'NONE',  ( 169.7287565553229456, -1.999999999999970024, -25.16025403784440329 ) ) ;
#17258=LINE ( 'NONE', #7949, #29246 ) ;
#17259=CARTESIAN_POINT ( 'NONE',  ( 173.6922820468853388, -1.999999999999970468, -23.73366926340167282 ) ) ;
#17260=VECTOR ( 'NONE', #8172, 1000.000000000000000 ) ;
#17263=ORIENTED_EDGE ( 'NONE', *, *, #8325, .F. ) ;
#17264=CARTESIAN_POINT ( 'NONE',  ( 13.06581296851301310, -5.000000000000014211, 40.21243747300340488 ) ) ;
#17265=ORIENTED_EDGE ( 'NONE', *, *, #7571, .F. ) ;
#17267=ORIENTED_EDGE ( 'NONE', *, *, #5505, .T. ) ;
#17269=DIRECTION ( 'NONE',  ( -0.9510565162951536422, -2.566386769018988816E-16, -0.3090169943749472292 ) ) ;
#17273=DIRECTION ( 'NONE',  ( -0.9510565162951536422, -2.566386769018988816E-16, -0.3090169943749472292 ) ) ;
#17274=ORIENTED_EDGE ( 'NONE', *, *, #24186, .T. ) ;
#17278=ORIENTED_EDGE ( 'NONE', *, *, #27935, .F. ) ;
#17280=LINE ( 'NONE', #12849, #8170 ) ;
#17282=ADVANCED_FACE ( 'NONE', ( #25444 ), #2118, .T. ) ;
#17283=DIRECTION ( 'NONE',  ( -0.8090169943749474513, -2.183098979609982436E-16, -0.5877852522924731371 ) ) ;
#17284=ADVANCED_FACE ( 'NONE', ( #2416 ), #18572, .T. ) ;
#17290=ORIENTED_EDGE ( 'NONE', *, *, #16054, .F. ) ;
#17291=ORIENTED_EDGE ( 'NONE', *, *, #26650, .F. ) ;
#17292=DIRECTION ( 'NONE',  ( 0.3090169943749475623, 8.338696094058001131E-17, 0.9510565162951536422 ) ) ;
#17293=CARTESIAN_POINT ( 'NONE',  ( 16.95959666478115224, -5.000000000000013323, -52.19627145232931298 ) ) ;
#17300=ORIENTED_EDGE ( 'NONE', *, *, #680, .F. ) ;
#17301=CARTESIAN_POINT ( 'NONE',  ( 134.5152310637605808, -4.999999999999980460, -19.94844914048349338 ) ) ;
#17302=CARTESIAN_POINT ( 'NONE',  ( 157.0152310637604671, -10.00000000000000000, -8.721423840594312082 ) ) ;
#17304=DIRECTION ( 'NONE',  ( -1.110223024625156540E-16, 0.000000000000000000, -1.000000000000000000 ) ) ;
#17307=DIRECTION ( 'NONE',  ( 0.3090169943749472292, 8.338696094057992503E-17, -0.9510565162951536422 ) ) ;
#17309=EDGE_LOOP ( 'NONE', ( #14957, #15811, #14892, #25642 ) ) ;
#17315=CARTESIAN_POINT ( 'NONE',  ( 159.5152310637605240, -4.999999999999974243, -30.37205893520531319 ) ) ;
#17317=EDGE_LOOP ( 'NONE', ( #5108, #20652, #10323, #9649 ) ) ;
#17318=ADVANCED_FACE ( 'NONE', ( #23301 ), #23459, .T. ) ;
#17324=VECTOR ( 'NONE', #15043, 1000.000000000000000 ) ;
#17325=ORIENTED_EDGE ( 'NONE', *, *, #8071, .F. ) ;
#17327=CARTESIAN_POINT ( 'NONE',  ( 136.1922820468854241, -10.00000000000000533, -13.59645775552055547 ) ) ;
#17328=CARTESIAN_POINT ( 'NONE',  ( 129.5152310637605808, -10.00000000000000888, -11.28819510263909187 ) ) ;
#17329=LINE ( 'NONE', #5750, #12543 ) ;
#17330=CARTESIAN_POINT ( 'NONE',  ( 136.1922820468854241, -10.00000000000000533, -10.74328820663507322 ) ) ;
#17332=EDGE_CURVE ( 'NONE', #7083, #29062, #16582, .T. ) ;
#17335=AXIS2_PLACEMENT_3D ( 'NONE', #4696, #282, #28086 ) ;
#17339=PLANE ( 'NONE',  #1966 ) ;
#17341=ORIENTED_EDGE ( 'NONE', *, *, #16024, .T. ) ;
#17343=CARTESIAN_POINT ( 'NONE',  ( 174.5152310637603819, -4.999999999999970690, -1.937508276747661261E-14 ) ) ;
#17344=LINE ( 'NONE', #10325, #542 ) ;
#17346=CARTESIAN_POINT ( 'NONE',  ( 163.6922820468853104, -9.999999999999998224, -9.266330736598359152 ) ) ;
#17348=ORIENTED_EDGE ( 'NONE', *, *, #13486, .T. ) ;
#17350=EDGE_LOOP ( 'NONE', ( #23375, #2690, #726, #22091 ) ) ;
#17351=VECTOR ( 'NONE', #23119, 1000.000000000000000 ) ;
#17354=CARTESIAN_POINT ( 'NONE',  ( 139.5152310637606092, -1.999999999999978684, -11.28819510263909542 ) ) ;
#17355=CARTESIAN_POINT ( 'NONE',  ( 131.1922820468854241, -1.999999999999981792, -2.083034168790677043 ) ) ;
#17356=CARTESIAN_POINT ( 'NONE',  ( 149.7287565553230024, -10.00000000000000178, -16.50000000000000355 ) ) ;
#17357=AXIS2_PLACEMENT_3D ( 'NONE', #22355, #15471, #3891 ) ;
#17358=VERTEX_POINT ( 'NONE', #9547 ) ;
#17359=CARTESIAN_POINT ( 'NONE',  ( 139.5152310637605808, -10.00000000000000533, -2.627941064794695691 ) ) ;
#17360=LINE ( 'NONE', #10341, #28777 ) ;
#17361=VECTOR ( 'NONE', #4146, 1000.000000000000000 ) ;
#17362=DIRECTION ( 'NONE',  ( -2.698458740408365879E-16, 1.000000000000000000, 0.000000000000000000 ) ) ;
#17366=EDGE_CURVE ( 'NONE', #23763, #22699, #4240, .T. ) ;
#17368=ORIENTED_EDGE ( 'NONE', *, *, #24957, .F. ) ;
#17371=ADVANCED_FACE ( 'NONE', ( #22863 ), #30233, .T. ) ;
#17375=FACE_BOUND ( 'NONE', #14325, .T. ) ;
#17376=ORIENTED_EDGE ( 'NONE', *, *, #2681, .F. ) ;
#17377=CARTESIAN_POINT ( 'NONE',  ( 154.5152310637605240, -10.00000000000000000, -11.28819510263909542 ) ) ;
#17378=VECTOR ( 'NONE', #28938, 1000.000000000000000 ) ;
#17380=LINE ( 'NONE', #19666, #20816 ) ;
#17382=FACE_OUTER_BOUND ( 'NONE', #14371, .T. ) ;
#17383=EDGE_LOOP ( 'NONE', ( #1708, #8275, #18981, #21119 ) ) ;
#17385=ORIENTED_EDGE ( 'NONE', *, *, #6987, .F. ) ;
#17386=VECTOR ( 'NONE', #27354, 1000.000000000000000 ) ;
#17389=VECTOR ( 'NONE', #30248, 1000.000000000000000 ) ;
#17390=LINE ( 'NONE', #24427, #1396 ) ;
#17391=ORIENTED_EDGE ( 'NONE', *, *, #18418, .F. ) ;
#17394=VERTEX_POINT ( 'NONE', #20696 ) ;
#17395=DIRECTION ( 'NONE',  ( 0.3090169943749475623, 8.338696094058001131E-17, 0.9510565162951536422 ) ) ;
#17396=FACE_BOUND ( 'NONE', #1229, .T. ) ;
#17397=AXIS2_PLACEMENT_3D ( 'NONE', #12386, #5687, #12840 ) ;
#17399=ADVANCED_FACE ( 'NONE', ( #27773 ), #2263, .T. ) ;
#17402=AXIS2_PLACEMENT_3D ( 'NONE', #26310, #7236, #25698 ) ;
#17403=ORIENTED_EDGE ( 'NONE', *, *, #6915, .T. ) ;
#17404=EDGE_CURVE ( 'NONE', #26448, #12211, #9395, .T. ) ;
#17405=CARTESIAN_POINT ( 'NONE',  ( 14.57230909446801270, -5.000000000000013323, -44.84895579867345106 ) ) ;
#17407=ADVANCED_FACE ( 'NONE', ( #26512 ), #5288, .T. ) ;
#17409=CARTESIAN_POINT ( 'NONE',  ( 151.1922820468853956, -10.00000000000000178, -13.59645775552055902 ) ) ;
#17410=LINE ( 'NONE', #21692, #18300 ) ;
#17411=EDGE_LOOP ( 'NONE', ( #4590, #1701, #4284, #17792 ) ) ;
#17413=ORIENTED_EDGE ( 'NONE', *, *, #26567, .F. ) ;
#17415=CARTESIAN_POINT ( 'NONE',  ( 169.5152310637604955, -1.999999999999970468, -19.94844914048349693 ) ) ;
#17418=DIRECTION ( 'NONE',  ( 2.908569913943825554E-16, -1.000000000000000000, 0.000000000000000000 ) ) ;
#17419=ORIENTED_EDGE ( 'NONE', *, *, #16733, .F. ) ;
#17425=AXIS2_PLACEMENT_3D ( 'NONE', #16186, #14486, #11750 ) ;
#17426=CARTESIAN_POINT ( 'NONE',  ( 132.0152310637605524, -4.999999999999982236, -34.70218595412750773 ) ) ;
#17428=CARTESIAN_POINT ( 'NONE',  ( 158.6922820468853956, -1.999999999999974465, -23.73366926340167282 ) ) ;
#17432=VERTEX_POINT ( 'NONE', #19025 ) ;
#17433=ORIENTED_EDGE ( 'NONE', *, *, #23052, .T. ) ;
#17435=DIRECTION ( 'NONE',  ( 0.5877852522924731371, 1.586114251531760728E-16, -0.8090169943749474513 ) ) ;
#17437=LINE ( 'NONE', #20038, #18194 ) ;
#17438=CARTESIAN_POINT ( 'NONE',  ( 142.0152310637606092, -1.999999999999978018, -32.93883019725009120 ) ) ;
#17439=CARTESIAN_POINT ( 'NONE',  ( 157.0152310637604955, -10.00000000000000000, -6.958068083716895558 ) ) ;
#17440=EDGE_CURVE ( 'NONE', #13196, #3218, #23608, .T. ) ;
#17441=EDGE_CURVE ( 'NONE', #24401, #25168, #28380, .T. ) ;
#17442=CARTESIAN_POINT ( 'NONE',  ( 141.1922820468854525, -10.00000000000000533, -28.06379628232387446 ) ) ;
#17443=VECTOR ( 'NONE', #11217, 1000.000000000000000 ) ;
#17446=EDGE_CURVE ( 'NONE', #23239, #16280, #7436, .T. ) ;
#17449=ORIENTED_EDGE ( 'NONE', *, *, #4362, .T. ) ;
#17450=CARTESIAN_POINT ( 'NONE',  ( 137.0152310637605808, -10.00000000000000533, 1.702185954127501066 ) ) ;
#17452=DIRECTION ( 'NONE',  ( 1.000000000000000000, 2.698458740408365879E-16, -1.110223024625156540E-16 ) ) ;
#17453=PLANE ( 'NONE',  #2884 ) ;
#17454=CARTESIAN_POINT ( 'NONE',  ( 138.6922820468854525, -1.999999999999979128, -32.39392330124607611 ) ) ;
#17455=LINE ( 'NONE', #14403, #10252 ) ;
#17456=DIRECTION ( 'NONE',  ( -0.9510565162951536422, 0.000000000000000000, -0.3090169943749472292 ) ) ;
#17459=DIRECTION ( 'NONE',  ( 0.9510565162951535312, 2.566386769018988816E-16, -0.3090169943749475623 ) ) ;
#17461=DIRECTION ( 'NONE',  ( 0.5877852522924731371, 0.000000000000000000, 0.8090169943749474513 ) ) ;
#17471=EDGE_LOOP ( 'NONE', ( #23740, #11127, #27670, #2487, #20789 ) ) ;
#17473=AXIS2_PLACEMENT_3D ( 'NONE', #19135, #9824, #12265 ) ;
#17474=VERTEX_POINT ( 'NONE', #571 ) ;
#17475=CARTESIAN_POINT ( 'NONE',  ( 157.2287565553229172, -10.00000000000000178, -3.509618943233403510 ) ) ;
#17476=VECTOR ( 'NONE', #18901, 1000.000000000000000 ) ;
#17477=ORIENTED_EDGE ( 'NONE', *, *, #16869, .T. ) ;
#17478=ORIENTED_EDGE ( 'NONE', *, *, #25396, .F. ) ;
#17479=LINE ( 'NONE', #710, #9735 ) ;
#17480=DIRECTION ( 'NONE',  ( -2.908569913943825554E-16, 1.000000000000000000, -6.826925868028084042E-18 ) ) ;
#17482=LINE ( 'NONE', #26832, #6075 ) ;
#17484=EDGE_CURVE ( 'NONE', #16280, #3964, #7877, .T. ) ;
#17486=CARTESIAN_POINT ( 'NONE',  ( 149.5152310637605808, -1.999999999999975353, -30.37205893520531319 ) ) ;
#17489=LINE ( 'NONE', #28684, #17101 ) ;
#17490=CARTESIAN_POINT ( 'NONE',  ( 131.1922820468854241, -1.999999999999982236, -30.91696583120935671 ) ) ;
#17494=CARTESIAN_POINT ( 'NONE',  ( 154.5152310637605240, -4.999999999999975131, -11.28819510263909542 ) ) ;
#17495=VERTEX_POINT ( 'NONE', #5443 ) ;
#17496=VECTOR ( 'NONE', #197, 1000.000000000000000 ) ;
#17497=CARTESIAN_POINT ( 'NONE',  ( 149.7287565553230309, -10.00000000000000178, -33.82050807568879947 ) ) ;
#17498=CARTESIAN_POINT ( 'NONE',  ( 163.6922820468853104, -9.999999999999998224, -6.413161187712876909 ) ) ;
#17500=ORIENTED_EDGE ( 'NONE', *, *, #28881, .T. ) ;
#17502=ORIENTED_EDGE ( 'NONE', *, *, #11041, .F. ) ;
#17506=CARTESIAN_POINT ( 'NONE',  ( 175.7287565553229456, -4.999999999999970690, -33.50000000000000000 ) ) ;
#17507=CARTESIAN_POINT ( 'NONE',  ( 157.0152310637605524, -9.999999999999998224, -34.70218595412750773 ) ) ;
#17509=ADVANCED_FACE ( 'NONE', ( #9857 ), #17186, .T. ) ;
#17510=ORIENTED_EDGE ( 'NONE', *, *, #23084, .T. ) ;
#17511=LINE ( 'NONE', #24549, #21100 ) ;
#17513=VECTOR ( 'NONE', #12341, 1000.000000000000000 ) ;
#17515=CARTESIAN_POINT ( 'NONE',  ( 153.6922820468853388, -4.999999999999976907, -17.92658477444275533 ) ) ;
#17516=CARTESIAN_POINT ( 'NONE',  ( 149.5152310637605524, -10.00000000000000178, -11.28819510263909542 ) ) ;
#17522=ORIENTED_EDGE ( 'NONE', *, *, #16517, .F. ) ;
#17526=FACE_BOUND ( 'NONE', #27940, .T. ) ;
#17527=ORIENTED_EDGE ( 'NONE', *, *, #7405, .F. ) ;
#17528=PLANE ( 'NONE',  #8553 ) ;
#17531=VERTEX_POINT ( 'NONE', #21309 ) ;
#17532=CARTESIAN_POINT ( 'NONE',  ( 133.6922820468854241, -10.00000000000000711, -9.266330736598357376 ) ) ;
#17533=ORIENTED_EDGE ( 'NONE', *, *, #20617, .F. ) ;
#17536=EDGE_LOOP ( 'NONE', ( #9492, #27914, #19618, #7115, #22777 ) ) ;
#17540=VECTOR ( 'NONE', #25408, 1000.000000000000000 ) ;
#17541=CARTESIAN_POINT ( 'NONE',  ( 156.1922820468854241, -4.999999999999975131, -28.06379628232387802 ) ) ;
#17542=ORIENTED_EDGE ( 'NONE', *, *, #3281, .F. ) ;
#17546=EDGE_CURVE ( 'NONE', #21674, #21255, #3019, .T. ) ;
#17547=ADVANCED_FACE ( 'NONE', ( #23764 ), #1027, .T. ) ;
#17549=CARTESIAN_POINT ( 'NONE',  ( 171.1922820468853388, -1.999999999999970024, -19.40354224447947828 ) ) ;
#17550=VECTOR ( 'NONE', #28359, 1000.000000000000000 ) ;
#17551=FACE_OUTER_BOUND ( 'NONE', #23559, .T. ) ;
#17552=AXIS2_PLACEMENT_3D ( 'NONE', #26339, #24050, #3149 ) ;
#17553=ORIENTED_EDGE ( 'NONE', *, *, #4868, .F. ) ;
#17554=EDGE_LOOP ( 'NONE', ( #26806, #22286, #6136, #24478 ) ) ;
#17555=DIRECTION ( 'NONE',  ( -2.698458740408365879E-16, 1.000000000000000000, 0.000000000000000000 ) ) ;
#17558=CARTESIAN_POINT ( 'NONE',  ( 166.1922820468853104, -1.999999999999972689, -4.936203717676158398 ) ) ;
#17559=LINE ( 'NONE', #27226, #12437 ) ;
#17563=FACE_OUTER_BOUND ( 'NONE', #17205, .T. ) ;
#17564=ORIENTED_EDGE ( 'NONE', *, *, #12252, .F. ) ;
#17566=CARTESIAN_POINT ( 'NONE',  ( 175.7287565553229456, -9.999999999999994671, -4.785595155761523500 ) ) ;
#17567=CARTESIAN_POINT ( 'NONE',  ( 146.1922820468854525, -1.999999999999977129, -22.25671179336496053 ) ) ;
#17568=ORIENTED_EDGE ( 'NONE', *, *, #3915, .T. ) ;
#17569=LINE ( 'NONE', #10707, #11998 ) ;
#17572=VECTOR ( 'NONE', #26533, 1000.000000000000000 ) ;
#17576=VERTEX_POINT ( 'NONE', #7723 ) ;
#17577=DIRECTION ( 'NONE',  ( 1.000000000000000000, 2.698458740408365879E-16, -1.110223024625156540E-16 ) ) ;
#17579=DIRECTION ( 'NONE',  ( -2.698458740408365879E-16, 1.000000000000000000, 0.000000000000000000 ) ) ;
#17582=EDGE_CURVE ( 'NONE', #12464, #19711, #25906, .T. ) ;
#17587=EDGE_CURVE ( 'NONE', #18177, #10339, #11355, .T. ) ;
#17588=ORIENTED_EDGE ( 'NONE', *, *, #12554, .T. ) ;
#17589=CARTESIAN_POINT ( 'NONE',  ( 133.6922820468854241, -1.999999999999980904, 2.247092850131519715 ) ) ;
#17590=DIRECTION ( 'NONE',  ( 0.3090169943749475623, 8.338696094058001131E-17, 0.9510565162951536422 ) ) ;
#17591=LINE ( 'NONE', #22487, #1166 ) ;
#17593=CARTESIAN_POINT ( 'NONE',  ( 152.2287565553230309, -10.00000000000000178, -29.49038105676660493 ) ) ;
#17594=CARTESIAN_POINT ( 'NONE',  ( 13.54327048257564314, -5.000000000000014211, 41.68190060373459005 ) ) ;
#17595=VECTOR ( 'NONE', #851, 999.9999999999998863 ) ;
#17596=PLANE ( 'NONE',  #8525 ) ;
#17600=VERTEX_POINT ( 'NONE', #19316 ) ;
#17602=CARTESIAN_POINT ( 'NONE',  ( 144.5152310637606092, -1.999999999999977129, -19.94844914048349693 ) ) ;
#17604=CARTESIAN_POINT ( 'NONE',  ( 131.1922820468854241, -10.00000000000000888, -13.59645775552055547 ) ) ;
#17605=DIRECTION ( 'NONE',  ( -0.5877852522924731371, 0.000000000000000000, 0.8090169943749474513 ) ) ;
#17608=ORIENTED_EDGE ( 'NONE', *, *, #24775, .F. ) ;
#17609=CARTESIAN_POINT ( 'NONE',  ( 163.6922820468853388, -4.999999999999973355, -15.07341522555727664 ) ) ;
#17612=PLANE ( 'NONE',  #29364 ) ;
#17614=DIRECTION ( 'NONE',  ( -0.5877852522924731371, -1.586114251531760728E-16, -0.8090169943749474513 ) ) ;
#17616=VERTEX_POINT ( 'NONE', #26365 ) ;
#17621=EDGE_CURVE ( 'NONE', #1987, #4875, #14725, .T. ) ;
#17622=EDGE_CURVE ( 'NONE', #7797, #25128, #12439, .T. ) ;
#17624=EDGE_CURVE ( 'NONE', #11448, #28119, #13050, .T. ) ;
#17625=ADVANCED_FACE ( 'NONE', ( #27295 ), #10765, .T. ) ;
#17626=LINE ( 'NONE', #2376, #16586 ) ;
#17627=VERTEX_POINT ( 'NONE', #24975 ) ;
#17628=FACE_OUTER_BOUND ( 'NONE', #10648, .T. ) ;
#17629=CARTESIAN_POINT ( 'NONE',  ( 175.7287565553229456, -4.999999999999970690, 3.500000000000003109 ) ) ;
#17630=DIRECTION ( 'NONE',  ( 0.5877852522924731371, 1.586114251531760728E-16, 0.8090169943749474513 ) ) ;
#17631=LINE ( 'NONE', #1324, #17260 ) ;
#17632=AXIS2_PLACEMENT_3D ( 'NONE', #3974, #9124, #1855 ) ;
#17637=CARTESIAN_POINT ( 'NONE',  ( 120.6264357055466689, -4.999999999999984901, -87.64023554178400843 ) ) ;
#17639=LINE ( 'NONE', #13218, #11255 ) ;
#17641=DIRECTION ( 'NONE',  ( -0.8090169943749474513, -2.183098979609982436E-16, 0.5877852522924731371 ) ) ;
#17644=ORIENTED_EDGE ( 'NONE', *, *, #612, .T. ) ;
#17646=CARTESIAN_POINT ( 'NONE',  ( 161.1922820468853672, -1.999999999999973133, -22.25671179336496053 ) ) ;
#17647=VECTOR ( 'NONE', #2535, 1000.000000000000000 ) ;
#17648=CARTESIAN_POINT ( 'NONE',  ( 174.7287565553229172, -1.999999999999968914, -25.16025403784440329 ) ) ;
#17649=ORIENTED_EDGE ( 'NONE', *, *, #11031, .T. ) ;
#17652=ORIENTED_EDGE ( 'NONE', *, *, #5676, .T. ) ;
#17654=EDGE_CURVE ( 'NONE', #26426, #2723, #17918, .T. ) ;
#17656=CARTESIAN_POINT ( 'NONE',  ( 172.7287565553229456, -3.999999999999989786, -41.50000000000000711 ) ) ;
#17657=PLANE ( 'NONE',  #24315 ) ;
#17659=ADVANCED_FACE ( 'NONE', ( #29284 ), #29755, .T. ) ;
#17660=CARTESIAN_POINT ( 'NONE',  ( 139.5152310637605808, -10.00000000000000533, -30.37205893520530964 ) ) ;
#17661=ADVANCED_FACE ( 'NONE', ( #17628 ), #15179, .T. ) ;
#17664=DIRECTION ( 'NONE',  ( 0.3090169943749475623, 8.338696094058001131E-17, 0.9510565162951536422 ) ) ;
#17665=VERTEX_POINT ( 'NONE', #19920 ) ;
#17666=VECTOR ( 'NONE', #27658, 1000.000000000000000 ) ;
#17667=APPLICATION_CONTEXT ( 'automotive_design' ) ;
#17668=CARTESIAN_POINT ( 'NONE',  ( 142.2287565553230309, -4.999999999999979572, -12.16987298107780013 ) ) ;
#17669=LINE ( 'NONE', #29643, #8468 ) ;
#17674=VERTEX_POINT ( 'NONE', #3906 ) ;
#17675=AXIS2_PLACEMENT_3D ( 'NONE', #10488, #12934, #6529 ) ;
#17678=FACE_BOUND ( 'NONE', #556, .T. ) ;
#17679=ADVANCED_FACE ( 'NONE', ( #24363 ), #29128, .T. ) ;
#17680=VERTEX_POINT ( 'NONE', #1777 ) ;
#17681=LINE ( 'NONE', #27037, #18316 ) ;
#17683=CARTESIAN_POINT ( 'NONE',  ( 13.38537325061315286, -5.000000000000014211, 41.19594289235809015 ) ) ;
#17684=VERTEX_POINT ( 'NONE', #29602 ) ;
#17685=DIRECTION ( 'NONE',  ( 0.9510565162951535312, 2.566386769018988816E-16, -0.3090169943749475623 ) ) ;
#17686=VERTEX_POINT ( 'NONE', #4055 ) ;
#17688=ORIENTED_EDGE ( 'NONE', *, *, #12414, .T. ) ;
#17692=DIRECTION ( 'NONE',  ( 1.000000000000000000, 2.698458740408365879E-16, -1.110223024625156540E-16 ) ) ;
#17694=VECTOR ( 'NONE', #28947, 1000.000000000000000 ) ;
#17696=PLANE ( 'NONE',  #8880 ) ;
#17697=ORIENTED_EDGE ( 'NONE', *, *, #8578, .F. ) ;
#17702=ORIENTED_EDGE ( 'NONE', *, *, #10827, .F. ) ;
#17703=DIRECTION ( 'NONE',  ( 0.9510565162951536422, 0.000000000000000000, -0.3090169943749475623 ) ) ;
#17709=CARTESIAN_POINT ( 'NONE',  ( 149.7287565553230309, -4.999999999999977796, -33.82050807568879947 ) ) ;
#17712=ADVANCED_FACE ( 'NONE', ( #29453 ), #22674, .T. ) ;
#17715=CARTESIAN_POINT ( 'NONE',  ( 172.2287565553229456, -1.999999999999969358, -29.49038105676660493 ) ) ;
#17716=CARTESIAN_POINT ( 'NONE',  ( 138.6922820468854525, -4.999999999999980460, -26.58683881228715506 ) ) ;
#17717=DIRECTION ( 'NONE',  ( -0.5877852522924731371, -1.586114251531760728E-16, -0.8090169943749474513 ) ) ;
#17724=DIRECTION ( 'NONE',  ( -0.5877852522924731371, -1.586114251531760728E-16, -0.8090169943749474513 ) ) ;
#17725=LINE ( 'NONE', #6144, #18445 ) ;
#17726=CARTESIAN_POINT ( 'NONE',  ( 139.7287565553230309, -1.999999999999978684, -33.82050807568879947 ) ) ;
#17729=ORIENTED_EDGE ( 'NONE', *, *, #12212, .F. ) ;
#17730=ORIENTED_EDGE ( 'NONE', *, *, #8325, .T. ) ;
#17731=CARTESIAN_POINT ( 'NONE',  ( 146.1922820468854241, -4.999999999999978684, -13.59645775552055902 ) ) ;
#17732=LINE ( 'NONE', #1588, #15542 ) ;
#17734=LINE ( 'NONE', #17877, #23091 ) ;
#17735=LINE ( 'NONE', #8878, #14464 ) ;
#17736=LINE ( 'NONE', #29414, #20887 ) ;
#17737=LINE ( 'NONE', #13316, #4635 ) ;
#17740=EDGE_LOOP ( 'NONE', ( #25024, #701, #20597, #25392 ) ) ;
#17742=CARTESIAN_POINT ( 'NONE',  ( 144.5152310637605808, -1.999999999999977129, -30.37205893520530964 ) ) ;
#17743=EDGE_CURVE ( 'NONE', #30193, #3398, #15029, .T. ) ;
#17744=EDGE_CURVE ( 'NONE', #11783, #19520, #8471, .T. ) ;
#17745=ORIENTED_EDGE ( 'NONE', *, *, #7202, .F. ) ;
#17746=CARTESIAN_POINT ( 'NONE',  ( 152.0152310637605524, -1.999999999999974909, -26.04193191628311155 ) ) ;
#17747=CARTESIAN_POINT ( 'NONE',  ( 134.5152310637605524, -1.999999999999980460, -4.391296821672111328 ) ) ;
#17748=VERTEX_POINT ( 'NONE', #5745 ) ;
#17749=CARTESIAN_POINT ( 'NONE',  ( 146.1922820468854241, -1.999999999999977573, -10.74328820663507678 ) ) ;
#17751=CARTESIAN_POINT ( 'NONE',  ( 134.7287565553230024, -4.999999999999982236, -33.82050807568879947 ) ) ;
#17752=LINE ( 'NONE', #27110, #13227 ) ;
#17753=EDGE_CURVE ( 'NONE', #11968, #1963, #15326, .T. ) ;
#17756=ORIENTED_EDGE ( 'NONE', *, *, #1039, .T. ) ;
#17757=CARTESIAN_POINT ( 'NONE',  ( 144.5152310637605808, -1.999999999999977573, -11.28819510263909542 ) ) ;
#17759=CARTESIAN_POINT ( 'NONE',  ( 146.1922820468854241, -1.999999999999977129, -10.74328820663507678 ) ) ;
#17760=DIRECTION ( 'NONE',  ( 0.5877852522924731371, 0.000000000000000000, 0.8090169943749474513 ) ) ;
#17762=VECTOR ( 'NONE', #15492, 1000.000000000000000 ) ;
#17763=LINE ( 'NONE', #1463, #13511 ) ;
#17765=EDGE_LOOP ( 'NONE', ( #2326, #1319, #16086, #13028 ) ) ;
#17766=DIRECTION ( 'NONE',  ( -2.698458740408365879E-16, 1.000000000000000000, 0.000000000000000000 ) ) ;
#17770=ORIENTED_EDGE ( 'NONE', *, *, #4777, .T. ) ;
#17771=CARTESIAN_POINT ( 'NONE',  ( 157.0152310637604955, -4.999999999999975131, -1.743219247438260128E-14 ) ) ;
#17772=DIRECTION ( 'NONE',  ( 1.000000000000000000, 2.698458740408365879E-16, -1.110223024625156540E-16 ) ) ;
#17773=LINE ( 'NONE', #17629, #13645 ) ;
#17774=DIRECTION ( 'NONE',  ( -0.5877852522924731371, -1.586114251531760235E-16, 0.8090169943749474513 ) ) ;
#17775=CARTESIAN_POINT ( 'NONE',  ( 9.885273420212257633, -5.000000000000015099, 30.42374326586335798 ) ) ;
#17776=VECTOR ( 'NONE', #2347, 1000.000000000000000 ) ;
#17777=DIRECTION ( 'NONE',  ( -2.698458740408365879E-16, 1.000000000000000000, 0.000000000000000000 ) ) ;
#17779=DIRECTION ( 'NONE',  ( 0.5877852522924731371, 1.586114251531760728E-16, -0.8090169943749474513 ) ) ;
#17783=EDGE_CURVE ( 'NONE', #7245, #3516, #13207, .T. ) ;
#17784=PLANE ( 'NONE',  #19535 ) ;
#17785=CARTESIAN_POINT ( 'NONE',  ( 23.24172714540143048, -5.000000000000011546, -71.53068101092122788 ) ) ;
#17786=EDGE_CURVE ( 'NONE', #4321, #9967, #3602, .T. ) ;
#17787=EDGE_CURVE ( 'NONE', #1554, #26475, #8324, .T. ) ;
#17789=CARTESIAN_POINT ( 'NONE',  ( 146.1922820468854525, -10.00000000000000178, -30.91696583120935671 ) ) ;
#17790=DIRECTION ( 'NONE',  ( -1.110223024625156540E-16, 0.000000000000000000, -1.000000000000000000 ) ) ;
#17792=ORIENTED_EDGE ( 'NONE', *, *, #19476, .F. ) ;
#17793=CARTESIAN_POINT ( 'NONE',  ( 137.0152310637605524, -1.999999999999980016, -0.06116980274991495881 ) ) ;
#17794=CARTESIAN_POINT ( 'NONE',  ( 172.0152310637604103, -1.999999999999970468, -8.721423840594312082 ) ) ;
#17796=VERTEX_POINT ( 'NONE', #6946 ) ;
#17801=DIRECTION ( 'NONE',  ( -0.9510565162951536422, -2.566386769018988816E-16, -0.3090169943749472292 ) ) ;
#17802=FACE_OUTER_BOUND ( 'NONE', #28146, .T. ) ;
#17803=CIRCLE ( 'NONE', #10484, 3.000000000000002665 ) ;
#17804=CARTESIAN_POINT ( 'NONE',  ( 132.2287565553230309, -4.999999999999981348, -29.49038105676660848 ) ) ;
#17806=ORIENTED_EDGE ( 'NONE', *, *, #18448, .T. ) ;
#17807=CARTESIAN_POINT ( 'NONE',  ( 163.6922820468853672, -1.999999999999972244, -26.58683881228715862 ) ) ;
#17808=CARTESIAN_POINT ( 'NONE',  ( 149.5152310637604955, -4.999999999999976907, -1.659952520591373388E-14 ) ) ;
#17809=DIRECTION ( 'NONE',  ( -0.9510565162951536422, -2.566386769018988323E-16, 0.3090169943749475623 ) ) ;
#17810=CARTESIAN_POINT ( 'NONE',  ( 130.7287565553229172, -10.00000000000000888, -22.10610323145025902 ) ) ;
#17811=VECTOR ( 'NONE', #20867, 1000.000000000000000 ) ;
#17814=ORIENTED_EDGE ( 'NONE', *, *, #29403, .F. ) ;
#17817=EDGE_CURVE ( 'NONE', #16514, #21374, #79, .T. ) ;
#17823=DIRECTION ( 'NONE',  ( -2.698458740408365879E-16, 1.000000000000000000, 0.000000000000000000 ) ) ;
#17824=ADVANCED_FACE ( 'NONE', ( #6494 ), #16392, .T. ) ;
#17825=ORIENTED_EDGE ( 'NONE', *, *, #22532, .F. ) ;
#17826=PLANE ( 'NONE',  #2249 ) ;
#17829=CARTESIAN_POINT ( 'NONE',  ( 144.7287565553229740, -1.999999999999978018, 0.8205080756887930260 ) ) ;
#17830=CARTESIAN_POINT ( 'NONE',  ( 162.0152310637605524, -9.999999999999998224, -32.93883019725009120 ) ) ;
#17831=ORIENTED_EDGE ( 'NONE', *, *, #13208, .F. ) ;
#17837=DIRECTION ( 'NONE',  ( -0.5877852522924731371, -1.586114251531760235E-16, 0.8090169943749474513 ) ) ;
#17841=CARTESIAN_POINT ( 'NONE',  ( 142.0152310637605524, -1.999999999999978462, -8.721423840594312082 ) ) ;
#17842=VERTEX_POINT ( 'NONE', #8763 ) ;
#17843=VERTEX_POINT ( 'NONE', #23118 ) ;
#17844=DIRECTION ( 'NONE',  ( 0.9510565162951536422, 0.000000000000000000, -0.3090169943749475623 ) ) ;
#17846=CARTESIAN_POINT ( 'NONE',  ( 16.40801556695141628, -5.000000000000013323, 50.49867938812164425 ) ) ;
#17847=VERTEX_POINT ( 'NONE', #15784 ) ;
#17849=VECTOR ( 'NONE', #9500, 1000.000000000000000 ) ;
#17850=EDGE_CURVE ( 'NONE', #4159, #6652, #22826, .T. ) ;
#17854=ORIENTED_EDGE ( 'NONE', *, *, #10161, .T. ) ;
#17855=AXIS2_PLACEMENT_3D ( 'NONE', #5496, #14782, #19669 ) ;
#17860=DIRECTION ( 'NONE',  ( -2.698458740408365879E-16, 1.000000000000000000, 0.000000000000000000 ) ) ;
#17861=VERTEX_POINT ( 'NONE', #20517 ) ;
#17865=VERTEX_POINT ( 'NONE', #4796 ) ;
#17866=CARTESIAN_POINT ( 'NONE',  ( 131.1922820468854241, -1.999999999999982236, -4.936203717676158398 ) ) ;
#17868=DIRECTION ( 'NONE',  ( -0.8090169943749474513, -2.183098979609982436E-16, -0.5877852522924731371 ) ) ;
#17871=VECTOR ( 'NONE', #14814, 1000.000000000000000 ) ;
#17872=ORIENTED_EDGE ( 'NONE', *, *, #29751, .F. ) ;
#17873=EDGE_CURVE ( 'NONE', #4960, #1409, #27736, .T. ) ;
#17875=VECTOR ( 'NONE', #28479, 1000.000000000000000 ) ;
#17876=CARTESIAN_POINT ( 'NONE',  ( 168.6922820468853956, -9.999999999999996447, -32.39392330124607611 ) ) ;
#17877=CARTESIAN_POINT ( 'NONE',  ( 138.6922820468854525, -10.00000000000000533, -6.413161187712876909 ) ) ;
#17878=CARTESIAN_POINT ( 'NONE',  ( 172.0152310637604955, -9.999999999999994671, -34.70218595412750773 ) ) ;
#17880=DIRECTION ( 'NONE',  ( -0.9510565162951536422, -2.566386769018988323E-16, 0.3090169943749475623 ) ) ;
#17885=EDGE_LOOP ( 'NONE', ( #16755, #27388, #15538, #8812 ) ) ;
#17888=ORIENTED_EDGE ( 'NONE', *, *, #1892, .T. ) ;
#17890=VECTOR ( 'NONE', #14330, 1000.000000000000000 ) ;
#17891=LINE ( 'NONE', #16479, #413 ) ;
#17892=CARTESIAN_POINT ( 'NONE',  ( 143.6922820468853956, -10.00000000000000533, 2.247092850131519715 ) ) ;
#17893=DIRECTION ( 'NONE',  ( 1.000000000000000000, 2.698458740408365879E-16, -1.110223024625156540E-16 ) ) ;
#17895=ORIENTED_EDGE ( 'NONE', *, *, #10343, .T. ) ;
#17896=EDGE_LOOP ( 'NONE', ( #6701, #22213, #27423, #1993 ) ) ;
#17897=DIRECTION ( 'NONE',  ( -0.9510565162951536422, -2.566386769018988323E-16, 0.3090169943749475623 ) ) ;
#17899=VECTOR ( 'NONE', #20917, 1000.000000000000000 ) ;
#17900=CARTESIAN_POINT ( 'NONE',  ( 180.7287565553229456, -3.999999999999989786, 0.5000000000000029976 ) ) ;
#17902=ORIENTED_EDGE ( 'NONE', *, *, #24531, .T. ) ;
#17906=ORIENTED_EDGE ( 'NONE', *, *, #23807, .T. ) ;
#17907=DIRECTION ( 'NONE',  ( -2.698458740408365879E-16, 1.000000000000000000, 0.000000000000000000 ) ) ;
#17908=EDGE_LOOP ( 'NONE', ( #24162, #1264, #6510, #24053 ) ) ;
#17911=VERTEX_POINT ( 'NONE', #23420 ) ;
#17912=ORIENTED_EDGE ( 'NONE', *, *, #29655, .T. ) ;
#17913=EDGE_CURVE ( 'NONE', #6453, #5386, #2537, .T. ) ;
#17916=EDGE_CURVE ( 'NONE', #18174, #2968, #27890, .T. ) ;
#17918=LINE ( 'NONE', #22212, #16239 ) ;
#17919=VERTEX_POINT ( 'NONE', #16085 ) ;
#17920=DIRECTION ( 'NONE',  ( 0.3090169943749472292, 8.338696094057992503E-17, -0.9510565162951536422 ) ) ;
#17921=AXIS2_PLACEMENT_3D ( 'NONE', #20763, #20469, #11010 ) ;
#17922=LINE ( 'NONE', #27298, #25263 ) ;
#17923=DIRECTION ( 'NONE',  ( -0.5877852522924731371, -1.586114251531760728E-16, -0.8090169943749474513 ) ) ;
#17929=VECTOR ( 'NONE', #28762, 1000.000000000000000 ) ;
#17932=FACE_OUTER_BOUND ( 'NONE', #10960, .T. ) ;
#17935=PLANE ( 'NONE',  #5373 ) ;
#17936=ORIENTED_EDGE ( 'NONE', *, *, #18210, .F. ) ;
#17939=ORIENTED_EDGE ( 'NONE', *, *, #15965, .T. ) ;
#17940=DIRECTION ( 'NONE',  ( 0.5877852522924731371, 1.586114251531760728E-16, 0.8090169943749474513 ) ) ;
#17941=LINE ( 'NONE', #27316, #20042 ) ;
#17942=AXIS2_PLACEMENT_3D ( 'NONE', #3811, #4110, #24570 ) ;
#17943=DIRECTION ( 'NONE',  ( -2.698458740408365879E-16, 1.000000000000000000, 0.000000000000000000 ) ) ;
#17947=VECTOR ( 'NONE', #15055, 1000.000000000000000 ) ;
#17951=AXIS2_PLACEMENT_3D ( 'NONE', #1660, #8503, #22245 ) ;
#17952=DIRECTION ( 'NONE',  ( 0.5877852522924731371, 0.000000000000000000, 0.8090169943749474513 ) ) ;
#17954=ADVANCED_FACE ( 'NONE', ( #25552 ), #4646, .T. ) ;
#17955=VECTOR ( 'NONE', #27963, 999.9999999999998863 ) ;
#17956=ADVANCED_FACE ( 'NONE', ( #8912 ), #25111, .T. ) ;
#17957=ADVANCED_FACE ( 'NONE', ( #18228 ), #13792, .T. ) ;
#17958=VERTEX_POINT ( 'NONE', #15937 ) ;
#17960=CARTESIAN_POINT ( 'NONE',  ( 158.6922820468853388, -1.999999999999974021, -6.413161187712876909 ) ) ;
#17962=ORIENTED_EDGE ( 'NONE', *, *, #30234, .T. ) ;
#17965=PLANE ( 'NONE',  #20935 ) ;
#17968=AXIS2_PLACEMENT_3D ( 'NONE', #1659, #10937, #22404 ) ;
#17969=ORIENTED_EDGE ( 'NONE', *, *, #17005, .F. ) ;
#17971=EDGE_LOOP ( 'NONE', ( #21513, #21388, #20686, #16336 ) ) ;
#17973=DIRECTION ( 'NONE',  ( -1.110223024625156540E-16, 0.000000000000000000, -1.000000000000000000 ) ) ;
#17975=CARTESIAN_POINT ( 'NONE',  ( 130.7287565553229456, -10.00000000000000888, -13.44584919360586284 ) ) ;
#17976=VECTOR ( 'NONE', #6079, 1000.000000000000000 ) ;
#17978=LINE ( 'NONE', #15077, #7584 ) ;
#17980=DIRECTION ( 'NONE',  ( -0.9510565162951536422, -2.566386769018988323E-16, 0.3090169943749475623 ) ) ;
#17981=ORIENTED_EDGE ( 'NONE', *, *, #4600, .T. ) ;
#17983=ORIENTED_EDGE ( 'NONE', *, *, #20922, .T. ) ;
#17985=VERTEX_POINT ( 'NONE', #30046 ) ;
#17988=VECTOR ( 'NONE', #30177, 1000.000000000000000 ) ;
#17990=ORIENTED_EDGE ( 'NONE', *, *, #23562, .T. ) ;
#17991=PLANE ( 'NONE',  #15214 ) ;
#17992=VECTOR ( 'NONE', #5215, 1000.000000000000000 ) ;
#17995=ADVANCED_FACE ( 'NONE', ( #5100 ), #17149, .T. ) ;
#17996=EDGE_CURVE ( 'NONE', #23960, #1065, #28638, .T. ) ;
#17997=ORIENTED_EDGE ( 'NONE', *, *, #10522, .T. ) ;
#17998=VECTOR ( 'NONE', #15677, 1000.000000000000000 ) ;
#17999=FACE_OUTER_BOUND ( 'NONE', #4270, .T. ) ;
#18002=ORIENTED_EDGE ( 'NONE', *, *, #14652, .T. ) ;
#18003=VERTEX_POINT ( 'NONE', #10119 ) ;
#18004=CARTESIAN_POINT ( 'NONE',  ( 130.7287565553229456, -4.999999999999983125, 3.500000000000003109 ) ) ;
#18006=FACE_OUTER_BOUND ( 'NONE', #20174, .T. ) ;
#18007=EDGE_LOOP ( 'NONE', ( #22554, #1423, #8307, #23403 ) ) ;
#18008=ORIENTED_EDGE ( 'NONE', *, *, #27650, .F. ) ;
#18009=CARTESIAN_POINT ( 'NONE',  ( 141.1922820468854525, -1.999999999999978684, -30.91696583120935671 ) ) ;
#18015=ORIENTED_EDGE ( 'NONE', *, *, #11656, .T. ) ;
#18016=FACE_OUTER_BOUND ( 'NONE', #6943, .T. ) ;
#18017=VECTOR ( 'NONE', #9177, 1000.000000000000000 ) ;
#18021=VECTOR ( 'NONE', #19690, 1000.000000000000000 ) ;
#18022=ORIENTED_EDGE ( 'NONE', *, *, #11318, .T. ) ;
#18024=CARTESIAN_POINT ( 'NONE',  ( 107.4261961205572931, -4.999999999999988454, -78.04970010342938735 ) ) ;
#18025=ORIENTED_EDGE ( 'NONE', *, *, #27450, .F. ) ;
#18029=ORIENTED_EDGE ( 'NONE', *, *, #20441, .T. ) ;
#18030=CARTESIAN_POINT ( 'NONE',  ( 159.5152310637605240, -9.999999999999998224, -19.94844914048349693 ) ) ;
#18033=VECTOR ( 'NONE', #14813, 1000.000000000000000 ) ;
#18035=EDGE_CURVE ( 'NONE', #17865, #18212, #16997, .T. ) ;
#18036=EDGE_CURVE ( 'NONE', #7426, #2040, #9508, .T. ) ;
#18037=VERTEX_POINT ( 'NONE', #12406 ) ;
#18038=CARTESIAN_POINT ( 'NONE',  ( 157.2287565553229740, -10.00000000000000000, -20.83012701892220520 ) ) ;
#18039=VECTOR ( 'NONE', #7819, 1000.000000000000000 ) ;
#18040=CARTESIAN_POINT ( 'NONE',  ( 152.0152310637605808, -1.999999999999974909, -24.27857615940569502 ) ) ;
#18041=DIRECTION ( 'NONE',  ( 0.5877852522924731371, 1.586114251531760728E-16, 0.8090169943749474513 ) ) ;
#18042=CARTESIAN_POINT ( 'NONE',  ( 141.1922820468854525, -1.999999999999978684, -10.74328820663507678 ) ) ;
#18043=UNCERTAINTY_MEASURE_WITH_UNIT (LENGTH_MEASURE( 1.000000000000000082E-05 ), #29441, 'distance_accuracy_value', 'NONE');
#18046=LINE ( 'NONE', #17742, #16012 ) ;
#18048=VECTOR ( 'NONE', #12875, 1000.000000000000000 ) ;
#18051=EDGE_LOOP ( 'NONE', ( #4563, #4671, #16719, #15070, #26620 ) ) ;
#18052=VECTOR ( 'NONE', #20096, 1000.000000000000000 ) ;
#18054=DIRECTION ( 'NONE',  ( 0.9510565162951536422, 2.566386769018988816E-16, 0.3090169943749472292 ) ) ;
#18057=CARTESIAN_POINT ( 'NONE',  ( 168.6922820468852819, -4.999999999999971578, -0.6060766987539614181 ) ) ;
#18059=ORIENTED_EDGE ( 'NONE', *, *, #21683, .T. ) ;
#18061=CARTESIAN_POINT ( 'NONE',  ( 130.7287565553229456, -9.999999999999982236, 3.500000000000003109 ) ) ;
#18063=EDGE_CURVE ( 'NONE', #11008, #23288, #9966, .T. ) ;
#18064=VECTOR ( 'NONE', #5173, 1000.000000000000000 ) ;
#18068=LINE ( 'NONE', #6333, #28185 ) ;
#18070=ORIENTED_EDGE ( 'NONE', *, *, #6862, .T. ) ;
#18071=CARTESIAN_POINT ( 'NONE',  ( 139.5152310637606092, -10.00000000000000533, -28.60870317832789311 ) ) ;
#18072=SURFACE_STYLE_FILL_AREA ( #18222 ) ;
#18075=EDGE_CURVE ( 'NONE', #12812, #26944, #26478, .T. ) ;
#18076=VERTEX_POINT ( 'NONE', #4951 ) ;
#18077=VECTOR ( 'NONE', #22841, 1000.000000000000000 ) ;
#18078=PLANE ( 'NONE',  #2952 ) ;
#18079=CONICAL_SURFACE ( 'NONE', #21987, 5.999999999999970690, 0.7853981633974530530 ) ;
#18080=CARTESIAN_POINT ( 'NONE',  ( 147.0152310637606092, -10.00000000000000178, -32.93883019725009120 ) ) ;
#18082=FACE_OUTER_BOUND ( 'NONE', #8394, .T. ) ;
#18083=DIRECTION ( 'NONE',  ( -1.110223024625156540E-16, 0.000000000000000000, -1.000000000000000000 ) ) ;
#18084=LINE ( 'NONE', #10770, #18727 ) ;
#18092=CARTESIAN_POINT ( 'NONE',  ( 174.5152310637604103, -9.999999999999994671, -2.627941064794695691 ) ) ;
#18095=ORIENTED_EDGE ( 'NONE', *, *, #22760, .F. ) ;
#18097=AXIS2_PLACEMENT_3D ( 'NONE', #19150, #16859, #26803 ) ;
#18099=EDGE_CURVE ( 'NONE', #20136, #16501, #19133, .T. ) ;
#18100=VERTEX_POINT ( 'NONE', #7402 ) ;
#18101=LINE ( 'NONE', #2400, #27143 ) ;
#18102=DIRECTION ( 'NONE',  ( -2.698458740408365879E-16, 1.000000000000000000, 0.000000000000000000 ) ) ;
#18103=ADVANCED_FACE ( 'NONE', ( #5251 ), #5559, .T. ) ;
#18104=DIRECTION ( 'NONE',  ( 0.5877852522924731371, 0.000000000000000000, 0.8090169943749474513 ) ) ;
#18105=VERTEX_POINT ( 'NONE', #229 ) ;
#18110=PLANE ( 'NONE',  #26960 ) ;
#18113=LINE ( 'NONE', #22713, #6008 ) ;
#18114=DIRECTION ( 'NONE',  ( -0.9510565162951536422, -2.566386769018988816E-16, -0.3090169943749472292 ) ) ;
#18117=CARTESIAN_POINT ( 'NONE',  ( 173.6922820468852535, -9.999999999999996447, -0.6060766987539614181 ) ) ;
#18118=DIRECTION ( 'NONE',  ( -0.9510565162951536422, 0.000000000000000000, -0.3090169943749472292 ) ) ;
#18120=ORIENTED_EDGE ( 'NONE', *, *, #439, .T. ) ;
#18123=VERTEX_POINT ( 'NONE', #18832 ) ;
#18127=FACE_OUTER_BOUND ( 'NONE', #11152, .T. ) ;
#18128=ORIENTED_EDGE ( 'NONE', *, *, #14907, .T. ) ;
#18129=ORIENTED_EDGE ( 'NONE', *, *, #22074, .T. ) ;
#18130=ADVANCED_FACE ( 'NONE', ( #11948 ), #12262, .T. ) ;
#18131=VERTEX_POINT ( 'NONE', #16703 ) ;
#18132=LINE ( 'NONE', #6548, #24656 ) ;
#18135=VECTOR ( 'NONE', #25780, 1000.000000000000000 ) ;
#18136=PLANE ( 'NONE',  #5258 ) ;
#18137=ORIENTED_EDGE ( 'NONE', *, *, #8149, .F. ) ;
#18138=EDGE_CURVE ( 'NONE', #4340, #27514, #2669, .T. ) ;
#18139=ORIENTED_EDGE ( 'NONE', *, *, #11070, .T. ) ;
#18140=DIRECTION ( 'NONE',  ( 0.9510565162951536422, 0.000000000000000000, -0.3090169943749475623 ) ) ;
#18141=EDGE_LOOP ( 'NONE', ( #16325, #18639, #12582, #2181 ) ) ;
#18145=VERTEX_POINT ( 'NONE', #381 ) ;
#18148=LINE ( 'NONE', #22898, #11316 ) ;
#18150=VECTOR ( 'NONE', #4277, 1000.000000000000000 ) ;
#18151=VERTEX_POINT ( 'NONE', #23728 ) ;
#18153=CARTESIAN_POINT ( 'NONE',  ( 147.2287565553230309, -10.00000000000000178, -20.83012701892220520 ) ) ;
#18154=VECTOR ( 'NONE', #10338, 1000.000000000000000 ) ;
#18156=EDGE_CURVE ( 'NONE', #16318, #1647, #26025, .T. ) ;
#18157=LINE ( 'NONE', #25190, #9229 ) ;
#18159=DIRECTION ( 'NONE',  ( -0.9510565162951536422, 0.000000000000000000, -0.3090169943749472292 ) ) ;
#18160=ORIENTED_EDGE ( 'NONE', *, *, #5897, .F. ) ;
#18161=ORIENTED_EDGE ( 'NONE', *, *, #6372, .F. ) ;
#18162=LINE ( 'NONE', #11432, #5133 ) ;
#18167=DIRECTION ( 'NONE',  ( -0.9510565162951536422, 0.000000000000000000, -0.3090169943749472292 ) ) ;
#18168=EDGE_CURVE ( 'NONE', #4109, #28929, #21429, .T. ) ;
#18170=LINE ( 'NONE', #2324, #29836 ) ;
#18172=EDGE_CURVE ( 'NONE', #19263, #17861, #21874, .T. ) ;
#18173=EDGE_CURVE ( 'NONE', #5025, #5499, #10869, .T. ) ;
#18174=VERTEX_POINT ( 'NONE', #15452 ) ;
#18175=CARTESIAN_POINT ( 'NONE',  ( 156.1922820468854241, -1.999999999999973577, -28.06379628232387802 ) ) ;
#18176=EDGE_CURVE ( 'NONE', #17207, #29150, #17591, .T. ) ;
#18177=VERTEX_POINT ( 'NONE', #24326 ) ;
#18181=DIRECTION ( 'NONE',  ( 2.908569913943825554E-16, -1.000000000000000000, 0.000000000000000000 ) ) ;
#18182=ORIENTED_EDGE ( 'NONE', *, *, #9838, .T. ) ;
#18183=VECTOR ( 'NONE', #9999, 1000.000000000000000 ) ;
#18184=CARTESIAN_POINT ( 'NONE',  ( 141.1922820468854525, -10.00000000000000533, -19.40354224447947473 ) ) ;
#18188=ORIENTED_EDGE ( 'NONE', *, *, #1806, .F. ) ;
#18190=LINE ( 'NONE', #6755, #3037 ) ;
#18191=LINE ( 'NONE', #15292, #27187 ) ;
#18192=DIRECTION ( 'NONE',  ( -0.5877852522924731371, -1.586114251531760235E-16, 0.8090169943749474513 ) ) ;
#18194=VECTOR ( 'NONE', #29559, 1000.000000000000000 ) ;
#18197=ORIENTED_EDGE ( 'NONE', *, *, #21558, .F. ) ;
#18199=ORIENTED_EDGE ( 'NONE', *, *, #19437, .F. ) ;
#18201=EDGE_CURVE ( 'NONE', #27047, #18859, #17437, .T. ) ;
#18203=PLANE ( 'NONE',  #11216 ) ;
#18204=DIRECTION ( 'NONE',  ( -0.9510565162951536422, 0.000000000000000000, -0.3090169943749472292 ) ) ;
#18205=EDGE_CURVE ( 'NONE', #16252, #20351, #1591, .T. ) ;
#18208=ORIENTED_EDGE ( 'NONE', *, *, #25485, .T. ) ;
#18209=DIRECTION ( 'NONE',  ( -2.698458740408365879E-16, 1.000000000000000000, 0.000000000000000000 ) ) ;
#18210=EDGE_CURVE ( 'NONE', #9707, #22500, #22030, .T. ) ;
#18212=VERTEX_POINT ( 'NONE', #22175 ) ;
#18214=CARTESIAN_POINT ( 'NONE',  ( 162.2287565553229172, -4.999999999999973355, -20.83012701892220164 ) ) ;
#18215=ORIENTED_EDGE ( 'NONE', *, *, #22873, .T. ) ;
#18217=LINE ( 'NONE', #9043, #27699 ) ;
#18221=VERTEX_POINT ( 'NONE', #1284 ) ;
#18222=FILL_AREA_STYLE ('',( #29896 ) ) ;
#18227=CYLINDRICAL_SURFACE ( 'NONE', #3445, 8.000000000000007105 ) ;
#18228=FACE_OUTER_BOUND ( 'NONE', #19670, .T. ) ;
#18229=DIRECTION ( 'NONE',  ( 0.9510565162951536422, 0.000000000000000000, -0.3090169943749475623 ) ) ;
#18231=CARTESIAN_POINT ( 'NONE',  ( 161.1922820468853104, -1.999999999999974021, -4.936203717676158398 ) ) ;
#18232=DIRECTION ( 'NONE',  ( 0.3090169943749475623, 8.338696094058001131E-17, 0.9510565162951536422 ) ) ;
#18238=AXIS2_PLACEMENT_3D ( 'NONE', #14877, #28680, #5596 ) ;
#18239=DIRECTION ( 'NONE',  ( -0.5877852522924731371, -1.586114251531760235E-16, 0.8090169943749474513 ) ) ;
#18240=DIRECTION ( 'NONE',  ( 0.9510565162951535312, 2.566386769018988816E-16, -0.3090169943749475623 ) ) ;
#18242=ADVANCED_FACE ( 'NONE', ( #24933 ), #6307, .T. ) ;
#18243=DIRECTION ( 'NONE',  ( 0.9510565162951536422, 0.000000000000000000, -0.3090169943749475623 ) ) ;
#18244=ORIENTED_EDGE ( 'NONE', *, *, #28694, .T. ) ;
#18245=DIRECTION ( 'NONE',  ( 0.3090169943749475623, 8.338696094058001131E-17, 0.9510565162951536422 ) ) ;
#18246=EDGE_CURVE ( 'NONE', #3020, #25860, #24780, .T. ) ;
#18248=ORIENTED_EDGE ( 'NONE', *, *, #26932, .T. ) ;
#18249=CARTESIAN_POINT ( 'NONE',  ( 144.5152310637605524, -1.999999999999977573, -13.05155085951651195 ) ) ;
#18252=CARTESIAN_POINT ( 'NONE',  ( 161.1922820468853956, -9.999999999999998224, -28.06379628232387802 ) ) ;
#18253=ORIENTED_EDGE ( 'NONE', *, *, #4401, .T. ) ;
#18258=DIRECTION ( 'NONE',  ( 0.5877852522924731371, 1.586114251531760728E-16, 0.8090169943749474513 ) ) ;
#18260=AXIS2_PLACEMENT_3D ( 'NONE', #4166, #2046, #16050 ) ;
#18261=EDGE_LOOP ( 'NONE', ( #10044, #1300, #26964, #26575 ) ) ;
#18264=EDGE_CURVE ( 'NONE', #19635, #18890, #17734, .T. ) ;
#18265=EDGE_CURVE ( 'NONE', #10473, #22161, #15290, .T. ) ;
#18266=CARTESIAN_POINT ( 'NONE',  ( 149.5152310637605524, -4.999999999999976907, -21.71180489736091346 ) ) ;
#18268=CARTESIAN_POINT ( 'NONE',  ( 129.5152310637605808, -10.00000000000000888, -2.627941064794695691 ) ) ;
#18272=ORIENTED_EDGE ( 'NONE', *, *, #12891, .T. ) ;
#18274=DIRECTION ( 'NONE',  ( -2.698458740408365879E-16, 1.000000000000000000, 0.000000000000000000 ) ) ;
#18276=DIRECTION ( 'NONE',  ( 0.3090169943749475623, 8.338696094058001131E-17, 0.9510565162951536422 ) ) ;
#18277=PLANE ( 'NONE',  #5708 ) ;
#18278=ORIENTED_EDGE ( 'NONE', *, *, #7871, .T. ) ;
#18279=DIRECTION ( 'NONE',  ( -2.698458740408365879E-16, 1.000000000000000000, 0.000000000000000000 ) ) ;
#18280=VECTOR ( 'NONE', #2464, 1000.000000000000000 ) ;
#18281=CARTESIAN_POINT ( 'NONE',  ( 154.5152310637605240, -1.999999999999974909, -11.28819510263909542 ) ) ;
#18283=ORIENTED_EDGE ( 'NONE', *, *, #17440, .T. ) ;
#18284=PLANE ( 'NONE',  #11056 ) ;
#18285=VERTEX_POINT ( 'NONE', #10575 ) ;
#18291=ORIENTED_EDGE ( 'NONE', *, *, #26932, .F. ) ;
#18293=VECTOR ( 'NONE', #29916, 1000.000000000000000 ) ;
#18295=AXIS2_PLACEMENT_3D ( 'NONE', #7892, #21481, #28397 ) ;
#18296=DIRECTION ( 'NONE',  ( -6.938893903907227392E-16, 0.000000000000000000, -1.000000000000000000 ) ) ;
#18297=ADVANCED_FACE ( 'NONE', ( #22332 ), #3870, .T. ) ;
#18298=LINE ( 'NONE', #29974, #26979 ) ;
#18299=EDGE_CURVE ( 'NONE', #19125, #18552, #19879, .T. ) ;
#18300=VECTOR ( 'NONE', #26757, 999.9999999999998863 ) ;
#18301=ADVANCED_FACE ( 'NONE', ( #15142 ), #24623, .T. ) ;
#18302=VECTOR ( 'NONE', #24676, 1000.000000000000000 ) ;
#18303=EDGE_CURVE ( 'NONE', #3213, #5949, #5709, .T. ) ;
#18306=CYLINDRICAL_SURFACE ( 'NONE', #4860, 3.000000000000002665 ) ;
#18308=VERTEX_POINT ( 'NONE', #12709 ) ;
#18309=DIRECTION ( 'NONE',  ( 0.3090169943749472292, 8.338696094057992503E-17, -0.9510565162951536422 ) ) ;
#18312=CARTESIAN_POINT ( 'NONE',  ( 163.6922820468853956, -9.999999999999998224, -35.24709285013155835 ) ) ;
#18313=ORIENTED_EDGE ( 'NONE', *, *, #13820, .F. ) ;
#18316=VECTOR ( 'NONE', #29813, 1000.000000000000000 ) ;
#18320=ORIENTED_EDGE ( 'NONE', *, *, #26567, .T. ) ;
#18321=CARTESIAN_POINT ( 'NONE',  ( 101.6614607007391982, -4.999999999999989342, 73.86137465823269110 ) ) ;
#18322=ORIENTED_EDGE ( 'NONE', *, *, #14691, .F. ) ;
#18324=VECTOR ( 'NONE', #2243, 1000.000000000000000 ) ;
#18327=ORIENTED_EDGE ( 'NONE', *, *, #5813, .F. ) ;
#18329=LINE ( 'NONE', #13155, #14506 ) ;
#18330=PLANE ( 'NONE',  #1584 ) ;
#18335=DIRECTION ( 'NONE',  ( 1.110223024625156540E-16, 2.995891024602366092E-32, 1.000000000000000000 ) ) ;
#18339=VECTOR ( 'NONE', #28661, 1000.000000000000000 ) ;
#18340=EDGE_CURVE ( 'NONE', #26457, #1081, #3569, .T. ) ;
#18342=DIRECTION ( 'NONE',  ( -0.5877852522924731371, -1.586114251531760728E-16, -0.8090169943749474513 ) ) ;
#18343=CARTESIAN_POINT ( 'NONE',  ( 19.02732395299416623, -5.000000000000012434, -58.56008168663054647 ) ) ;
#18344=AXIS2_PLACEMENT_3D ( 'NONE', #11339, #13187, #10887 ) ;
#18346=VECTOR ( 'NONE', #13466, 1000.000000000000000 ) ;
#18355=CARTESIAN_POINT ( 'NONE',  ( 72.52133520196026950, -4.999999999999997335, 52.68983421195638073 ) ) ;
#18358=ORIENTED_EDGE ( 'NONE', *, *, #21938, .T. ) ;
#18359=EDGE_LOOP ( 'NONE', ( #18139, #15204, #24906, #27755 ) ) ;
#18360=LINE ( 'NONE', #20346, #16361 ) ;
#18363=LINE ( 'NONE', #2211, #8813 ) ;
#18364=VECTOR ( 'NONE', #25703, 1000.000000000000000 ) ;
#18365=CARTESIAN_POINT ( 'NONE',  ( 176.1922820468852535, -9.999999999999994671, -2.083034168790677043 ) ) ;
#18366=EDGE_CURVE ( 'NONE', #25049, #22665, #23647, .T. ) ;
#18368=EDGE_LOOP ( 'NONE', ( #274, #16294, #24848, #24470 ) ) ;
#18369=LINE ( 'NONE', #18678, #2291 ) ;
#18372=AXIS2_PLACEMENT_3D ( 'NONE', #3219, #15081, #19373 ) ;
#18376=LINE ( 'NONE', #6793, #13164 ) ;
#18377=EDGE_CURVE ( 'NONE', #19537, #9002, #2748, .T. ) ;
#18379=EDGE_CURVE ( 'NONE', #2523, #19537, #9433, .T. ) ;
#18380=CARTESIAN_POINT ( 'NONE',  ( 156.1922820468853672, -10.00000000000000000, -10.74328820663507678 ) ) ;
#18381=ORIENTED_EDGE ( 'NONE', *, *, #1450, .F. ) ;
#18382=EDGE_CURVE ( 'NONE', #30249, #3306, #11731, .T. ) ;
#18383=FACE_OUTER_BOUND ( 'NONE', #7992, .T. ) ;
#18384=DIRECTION ( 'NONE',  ( -1.110223024625156540E-16, 0.000000000000000000, -1.000000000000000000 ) ) ;
#18386=VECTOR ( 'NONE', #24911, 1000.000000000000000 ) ;
#18393=VECTOR ( 'NONE', #14077, 1000.000000000000000 ) ;
#18396=PLANE ( 'NONE',  #12447 ) ;
#18398=DIRECTION ( 'NONE',  ( 1.110223024625156540E-16, 2.995891024602366092E-32, 1.000000000000000000 ) ) ;
#18400=VERTEX_POINT ( 'NONE', #2602 ) ;
#18401=LINE ( 'NONE', #27753, #2272 ) ;
#18403=VECTOR ( 'NONE', #20771, 1000.000000000000000 ) ;
#18405=LINE ( 'NONE', #16110, #7606 ) ;
#18414=VECTOR ( 'NONE', #24572, 1000.000000000000000 ) ;
#18415=CARTESIAN_POINT ( 'NONE',  ( 154.7287565553230024, -1.999999999999974021, -25.16025403784440329 ) ) ;
#18418=EDGE_CURVE ( 'NONE', #24045, #17748, #455, .T. ) ;
#18419=ORIENTED_EDGE ( 'NONE', *, *, #1589, .F. ) ;
#18421=CARTESIAN_POINT ( 'NONE',  ( 166.1922820468853672, -9.999999999999996447, -30.91696583120936026 ) ) ;
#18422=EDGE_CURVE ( 'NONE', #319, #30249, #7317, .T. ) ;
#18423=DIRECTION ( 'NONE',  ( -2.698458740408365879E-16, 1.000000000000000000, 0.000000000000000000 ) ) ;
#18424=EDGE_LOOP ( 'NONE', ( #5048, #28668, #12810, #24213 ) ) ;
#18425=ORIENTED_EDGE ( 'NONE', *, *, #23993, .F. ) ;
#18426=FACE_OUTER_BOUND ( 'NONE', #1656, .T. ) ;
#18427=FACE_OUTER_BOUND ( 'NONE', #29539, .T. ) ;
#18428=ORIENTED_EDGE ( 'NONE', *, *, #15753, .F. ) ;
#18431=ORIENTED_EDGE ( 'NONE', *, *, #18377, .F. ) ;
#18432=VECTOR ( 'NONE', #24003, 1000.000000000000000 ) ;
#18434=DIRECTION ( 'NONE',  ( 1.000000000000000000, 2.698458740408365879E-16, -1.110223024625156540E-16 ) ) ;
#18436=DIRECTION ( 'NONE',  ( -2.698458740408365879E-16, 1.000000000000000000, 0.000000000000000000 ) ) ;
#18437=CARTESIAN_POINT ( 'NONE',  ( 72.09850868606311280, -4.999999999999998224, 52.38263276618876318 ) ) ;
#18438=ORIENTED_EDGE ( 'NONE', *, *, #24524, .F. ) ;
#18440=FACE_OUTER_BOUND ( 'NONE', #1702, .T. ) ;
#18441=CARTESIAN_POINT ( 'NONE',  ( 87.30281120929834060, -4.999999999999993783, 63.42920515797836600 ) ) ;
#18445=VECTOR ( 'NONE', #15440, 1000.000000000000000 ) ;
#18446=ORIENTED_EDGE ( 'NONE', *, *, #14952, .F. ) ;
#18448=EDGE_CURVE ( 'NONE', #6539, #3010, #28265, .T. ) ;
#18452=LINE ( 'NONE', #5013, #16467 ) ;
#18453=PLANE ( 'NONE',  #7724 ) ;
#18458=CARTESIAN_POINT ( 'NONE',  ( 10.36273093427488590, -5.000000000000015099, 31.89320639659453605 ) ) ;
#18460=VECTOR ( 'NONE', #28263, 1000.000000000000000 ) ;
#18464=CARTESIAN_POINT ( 'NONE',  ( 131.1922820468854241, -1.999999999999982236, -13.59645775552055547 ) ) ;
#18465=ORIENTED_EDGE ( 'NONE', *, *, #15235, .T. ) ;
#18466=ORIENTED_EDGE ( 'NONE', *, *, #18593, .T. ) ;
#18472=VERTEX_POINT ( 'NONE', #11020 ) ;
#18475=LINE ( 'NONE', #18776, #28351 ) ;
#18476=DIRECTION ( 'NONE',  ( 0.9510565162951536422, 2.566386769018988816E-16, 0.3090169943749472292 ) ) ;
#18479=ORIENTED_EDGE ( 'NONE', *, *, #25580, .T. ) ;
#18481=EDGE_CURVE ( 'NONE', #27442, #966, #7172, .T. ) ;
#18485=EDGE_LOOP ( 'NONE', ( #12311, #16938, #11802, #4191 ) ) ;
#18486=ADVANCED_FACE ( 'NONE', ( #23493 ), #11877, .T. ) ;
#18487=DIRECTION ( 'NONE',  ( 1.110223024625156540E-16, 2.995891024602366092E-32, 1.000000000000000000 ) ) ;
#18489=CARTESIAN_POINT ( 'NONE',  ( 153.6922820468853388, -1.999999999999976241, -0.6060766987539614181 ) ) ;
#18495=LINE ( 'NONE', #27850, #11804 ) ;
#18496=DIRECTION ( 'NONE',  ( 0.000000000000000000, -1.000000000000000000, 0.000000000000000000 ) ) ;
#18497=VECTOR ( 'NONE', #21653, 1000.000000000000000 ) ;
#18498=CARTESIAN_POINT ( 'NONE',  ( 176.1922820468852819, -1.999999999999969580, -10.74328820663507678 ) ) ;
#18499=CARTESIAN_POINT ( 'NONE',  ( 6.862631103873988891, -5.000000000000015987, 21.12100677009980032 ) ) ;
#18502=CONICAL_SURFACE ( 'NONE', #7794, 5.999999999999977796, 0.7853981633974509435 ) ;
#18503=DIRECTION ( 'NONE',  ( -0.9510565162951536422, -2.566386769018988816E-16, -0.3090169943749472292 ) ) ;
#18505=DIRECTION ( 'NONE',  ( 1.000000000000000000, 2.698458740408365879E-16, -1.110223024625156540E-16 ) ) ;
#18506=ORIENTED_EDGE ( 'NONE', *, *, #28034, .F. ) ;
#18508=ORIENTED_EDGE ( 'NONE', *, *, #10653, .F. ) ;
#18510=CARTESIAN_POINT ( 'NONE',  ( 4.952801047623463404, -5.000000000000015987, 15.24315424717507206 ) ) ;
#18511=CARTESIAN_POINT ( 'NONE',  ( 98.27884857356201564, -4.999999999999990230, 71.40376309209180761 ) ) ;
#18513=ORIENTED_EDGE ( 'NONE', *, *, #15689, .T. ) ;
#18514=ORIENTED_EDGE ( 'NONE', *, *, #20669, .T. ) ;
#18515=LINE ( 'NONE', #11191, #332 ) ;
#18517=VERTEX_POINT ( 'NONE', #18912 ) ;
#18520=CARTESIAN_POINT ( 'NONE',  ( 175.7287565553229456, -4.999999999999970690, 3.500000000000003109 ) ) ;
#18522=DIRECTION ( 'NONE',  ( 0.9510565162951535312, 2.566386769018988816E-16, -0.3090169943749475623 ) ) ;
#18525=ORIENTED_EDGE ( 'NONE', *, *, #19061, .T. ) ;
#18527=LINE ( 'NONE', #6631, #7159 ) ;
#18529=VECTOR ( 'NONE', #4482, 1000.000000000000000 ) ;
#18532=ORIENTED_EDGE ( 'NONE', *, *, #17070, .F. ) ;
#18535=AXIS2_PLACEMENT_3D ( 'NONE', #23583, #2840, #18545 ) ;
#18536=DIRECTION ( 'NONE',  ( 0.5877852522924731371, 0.000000000000000000, 0.8090169943749474513 ) ) ;
#18543=VECTOR ( 'NONE', #6533, 1000.000000000000000 ) ;
#18545=DIRECTION ( 'NONE',  ( 0.9510565162951536422, 0.000000000000000000, -0.3090169943749475623 ) ) ;
#18546=LINE ( 'NONE', #20982, #24934 ) ;
#18547=CARTESIAN_POINT ( 'NONE',  ( 147.2287565553230024, -1.999999999999976685, -12.16987298107780369 ) ) ;
#18550=PLANE ( 'NONE',  #22231 ) ;
#18552=VERTEX_POINT ( 'NONE', #7020 ) ;
#18555=EDGE_CURVE ( 'NONE', #13963, #10847, #4578, .T. ) ;
#18557=EDGE_CURVE ( 'NONE', #28590, #23545, #2, .T. ) ;
#18559=EDGE_CURVE ( 'NONE', #3628, #15830, #28559, .T. ) ;
#18560=ORIENTED_EDGE ( 'NONE', *, *, #14021, .T. ) ;
#18561=EDGE_CURVE ( 'NONE', #29468, #15766, #28714, .T. ) ;
#18563=AXIS2_PLACEMENT_3D ( 'NONE', #18582, #25593, #7444 ) ;
#18565=VECTOR ( 'NONE', #10789, 1000.000000000000000 ) ;
#18567=ORIENTED_EDGE ( 'NONE', *, *, #4401, .F. ) ;
#18568=CARTESIAN_POINT ( 'NONE',  ( 8.851409776105752414, -5.000000000000015099, 27.24183814871275544 ) ) ;
#18572=PLANE ( 'NONE',  #10377 ) ;
#18573=CARTESIAN_POINT ( 'NONE',  ( 144.7287565553229740, -10.00000000000000533, 0.8205080756887930260 ) ) ;
#18574=ORIENTED_EDGE ( 'NONE', *, *, #13349, .F. ) ;
#18575=ORIENTED_EDGE ( 'NONE', *, *, #22136, .F. ) ;
#18576=CARTESIAN_POINT ( 'NONE',  ( 133.6922820468854241, -1.999999999999981348, -9.266330736598357376 ) ) ;
#18582=CARTESIAN_POINT ( 'NONE',  ( 153.6922820468853388, -10.00000000000000178, -15.07341522555727309 ) ) ;
#18583=DIRECTION ( 'NONE',  ( 1.000000000000000000, 2.698458740408365879E-16, -1.110223024625156540E-16 ) ) ;
#18585=CARTESIAN_POINT ( 'NONE',  ( 147.2287565553229740, -1.999999999999977129, -3.509618943233403510 ) ) ;
#18586=LINE ( 'NONE', #11266, #20732 ) ;
#18587=VERTEX_POINT ( 'NONE', #3204 ) ;
#18589=EDGE_CURVE ( 'NONE', #4293, #12466, #3055, .T. ) ;
#18590=LINE ( 'NONE', #17346, #2004 ) ;
#18591=VERTEX_POINT ( 'NONE', #19353 ) ;
#18592=VERTEX_POINT ( 'NONE', #7613 ) ;
#18593=EDGE_CURVE ( 'NONE', #29723, #2898, #29165, .T. ) ;
#18595=ORIENTED_EDGE ( 'NONE', *, *, #23169, .T. ) ;
#18596=EDGE_CURVE ( 'NONE', #18615, #18805, #10493, .T. ) ;
#18602=DIRECTION ( 'NONE',  ( -2.698458740408365879E-16, 1.000000000000000000, 0.000000000000000000 ) ) ;
#18603=CARTESIAN_POINT ( 'NONE',  ( 163.6922820468852819, -9.999999999999998224, 2.247092850131519715 ) ) ;
#18607=DIRECTION ( 'NONE',  ( -2.698458740408365879E-16, 1.000000000000000000, 0.000000000000000000 ) ) ;
#18608=LINE ( 'NONE', #26093, #15219 ) ;
#18609=VECTOR ( 'NONE', #26628, 1000.000000000000000 ) ;
#18610=DIRECTION ( 'NONE',  ( -0.9510565162951536422, -2.566386769018988323E-16, 0.3090169943749475623 ) ) ;
#18611=DIRECTION ( 'NONE',  ( 1.110223024625156540E-16, 2.995891024602366092E-32, 1.000000000000000000 ) ) ;
#18615=VERTEX_POINT ( 'NONE', #23966 ) ;
#18619=VERTEX_POINT ( 'NONE', #7762 ) ;
#18620=PLANE ( 'NONE',  #264 ) ;
#18626=ORIENTED_EDGE ( 'NONE', *, *, #13891, .F. ) ;
#18627=ORIENTED_EDGE ( 'NONE', *, *, #10098, .T. ) ;
#18631=PLANE ( 'NONE',  #28855 ) ;
#18632=LINE ( 'NONE', #26114, #28675 ) ;
#18633=VERTEX_POINT ( 'NONE', #604 ) ;
#18634=ORIENTED_EDGE ( 'NONE', *, *, #14822, .F. ) ;
#18636=ORIENTED_EDGE ( 'NONE', *, *, #8242, .F. ) ;
#18637=EDGE_CURVE ( 'NONE', #24640, #28929, #12183, .T. ) ;
#18639=ORIENTED_EDGE ( 'NONE', *, *, #27218, .T. ) ;
#18642=AXIS2_PLACEMENT_3D ( 'NONE', #18038, #2041, #20628 ) ;
#18644=VERTEX_POINT ( 'NONE', #28878 ) ;
#18650=EDGE_LOOP ( 'NONE', ( #18789, #19410, #9378, #16316 ) ) ;
#18651=CARTESIAN_POINT ( 'NONE',  ( 139.7287565553230024, -4.999999999999979572, 0.8205080756887861426 ) ) ;
#18652=ORIENTED_EDGE ( 'NONE', *, *, #13817, .F. ) ;
#18656=EDGE_CURVE ( 'NONE', #29392, #20051, #26401, .T. ) ;
#18657=CARTESIAN_POINT ( 'NONE',  ( 146.1922820468854241, -1.999999999999977573, -13.59645775552055902 ) ) ;
#18662=ORIENTED_EDGE ( 'NONE', *, *, #9684, .T. ) ;
#18664=ORIENTED_EDGE ( 'NONE', *, *, #7535, .T. ) ;
#18667=LINE ( 'NONE', #11781, #20972 ) ;
#18668=CARTESIAN_POINT ( 'NONE',  ( 148.6922820468854525, -10.00000000000000178, -26.58683881228715862 ) ) ;
#18670=EDGE_LOOP ( 'NONE', ( #7528, #27861, #29527, #3089, #19074 ) ) ;
#18671=PLANE ( 'NONE',  #16886 ) ;
#18674=CARTESIAN_POINT ( 'NONE',  ( 174.5152310637604671, -1.999999999999968914, -30.37205893520531319 ) ) ;
#18677=VERTEX_POINT ( 'NONE', #14467 ) ;
#18678=CARTESIAN_POINT ( 'NONE',  ( 5.907716075748727036, -5.000000000000015987, 18.18208050863744063 ) ) ;
#18685=VECTOR ( 'NONE', #28798, 1000.000000000000000 ) ;
#18686=CARTESIAN_POINT ( 'NONE',  ( 75.79387768789761992, -4.999999999999996447, 55.06747550269425773 ) ) ;
#18687=ORIENTED_EDGE ( 'NONE', *, *, #10697, .T. ) ;
#18688=EDGE_CURVE ( 'NONE', #2298, #17680, #26550, .T. ) ;
#18689=EDGE_CURVE ( 'NONE', #21176, #24060, #19805, .T. ) ;
#18692=EDGE_CURVE ( 'NONE', #28015, #15364, #3352, .T. ) ;
#18693=CARTESIAN_POINT ( 'NONE',  ( 136.1922820468854241, -1.999999999999980460, -13.59645775552055547 ) ) ;
#18694=EDGE_CURVE ( 'NONE', #11084, #8715, #23806, .T. ) ;
#18701=LINE ( 'NONE', #25727, #10298 ) ;
#18702=CARTESIAN_POINT ( 'NONE',  ( 151.1922820468853672, -1.999999999999976685, -4.936203717676158398 ) ) ;
#18704=VERTEX_POINT ( 'NONE', #14616 ) ;
#18705=CARTESIAN_POINT ( 'NONE',  ( 127.7287565553229740, -1.999999999999982681, 0.5000000000000115463 ) ) ;
#18710=CARTESIAN_POINT ( 'NONE',  ( 147.0152310637606092, -10.00000000000000178, -32.93883019725009120 ) ) ;
#18719=ORIENTED_EDGE ( 'NONE', *, *, #4090, .F. ) ;
#18721=EDGE_CURVE ( 'NONE', #9848, #8637, #9892, .T. ) ;
#18723=VERTEX_POINT ( 'NONE', #3501 ) ;
#18724=VERTEX_POINT ( 'NONE', #10345 ) ;
#18725=ADVANCED_FACE ( 'NONE', ( #12791 ), #22105, .T. ) ;
#18727=VECTOR ( 'NONE', #1178, 1000.000000000000000 ) ;
#18729=CARTESIAN_POINT ( 'NONE',  ( 11.55449181034387962, -5.000000000000014211, 35.56106922512162782 ) ) ;
#18733=DIRECTION ( 'NONE',  ( 0.9510565162951536422, 2.566386769018988816E-16, 0.3090169943749472292 ) ) ;
#18735=AXIS2_PLACEMENT_3D ( 'NONE', #4917, #23390, #9787 ) ;
#18738=CARTESIAN_POINT ( 'NONE',  ( 20.53864511116330149, -5.000000000000012434, -63.21144993451233063 ) ) ;
#18739=VERTEX_POINT ( 'NONE', #1669 ) ;
#18741=DIRECTION ( 'NONE',  ( -2.698458740408365879E-16, 1.000000000000000000, 0.000000000000000000 ) ) ;
#18742=DIRECTION ( 'NONE',  ( -2.698458740408365879E-16, 1.000000000000000000, 0.000000000000000000 ) ) ;
#18743=ORIENTED_EDGE ( 'NONE', *, *, #6986, .F. ) ;
#18749=DIRECTION ( 'NONE',  ( -0.9510565162951536422, -2.566386769018988323E-16, 0.3090169943749475623 ) ) ;
#18751=DIRECTION ( 'NONE',  ( 0.9510565162951535312, 2.566386769018988816E-16, -0.3090169943749475623 ) ) ;
#18753=LINE ( 'NONE', #23333, #27656 ) ;
#18754=PLANE ( 'NONE',  #12789 ) ;
#18763=ORIENTED_EDGE ( 'NONE', *, *, #17248, .F. ) ;
#18765=ORIENTED_EDGE ( 'NONE', *, *, #26020, .F. ) ;
#18766=LINE ( 'NONE', #4878, #1244 ) ;
#18767=VECTOR ( 'NONE', #8698, 1000.000000000000000 ) ;
#18770=CARTESIAN_POINT ( 'NONE',  ( 143.6922820468854241, -1.999999999999978462, -15.07341522555727664 ) ) ;
#18771=ORIENTED_EDGE ( 'NONE', *, *, #13655, .F. ) ;
#18772=ORIENTED_EDGE ( 'NONE', *, *, #17587, .T. ) ;
#18774=LINE ( 'NONE', #170, #28695 ) ;
#18776=CARTESIAN_POINT ( 'NONE',  ( 134.5152310637605808, -1.999999999999980460, -19.94844914048349338 ) ) ;
#18779=ORIENTED_EDGE ( 'NONE', *, *, #20074, .T. ) ;
#18781=VERTEX_POINT ( 'NONE', #13542 ) ;
#18783=EDGE_LOOP ( 'NONE', ( #25402, #29546, #7100, #18446 ) ) ;
#18787=ORIENTED_EDGE ( 'NONE', *, *, #12594, .T. ) ;
#18788=PLANE ( 'NONE',  #9136 ) ;
#18789=ORIENTED_EDGE ( 'NONE', *, *, #12215, .T. ) ;
#18794=VERTEX_POINT ( 'NONE', #1520 ) ;
#18796=ADVANCED_FACE ( 'NONE', ( #24553 ), #13392, .T. ) ;
#18799=LINE ( 'NONE', #11916, #21399 ) ;
#18800=PLANE ( 'NONE',  #19264 ) ;
#18804=DIRECTION ( 'NONE',  ( 1.000000000000000000, 2.698458740408365879E-16, -1.110223024625156540E-16 ) ) ;
#18805=VERTEX_POINT ( 'NONE', #27337 ) ;
#18806=VECTOR ( 'NONE', #2552, 1000.000000000000000 ) ;
#18808=VERTEX_POINT ( 'NONE', #17810 ) ;
#18812=DIRECTION ( 'NONE',  ( -2.698458740408365879E-16, 1.000000000000000000, 0.000000000000000000 ) ) ;
#18816=ORIENTED_EDGE ( 'NONE', *, *, #18561, .T. ) ;
#18818=DIRECTION ( 'NONE',  ( 2.908569913943825554E-16, -1.000000000000000000, 0.000000000000000000 ) ) ;
#18819=CARTESIAN_POINT ( 'NONE',  ( 138.6922820468854525, -10.00000000000000533, -23.73366926340167282 ) ) ;
#18821=ORIENTED_EDGE ( 'NONE', *, *, #18201, .F. ) ;
#18828=EDGE_LOOP ( 'NONE', ( #21847, #2139, #22647, #12898, #12739 ) ) ;
#18829=CARTESIAN_POINT ( 'NONE',  ( 159.7287565553229456, -1.999999999999973133, -16.50000000000000355 ) ) ;
#18832=CARTESIAN_POINT ( 'NONE',  ( 163.6922820468852819, -1.999999999999973577, -0.6060766987539614181 ) ) ;
#18833=CARTESIAN_POINT ( 'NONE',  ( 87.79094120493316211, -4.999999999999993783, -63.78385235900214667 ) ) ;
#18834=CARTESIAN_POINT ( 'NONE',  ( 133.7287565553229172, -9.999999999999980460, -33.50000000000000000 ) ) ;
#18836=ORIENTED_EDGE ( 'NONE', *, *, #24527, .F. ) ;
#18842=DIRECTION ( 'NONE',  ( -2.698458740408365879E-16, 1.000000000000000000, 0.000000000000000000 ) ) ;
#18844=VECTOR ( 'NONE', #10110, 1000.000000000000000 ) ;
#18848=ORIENTED_EDGE ( 'NONE', *, *, #9021, .F. ) ;
#18849=CARTESIAN_POINT ( 'NONE',  ( 132.0152310637605524, -1.999999999999981348, -17.38167787843870826 ) ) ;
#18851=EDGE_LOOP ( 'NONE', ( #17983, #10169, #25695, #9992, #265 ) ) ;
#18852=AXIS2_PLACEMENT_3D ( 'NONE', #25960, #9612, #14186 ) ;
#18853=LINE ( 'NONE', #2847, #15399 ) ;
#18854=DIRECTION ( 'NONE',  ( -0.5877852522924731371, -1.586114251531760728E-16, -0.8090169943749474513 ) ) ;
#18855=VECTOR ( 'NONE', #8402, 1000.000000000000000 ) ;
#18859=VERTEX_POINT ( 'NONE', #29333 ) ;
#18861=ADVANCED_FACE ( 'NONE', ( #13250 ), #22866, .T. ) ;
#18862=EDGE_CURVE ( 'NONE', #28921, #11253, #17669, .T. ) ;
#18863=VECTOR ( 'NONE', #3719, 1000.000000000000000 ) ;
#18865=ADVANCED_FACE ( 'NONE', ( #15532 ), #8948, .T. ) ;
#18868=VECTOR ( 'NONE', #12995, 1000.000000000000000 ) ;
#18870=DIRECTION ( 'NONE',  ( -2.698458740408365879E-16, 1.000000000000000000, 0.000000000000000000 ) ) ;
#18872=AXIS2_PLACEMENT_3D ( 'NONE', #21258, #2524, #24023 ) ;
#18873=DIRECTION ( 'NONE',  ( -2.698458740408365879E-16, 1.000000000000000000, 0.000000000000000000 ) ) ;
#18880=DIRECTION ( 'NONE',  ( -2.698458740408365879E-16, 1.000000000000000000, 0.000000000000000000 ) ) ;
#18883=LINE ( 'NONE', #585, #12945 ) ;
#18884=EDGE_CURVE ( 'NONE', #17616, #600, #3799, .T. ) ;
#18885=VERTEX_POINT ( 'NONE', #5937 ) ;
#18887=DIRECTION ( 'NONE',  ( 0.9510565162951536422, 2.566386769018988816E-16, 0.3090169943749472292 ) ) ;
#18888=VECTOR ( 'NONE', #7629, 1000.000000000000000 ) ;
#18890=VERTEX_POINT ( 'NONE', #1823 ) ;
#18891=DIRECTION ( 'NONE',  ( 6.938893903907227392E-16, -0.000000000000000000, 1.000000000000000000 ) ) ;
#18894=EDGE_CURVE ( 'NONE', #30251, #10208, #1363, .T. ) ;
#18897=EDGE_CURVE ( 'NONE', #3561, #17674, #20406, .T. ) ;
#18898=ADVANCED_FACE ( 'NONE', ( #27180 ), #15680, .T. ) ;
#18901=DIRECTION ( 'NONE',  ( -2.698458740408365879E-16, 1.000000000000000000, 0.000000000000000000 ) ) ;
#18902=EDGE_CURVE ( 'NONE', #11106, #6687, #8808, .T. ) ;
#18903=CARTESIAN_POINT ( 'NONE',  ( 174.5152310637604387, -4.999999999999970690, -11.28819510263909542 ) ) ;
#18906=ORIENTED_EDGE ( 'NONE', *, *, #11426, .T. ) ;
#18907=CARTESIAN_POINT ( 'NONE',  ( 157.0152310637605808, -9.999999999999998224, -32.93883019725009120 ) ) ;
#18908=LINE ( 'NONE', #23644, #4993 ) ;
#18909=CARTESIAN_POINT ( 'NONE',  ( 101.3039376645797347, -4.999999999999989342, -73.60161896772125090 ) ) ;
#18911=DIRECTION ( 'NONE',  ( -0.9510565162951536422, 0.000000000000000000, -0.3090169943749472292 ) ) ;
#18912=CARTESIAN_POINT ( 'NONE',  ( 132.0152310637605808, -4.999999999999982236, -15.61832212156129351 ) ) ;
#18915=CARTESIAN_POINT ( 'NONE',  ( 130.7287565553229172, -4.999999999999982236, -2.233642730705378998 ) ) ;
#18916=VECTOR ( 'NONE', #8534, 1000.000000000000000 ) ;
#18917=ORIENTED_EDGE ( 'NONE', *, *, #26706, .F. ) ;
#18919=ORIENTED_EDGE ( 'NONE', *, *, #13945, .F. ) ;
#18923=CARTESIAN_POINT ( 'NONE',  ( 10.99808568030000444, -5.000000000000015099, 33.84862723870220691 ) ) ;
#18924=ORIENTED_EDGE ( 'NONE', *, *, #5370, .T. ) ;
#18925=ORIENTED_EDGE ( 'NONE', *, *, #28285, .T. ) ;
#18927=CARTESIAN_POINT ( 'NONE',  ( 153.6922820468853388, -10.00000000000000178, -17.92658477444275533 ) ) ;
#18929=DIRECTION ( 'NONE',  ( 1.000000000000000000, 2.698458740408365879E-16, -1.110223024625156540E-16 ) ) ;
#18931=ORIENTED_EDGE ( 'NONE', *, *, #19310, .F. ) ;
#18933=ORIENTED_EDGE ( 'NONE', *, *, #11317, .F. ) ;
#18935=ORIENTED_EDGE ( 'NONE', *, *, #8623, .F. ) ;
#18939=EDGE_CURVE ( 'NONE', #23167, #26513, #2707, .T. ) ;
#18940=PLANE ( 'NONE',  #2839 ) ;
#18941=EDGE_CURVE ( 'NONE', #10103, #16958, #4988, .T. ) ;
#18942=EDGE_CURVE ( 'NONE', #4384, #20699, #28075, .T. ) ;
#18943=EDGE_CURVE ( 'NONE', #4151, #22156, #2572, .T. ) ;
#18950=FACE_BOUND ( 'NONE', #26264, .T. ) ;
#18951=VECTOR ( 'NONE', #23968, 1000.000000000000000 ) ;
#18952=CARTESIAN_POINT ( 'NONE',  ( 151.1922820468853956, -1.999999999999976241, -13.59645775552055902 ) ) ;
#18953=CARTESIAN_POINT ( 'NONE',  ( 133.7287565553229172, -4.000000000000003553, -33.50000000000000000 ) ) ;
#18954=CARTESIAN_POINT ( 'NONE',  ( 174.5152310637604671, -4.999999999999970690, -1.937508276747662207E-14 ) ) ;
#18957=CARTESIAN_POINT ( 'NONE',  ( 162.2287565553228887, -1.999999999999973133, -3.509618943233403510 ) ) ;
#18958=VECTOR ( 'NONE', #3100, 1000.000000000000000 ) ;
#18959=CARTESIAN_POINT ( 'NONE',  ( 161.1922820468853956, -4.999999999999973355, -28.06379628232387802 ) ) ;
#18960=EDGE_LOOP ( 'NONE', ( #25568, #9189, #13352, #18771 ) ) ;
#18965=DIRECTION ( 'NONE',  ( -2.698458740408365879E-16, 1.000000000000000000, 0.000000000000000000 ) ) ;
#18966=CARTESIAN_POINT ( 'NONE',  ( 133.7287565553229740, -84.33034373659253902, 8.500000000000003553 ) ) ;
#18968=AXIS2_PLACEMENT_3D ( 'NONE', #24852, #22405, #10798 ) ;
#18969=ORIENTED_EDGE ( 'NONE', *, *, #374, .T. ) ;
#18970=DIRECTION ( 'NONE',  ( -0.5877852522924731371, -1.586114251531760728E-16, -0.8090169943749474513 ) ) ;
#18974=CARTESIAN_POINT ( 'NONE',  ( 133.6922820468854241, -4.999999999999982236, -35.24709285013155835 ) ) ;
#18975=ORIENTED_EDGE ( 'NONE', *, *, #5508, .T. ) ;
#18976=EDGE_CURVE ( 'NONE', #14016, #20426, #2419, .T. ) ;
#18977=LINE ( 'NONE', #521, #20824 ) ;
#18980=EDGE_CURVE ( 'NONE', #15766, #3931, #21311, .T. ) ;
#18981=ORIENTED_EDGE ( 'NONE', *, *, #28189, .F. ) ;
#18983=CARTESIAN_POINT ( 'NONE',  ( 142.0152310637606092, -4.999999999999979572, -32.93883019725009120 ) ) ;
#18987=ORIENTED_EDGE ( 'NONE', *, *, #19402, .T. ) ;
#18989=VECTOR ( 'NONE', #278, 1000.000000000000000 ) ;
#18990=DIRECTION ( 'NONE',  ( 0.5877852522924731371, 1.586114251531760728E-16, -0.8090169943749474513 ) ) ;
#18992=DIRECTION ( 'NONE',  ( 1.110223024625156540E-16, 2.995891024602366092E-32, 1.000000000000000000 ) ) ;
#18993=CARTESIAN_POINT ( 'NONE',  ( 157.0152310637605808, -1.999999999999973133, -32.93883019725009120 ) ) ;
#18994=DIRECTION ( 'NONE',  ( 1.110223024625156540E-16, 2.995891024602366092E-32, 1.000000000000000000 ) ) ;
#18998=ADVANCED_FACE ( 'NONE', ( #11993 ), #25450, .T. ) ;
#19000=EDGE_LOOP ( 'NONE', ( #24586, #13434, #9659, #10022 ) ) ;
#19001=LINE ( 'NONE', #11817, #30078 ) ;
#19002=CARTESIAN_POINT ( 'NONE',  ( 18.62881505491278489, -5.000000000000012434, -57.33359741158763256 ) ) ;
#19003=CARTESIAN_POINT ( 'NONE',  ( 148.6922820468853672, -10.00000000000000355, 2.247092850131519715 ) ) ;
#19004=LINE ( 'NONE', #19151, #7581 ) ;
#19006=ORIENTED_EDGE ( 'NONE', *, *, #24360, .F. ) ;
#19007=LINE ( 'NONE', #16564, #28109 ) ;
#19009=VECTOR ( 'NONE', #21048, 1000.000000000000000 ) ;
#19010=FACE_OUTER_BOUND ( 'NONE', #1120, .T. ) ;
#19011=DIRECTION ( 'NONE',  ( 0.3090169943749475623, 8.338696094058001131E-17, 0.9510565162951536422 ) ) ;
#19013=ORIENTED_EDGE ( 'NONE', *, *, #11814, .T. ) ;
#19014=VECTOR ( 'NONE', #17555, 1000.000000000000000 ) ;
#19016=VECTOR ( 'NONE', #22530, 1000.000000000000000 ) ;
#19017=ORIENTED_EDGE ( 'NONE', *, *, #4534, .F. ) ;
#19022=VECTOR ( 'NONE', #1750, 1000.000000000000000 ) ;
#19023=VERTEX_POINT ( 'NONE', #11539 ) ;
#19024=EDGE_LOOP ( 'NONE', ( #24573, #29145, #27519, #15369 ) ) ;
#19025=CARTESIAN_POINT ( 'NONE',  ( 154.5152310637605524, -1.999999999999974465, -19.94844914048349693 ) ) ;
#19026=FACE_OUTER_BOUND ( 'NONE', #27367, .T. ) ;
#19027=CARTESIAN_POINT ( 'NONE',  ( 154.5152310637604955, -10.00000000000000178, -2.627941064794695691 ) ) ;
#19028=DIRECTION ( 'NONE',  ( 0.5877852522924731371, 0.000000000000000000, 0.8090169943749474513 ) ) ;
#19032=EDGE_LOOP ( 'NONE', ( #18560, #18425, #17729, #16195 ) ) ;
#19033=LINE ( 'NONE', #6847, #12710 ) ;
#19034=CARTESIAN_POINT ( 'NONE',  ( 148.6922820468854525, -1.999999999999976241, -35.24709285013155835 ) ) ;
#19036=CARTESIAN_POINT ( 'NONE',  ( 137.0152310637605808, -4.999999999999980460, 1.702185954127501066 ) ) ;
#19037=CARTESIAN_POINT ( 'NONE',  ( 132.0152310637605524, -1.999999999999981348, -17.38167787843870826 ) ) ;
#19038=VECTOR ( 'NONE', #23786, 1000.000000000000000 ) ;
#19039=EDGE_LOOP ( 'NONE', ( #24324, #30255, #22041, #13731 ) ) ;
#19040=VECTOR ( 'NONE', #172, 999.9999999999998863 ) ;
#19041=DIRECTION ( 'NONE',  ( 0.5877852522924731371, 0.000000000000000000, 0.8090169943749474513 ) ) ;
#19042=ORIENTED_EDGE ( 'NONE', *, *, #7571, .T. ) ;
#19043=CARTESIAN_POINT ( 'NONE',  ( 167.2287565553228887, -1.999999999999971800, -3.509618943233403510 ) ) ;
#19044=VERTEX_POINT ( 'NONE', #18576 ) ;
#19051=LINE ( 'NONE', #25779, #15523 ) ;
#19052=CARTESIAN_POINT ( 'NONE',  ( 152.0152310637604955, -1.999999999999975797, -8.721423840594312082 ) ) ;
#19053=CARTESIAN_POINT ( 'NONE',  ( 173.6922820468852819, -4.999999999999971578, -9.266330736598359152 ) ) ;
#19055=DIRECTION ( 'NONE',  ( 0.3090169943749472292, 8.338696094057992503E-17, -0.9510565162951536422 ) ) ;
#19056=DIRECTION ( 'NONE',  ( -2.698458740408365879E-16, 1.000000000000000000, -0.000000000000000000 ) ) ;
#19057=VECTOR ( 'NONE', #11675, 1000.000000000000000 ) ;
#19061=EDGE_CURVE ( 'NONE', #28345, #14964, #27925, .T. ) ;
#19062=ADVANCED_FACE ( 'NONE', ( #25305 ), #6985, .T. ) ;
#19063=DIRECTION ( 'NONE',  ( -2.698458740408365879E-16, 1.000000000000000000, 0.000000000000000000 ) ) ;
#19065=ORIENTED_EDGE ( 'NONE', *, *, #19310, .T. ) ;
#19067=EDGE_CURVE ( 'NONE', #8041, #14150, #27623, .T. ) ;
#19068=VERTEX_POINT ( 'NONE', #20853 ) ;
#19069=DIRECTION ( 'NONE',  ( 0.9510565162951535312, 2.566386769018988816E-16, -0.3090169943749475623 ) ) ;
#19070=EDGE_CURVE ( 'NONE', #19198, #12834, #9248, .T. ) ;
#19073=DIRECTION ( 'NONE',  ( -0.9510565162951536422, -2.566386769018988323E-16, 0.3090169943749475623 ) ) ;
#19074=ORIENTED_EDGE ( 'NONE', *, *, #28317, .T. ) ;
#19075=ORIENTED_EDGE ( 'NONE', *, *, #12409, .T. ) ;
#19077=CARTESIAN_POINT ( 'NONE',  ( 148.6922820468854241, -10.00000000000000178, -15.07341522555727664 ) ) ;
#19080=ORIENTED_EDGE ( 'NONE', *, *, #23918, .T. ) ;
#19082=ORIENTED_EDGE ( 'NONE', *, *, #2755, .T. ) ;
#19089=CARTESIAN_POINT ( 'NONE',  ( 148.6922820468854241, -4.999999999999976907, -15.07341522555727664 ) ) ;
#19094=VERTEX_POINT ( 'NONE', #21012 ) ;
#19095=FACE_BOUND ( 'NONE', #24946, .T. ) ;
#19096=VECTOR ( 'NONE', #21040, 1000.000000000000000 ) ;
#19098=FACE_OUTER_BOUND ( 'NONE', #8846, .T. ) ;
#19099=DIRECTION ( 'NONE',  ( -0.8090169943749474513, -2.183098979609982436E-16, -0.5877852522924731371 ) ) ;
#19100=ADVANCED_FACE ( 'NONE', ( #11697 ), #25588, .T. ) ;
#19101=DIRECTION ( 'NONE',  ( -0.5877852522924731371, -1.586114251531760235E-16, 0.8090169943749474513 ) ) ;
#19102=ADVANCED_FACE ( 'NONE', ( #18426 ), #23019, .T. ) ;
#19103=ADVANCED_FACE ( 'NONE', ( #21155 ), #269, .T. ) ;
#19107=EDGE_LOOP ( 'NONE', ( #26847, #2762, #2984, #4095 ) ) ;
#19108=CARTESIAN_POINT ( 'NONE',  ( 156.1922820468854241, -10.00000000000000000, -30.91696583120936026 ) ) ;
#19109=VERTEX_POINT ( 'NONE', #14581 ) ;
#19114=CARTESIAN_POINT ( 'NONE',  ( 142.0152310637605808, -4.999999999999979572, -34.70218595412750773 ) ) ;
#19115=CARTESIAN_POINT ( 'NONE',  ( 164.5152310637604671, -4.999999999999973355, -2.627941064794695691 ) ) ;
#19118=VERTEX_POINT ( 'NONE', #26062 ) ;
#19121=CARTESIAN_POINT ( 'NONE',  ( 167.2287565553229172, -1.999999999999971356, -12.16987298107780369 ) ) ;
#19122=VECTOR ( 'NONE', #10030, 1000.000000000000000 ) ;
#19125=VERTEX_POINT ( 'NONE', #19471 ) ;
#19126=PLANE ( 'NONE',  #25196 ) ;
#19131=DIRECTION ( 'NONE',  ( 0.5877852522924731371, 1.586114251531760728E-16, 0.8090169943749474513 ) ) ;
#19132=AXIS2_PLACEMENT_3D ( 'NONE', #9430, #19055, #28107 ) ;
#19133=LINE ( 'NONE', #7840, #6520 ) ;
#19135=CARTESIAN_POINT ( 'NONE',  ( 133.7287565553229740, -84.33034373659253902, 0.5000000000000029976 ) ) ;
#19137=ADVANCED_FACE ( 'NONE', ( #28530 ), #872, .T. ) ;
#19138=CARTESIAN_POINT ( 'NONE',  ( 159.7287565553229740, -9.999999999999998224, -25.16025403784440329 ) ) ;
#19141=EDGE_CURVE ( 'NONE', #12198, #4291, #5296, .T. ) ;
#19143=ADVANCED_FACE ( 'NONE', ( #24221 ), #9861, .T. ) ;
#19147=ORIENTED_EDGE ( 'NONE', *, *, #19616, .F. ) ;
#19148=PLANE ( 'NONE',  #12973 ) ;
#19150=CARTESIAN_POINT ( 'NONE',  ( 172.7287565553229456, -9.999999999999980460, 0.5000000000000029976 ) ) ;
#19151=CARTESIAN_POINT ( 'NONE',  ( 152.2287565553229456, -1.999999999999975797, -3.509618943233403510 ) ) ;
#19153=ORIENTED_EDGE ( 'NONE', *, *, #2235, .F. ) ;
#19154=LINE ( 'NONE', #16408, #27627 ) ;
#19156=LINE ( 'NONE', #9530, #3717 ) ;
#19157=DIRECTION ( 'NONE',  ( 0.5877852522924731371, 1.586114251531760728E-16, -0.8090169943749474513 ) ) ;
#19158=VECTOR ( 'NONE', #17219, 1000.000000000000000 ) ;
#19161=ORIENTED_EDGE ( 'NONE', *, *, #27287, .F. ) ;
#19165=VECTOR ( 'NONE', #11099, 1000.000000000000000 ) ;
#19168=VERTEX_POINT ( 'NONE', #12752 ) ;
#19169=ORIENTED_EDGE ( 'NONE', *, *, #29830, .F. ) ;
#19173=EDGE_CURVE ( 'NONE', #13402, #26227, #7729, .T. ) ;
#19174=CARTESIAN_POINT ( 'NONE',  ( 116.5082401878149909, -4.999999999999985789, -84.64819135951087503 ) ) ;
#19178=AXIS2_PLACEMENT_3D ( 'NONE', #26947, #8577, #14991 ) ;
#19180=CARTESIAN_POINT ( 'NONE',  ( 99.12450160535630062, -4.999999999999990230, 72.01816598362702848 ) ) ;
#19183=FACE_OUTER_BOUND ( 'NONE', #16578, .T. ) ;
#19184=ORIENTED_EDGE ( 'NONE', *, *, #18063, .T. ) ;
#19185=LINE ( 'NONE', #3185, #27126 ) ;
#19186=DIRECTION ( 'NONE',  ( -0.9510565162951536422, -2.566386769018988323E-16, 0.3090169943749475623 ) ) ;
#19187=EDGE_LOOP ( 'NONE', ( #7386, #17533, #1991, #5610 ) ) ;
#19188=VERTEX_POINT ( 'NONE', #24071 ) ;
#19189=ORIENTED_EDGE ( 'NONE', *, *, #7876, .F. ) ;
#19193=FACE_OUTER_BOUND ( 'NONE', #7002, .T. ) ;
#19194=FACE_OUTER_BOUND ( 'NONE', #27225, .T. ) ;
#19196=EDGE_CURVE ( 'NONE', #15051, #8663, #2868, .T. ) ;
#19198=VERTEX_POINT ( 'NONE', #7579 ) ;
#19199=CARTESIAN_POINT ( 'NONE',  ( 142.0152310637605808, -10.00000000000000355, -6.958068083716895558 ) ) ;
#19200=CARTESIAN_POINT ( 'NONE',  ( 134.5152310637605808, -10.00000000000000533, -11.28819510263909187 ) ) ;
#19201=LINE ( 'NONE', #7315, #10178 ) ;
#19202=LINE ( 'NONE', #21643, #16096 ) ;
#19203=DIRECTION ( 'NONE',  ( -0.8090169943749474513, -2.183098979609982436E-16, -0.5877852522924731371 ) ) ;
#19206=CARTESIAN_POINT ( 'NONE',  ( 173.6922820468853672, -4.999999999999970690, -35.24709285013155835 ) ) ;
#19209=CARTESIAN_POINT ( 'NONE',  ( 141.1922820468854241, -1.999999999999979128, -4.936203717676158398 ) ) ;
#19213=VERTEX_POINT ( 'NONE', #16882 ) ;
#19216=VECTOR ( 'NONE', #5448, 1000.000000000000000 ) ;
#19218=LINE ( 'NONE', #16934, #5744 ) ;
#19220=ORIENTED_EDGE ( 'NONE', *, *, #21520, .F. ) ;
#19222=EDGE_LOOP ( 'NONE', ( #27956, #10854, #18532, #9300 ) ) ;
#19228=ORIENTED_EDGE ( 'NONE', *, *, #10828, .F. ) ;
#19233=EDGE_CURVE ( 'NONE', #10558, #29062, #23931, .T. ) ;
#19234=ADVANCED_FACE ( 'NONE', ( #16740 ), #19620, .T. ) ;
#19236=ADVANCED_FACE ( 'NONE', ( #3174 ), #3323, .T. ) ;
#19238=EDGE_CURVE ( 'NONE', #11857, #17842, #711, .T. ) ;
#19240=FACE_BOUND ( 'NONE', #12944, .T. ) ;
#19241=VECTOR ( 'NONE', #2991, 1000.000000000000000 ) ;
#19242=DIRECTION ( 'NONE',  ( -0.5877852522924731371, -1.586114251531760235E-16, 0.8090169943749474513 ) ) ;
#19243=CARTESIAN_POINT ( 'NONE',  ( 136.1922820468854241, -4.999999999999981348, -22.25671179336495697 ) ) ;
#19244=CARTESIAN_POINT ( 'NONE',  ( 144.5152310637605524, -4.999999999999978684, -13.05155085951651195 ) ) ;
#19245=DIRECTION ( 'NONE',  ( -0.9510565162951536422, -2.566386769018988816E-16, -0.3090169943749472292 ) ) ;
#19249=DIRECTION ( 'NONE',  ( 0.9510565162951536422, 0.000000000000000000, -0.3090169943749475623 ) ) ;
#19250=ORIENTED_EDGE ( 'NONE', *, *, #14573, .T. ) ;
#19253=DIRECTION ( 'NONE',  ( -2.698458740408365879E-16, 1.000000000000000000, 0.000000000000000000 ) ) ;
#19255=ORIENTED_EDGE ( 'NONE', *, *, #8578, .T. ) ;
#19256=CARTESIAN_POINT ( 'NONE',  ( 19.10627256897540605, -5.000000000000012434, -58.80306054231878221 ) ) ;
#19257=ORIENTED_EDGE ( 'NONE', *, *, #950, .F. ) ;
#19258=CARTESIAN_POINT ( 'NONE',  ( 167.0152310637605524, -9.999999999999996447, -32.93883019725009120 ) ) ;
#19260=EDGE_LOOP ( 'NONE', ( #10287, #22014, #3361, #3372 ) ) ;
#19263=VERTEX_POINT ( 'NONE', #3462 ) ;
#19264=AXIS2_PLACEMENT_3D ( 'NONE', #16964, #7215, #5822 ) ;
#19265=FACE_OUTER_BOUND ( 'NONE', #15767, .T. ) ;
#19270=EDGE_CURVE ( 'NONE', #21626, #6687, #5138, .T. ) ;
#19272=EDGE_CURVE ( 'NONE', #23960, #16007, #3023, .T. ) ;
#19274=EDGE_CURVE ( 'NONE', #756, #26426, #15035, .T. ) ;
#19275=CARTESIAN_POINT ( 'NONE',  ( 173.6922820468853672, -9.999999999999994671, -35.24709285013155835 ) ) ;
#19276=EDGE_CURVE ( 'NONE', #9240, #30179, #12298, .T. ) ;
#19278=ORIENTED_EDGE ( 'NONE', *, *, #23377, .F. ) ;
#19279=LINE ( 'NONE', #18829, #10723 ) ;
#19280=VECTOR ( 'NONE', #5002, 1000.000000000000000 ) ;
#19282=DIRECTION ( 'NONE',  ( -2.698458740408365879E-16, 1.000000000000000000, 0.000000000000000000 ) ) ;
#19283=FACE_OUTER_BOUND ( 'NONE', #12862, .T. ) ;
#19285=CARTESIAN_POINT ( 'NONE',  ( 143.6922820468853956, -1.999999999999978462, 2.247092850131521491 ) ) ;
#19291=EDGE_LOOP ( 'NONE', ( #9414, #20129, #6240, #13102 ) ) ;
#19292=CARTESIAN_POINT ( 'NONE',  ( 133.6922820468853956, -1.999999999999980904, -6.413161187712875133 ) ) ;
#19293=DIRECTION ( 'NONE',  ( -2.698458740408365879E-16, 1.000000000000000000, 0.000000000000000000 ) ) ;
#19295=CARTESIAN_POINT ( 'NONE',  ( 125.7287565553229456, -84.33034373659255323, -33.50000000000000000 ) ) ;
#19299=CARTESIAN_POINT ( 'NONE',  ( 151.1922820468854241, -1.999999999999976241, -28.06379628232387446 ) ) ;
#19301=CARTESIAN_POINT ( 'NONE',  ( 130.7287565553229456, -4.999999999999983125, 3.500000000000003109 ) ) ;
#19302=DIRECTION ( 'NONE',  ( -0.9510565162951536422, 0.000000000000000000, -0.3090169943749472292 ) ) ;
#19309=VECTOR ( 'NONE', #8449, 1000.000000000000000 ) ;
#19310=EDGE_CURVE ( 'NONE', #3398, #18151, #13211, .T. ) ;
#19314=EDGE_CURVE ( 'NONE', #25811, #28921, #8329, .T. ) ;
#19315=EDGE_CURVE ( 'NONE', #10352, #28379, #12901, .T. ) ;
#19316=CARTESIAN_POINT ( 'NONE',  ( 131.1922820468854241, -4.999999999999982236, -13.59645775552055547 ) ) ;
#19317=CARTESIAN_POINT ( 'NONE',  ( 158.6922820468853956, -9.999999999999998224, -26.58683881228715862 ) ) ;
#19318=LINE ( 'NONE', #26674, #10610 ) ;
#19320=VECTOR ( 'NONE', #7084, 1000.000000000000000 ) ;
#19321=CARTESIAN_POINT ( 'NONE',  ( 144.7287565553230309, -4.999999999999978684, -25.16025403784439973 ) ) ;
#19323=VECTOR ( 'NONE', #9803, 1000.000000000000000 ) ;
#19325=VECTOR ( 'NONE', #28164, 1000.000000000000000 ) ;
#19326=DIRECTION ( 'NONE',  ( 0.9510565162951536422, 2.566386769018988816E-16, 0.3090169943749472292 ) ) ;
#19327=DIRECTION ( 'NONE',  ( -2.698458740408365879E-16, 1.000000000000000000, 0.000000000000000000 ) ) ;
#19329=DIRECTION ( 'NONE',  ( 0.3090169943749475623, 8.338696094058001131E-17, 0.9510565162951536422 ) ) ;
#19330=CARTESIAN_POINT ( 'NONE',  ( 14.49336047848676223, -5.000000000000013323, -44.60597694298518689 ) ) ;
#19331=ORIENTED_EDGE ( 'NONE', *, *, #11949, .T. ) ;
#19332=DIRECTION ( 'NONE',  ( 1.110223024625156540E-16, 2.995891024602366092E-32, 1.000000000000000000 ) ) ;
#19333=LINE ( 'NONE', #28857, #15640 ) ;
#19334=CARTESIAN_POINT ( 'NONE',  ( 20.61759372714454841, -5.000000000000012434, -63.45442879020060900 ) ) ;
#19340=EDGE_CURVE ( 'NONE', #3218, #288, #18084, .T. ) ;
#19342=VECTOR ( 'NONE', #25849, 1000.000000000000000 ) ;
#19343=FACE_OUTER_BOUND ( 'NONE', #29423, .T. ) ;
#19344=DIRECTION ( 'NONE',  ( -0.9510565162951536422, -2.566386769018988323E-16, 0.3090169943749475623 ) ) ;
#19345=EDGE_CURVE ( 'NONE', #1366, #2635, #13355, .T. ) ;
#19347=ADVANCED_FACE ( 'NONE', ( #6198 ), #15788, .T. ) ;
#19348=CARTESIAN_POINT ( 'NONE',  ( 142.2287565553230309, -1.999999999999978018, -12.16987298107780369 ) ) ;
#19349=ORIENTED_EDGE ( 'NONE', *, *, #22109, .F. ) ;
#19350=DIRECTION ( 'NONE',  ( -0.9510565162951536422, -2.566386769018988816E-16, -0.3090169943749472292 ) ) ;
#19351=DIRECTION ( 'NONE',  ( 1.000000000000000000, 2.698458740408365879E-16, -1.110223024625156540E-16 ) ) ;
#19353=CARTESIAN_POINT ( 'NONE',  ( 142.0152310637605524, -4.999999999999978684, 1.702185954127501066 ) ) ;
#19357=ORIENTED_EDGE ( 'NONE', *, *, #18264, .T. ) ;
#19359=CARTESIAN_POINT ( 'NONE',  ( 169.5152310637604955, -9.999999999999996447, -19.94844914048349693 ) ) ;
#19360=VECTOR ( 'NONE', #8328, 1000.000000000000000 ) ;
#19363=DIRECTION ( 'NONE',  ( -2.698458740408365879E-16, 1.000000000000000000, 0.000000000000000000 ) ) ;
#19364=ORIENTED_EDGE ( 'NONE', *, *, #5212, .F. ) ;
#19366=EDGE_LOOP ( 'NONE', ( #25289, #22310, #27622, #2616 ) ) ;
#19367=VECTOR ( 'NONE', #13926, 1000.000000000000000 ) ;
#19371=DIRECTION ( 'NONE',  ( -0.5877852522924731371, -1.586114251531760728E-16, -0.8090169943749474513 ) ) ;
#19372=ORIENTED_EDGE ( 'NONE', *, *, #10935, .T. ) ;
#19373=DIRECTION ( 'NONE',  ( -1.000000000000000000, -2.891205793294689173E-16, 0.000000000000000000 ) ) ;
#19374=EDGE_LOOP ( 'NONE', ( #14690, #9116, #14084, #7590 ) ) ;
#19380=ORIENTED_EDGE ( 'NONE', *, *, #230, .F. ) ;
#19381=CARTESIAN_POINT ( 'NONE',  ( 7.261140001955372014, -5.000000000000015987, 22.34749104514272844 ) ) ;
#19382=VERTEX_POINT ( 'NONE', #3609 ) ;
#19383=EDGE_CURVE ( 'NONE', #7231, #21422, #10912, .T. ) ;
#19388=CARTESIAN_POINT ( 'NONE',  ( 136.1922820468854241, -10.00000000000000533, -19.40354224447947473 ) ) ;
#19390=VECTOR ( 'NONE', #18487, 1000.000000000000000 ) ;
#19392=CARTESIAN_POINT ( 'NONE',  ( 139.5152310637605524, -1.999999999999979128, -4.391296821672111328 ) ) ;
#19393=DIRECTION ( 'NONE',  ( -1.110223024625156540E-16, 0.000000000000000000, -1.000000000000000000 ) ) ;
#19396=CARTESIAN_POINT ( 'NONE',  ( 105.4221331823114127, -4.999999999999988454, -76.59366314999438430 ) ) ;
#19397=EDGE_CURVE ( 'NONE', #19635, #20619, #22377, .T. ) ;
#19398=ORIENTED_EDGE ( 'NONE', *, *, #16238, .F. ) ;
#19399=LINE ( 'NONE', #17264, #5218 ) ;
#19400=ORIENTED_EDGE ( 'NONE', *, *, #18688, .F. ) ;
#19402=EDGE_CURVE ( 'NONE', #12094, #20051, #29132, .T. ) ;
#19403=ORIENTED_EDGE ( 'NONE', *, *, #9301, .F. ) ;
#19405=LINE ( 'NONE', #12087, #6380 ) ;
#19406=CARTESIAN_POINT ( 'NONE',  ( 148.6922820468853672, -1.999999999999977129, 2.247092850131519715 ) ) ;
#19407=DIRECTION ( 'NONE',  ( 0.5877852522924731371, 0.000000000000000000, 0.8090169943749474513 ) ) ;
#19408=ORIENTED_EDGE ( 'NONE', *, *, #12759, .F. ) ;
#19409=LINE ( 'NONE', #26766, #27152 ) ;
#19410=ORIENTED_EDGE ( 'NONE', *, *, #10485, .F. ) ;
#19412=VERTEX_POINT ( 'NONE', #26987 ) ;
#19413=AXIS2_PLACEMENT_3D ( 'NONE', #15400, #24733, #20135 ) ;
#19416=VERTEX_POINT ( 'NONE', #6352 ) ;
#19417=DIRECTION ( 'NONE',  ( 0.5877852522924731371, 1.586114251531760728E-16, 0.8090169943749474513 ) ) ;
#19425=DIRECTION ( 'NONE',  ( -2.698458740408365879E-16, 1.000000000000000000, 0.000000000000000000 ) ) ;
#19428=CARTESIAN_POINT ( 'NONE',  ( 94.75885269270503386, -4.999999999999992006, -68.84633638624551111 ) ) ;
#19429=CARTESIAN_POINT ( 'NONE',  ( 147.0152310637606092, -1.999999999999976241, -32.93883019725009120 ) ) ;
#19431=DIRECTION ( 'NONE',  ( -2.698458740408365879E-16, 1.000000000000000000, 0.000000000000000000 ) ) ;
#19437=EDGE_CURVE ( 'NONE', #8011, #4895, #4207, .T. ) ;
#19439=ORIENTED_EDGE ( 'NONE', *, *, #6301, .F. ) ;
#19440=VECTOR ( 'NONE', #26937, 1000.000000000000000 ) ;
#19442=CARTESIAN_POINT ( 'NONE',  ( 164.5152310637605240, -1.999999999999971356, -28.60870317832789667 ) ) ;
#19444=CARTESIAN_POINT ( 'NONE',  ( 148.6922820468854241, -1.999999999999976685, -17.92658477444275889 ) ) ;
#19445=ADVANCED_FACE ( 'NONE', ( #13503 ), #10459, .T. ) ;
#19446=CARTESIAN_POINT ( 'NONE',  ( 148.6922820468854525, -1.999999999999976241, -26.58683881228715862 ) ) ;
#19447=CARTESIAN_POINT ( 'NONE',  ( 143.6922820468854525, -1.999999999999977573, -23.73366926340167282 ) ) ;
#19448=EDGE_CURVE ( 'NONE', #30101, #2137, #17631, .T. ) ;
#19450=ORIENTED_EDGE ( 'NONE', *, *, #16372, .F. ) ;
#19451=DIRECTION ( 'NONE',  ( -0.8090169943749474513, -2.183098979609982436E-16, -0.5877852522924731371 ) ) ;
#19453=DIRECTION ( 'NONE',  ( -0.8090169943749474513, -2.183098979609982436E-16, 0.5877852522924731371 ) ) ;
#19457=EDGE_LOOP ( 'NONE', ( #2801, #25927, #5627, #9504 ) ) ;
#19459=ORIENTED_EDGE ( 'NONE', *, *, #6300, .F. ) ;
#19467=ORIENTED_EDGE ( 'NONE', *, *, #27731, .F. ) ;
#19468=DIRECTION ( 'NONE',  ( 0.9510565162951536422, 0.000000000000000000, -0.3090169943749475623 ) ) ;
#19471=CARTESIAN_POINT ( 'NONE',  ( 131.1922820468854241, -1.999999999999982236, -4.936203717676158398 ) ) ;
#19474=VECTOR ( 'NONE', #25315, 1000.000000000000000 ) ;
#19476=EDGE_CURVE ( 'NONE', #13972, #21176, #17482, .T. ) ;
#19477=LINE ( 'NONE', #717, #14662 ) ;
#19478=CARTESIAN_POINT ( 'NONE',  ( 139.5152310637606092, -10.00000000000000533, -28.60870317832789311 ) ) ;
#19479=EDGE_CURVE ( 'NONE', #18472, #12418, #8475, .T. ) ;
#19480=EDGE_CURVE ( 'NONE', #14, #25907, #10616, .T. ) ;
#19481=VECTOR ( 'NONE', #17779, 1000.000000000000000 ) ;
#19483=CARTESIAN_POINT ( 'NONE',  ( 163.6922820468852819, -9.999999999999998224, -0.6060766987539614181 ) ) ;
#19484=EDGE_CURVE ( 'NONE', #28345, #22694, #15184, .T. ) ;
#19486=ORIENTED_EDGE ( 'NONE', *, *, #27860, .T. ) ;
#19488=CARTESIAN_POINT ( 'NONE',  ( 137.0152310637605808, -1.999999999999979572, -8.721423840594312082 ) ) ;
#19489=DIRECTION ( 'NONE',  ( -0.9510565162951536422, -2.566386769018988323E-16, 0.3090169943749475623 ) ) ;
#19492=VERTEX_POINT ( 'NONE', #20664 ) ;
#19496=CARTESIAN_POINT ( 'NONE',  ( 100.3929811530477423, -4.999999999999990230, 72.93977032092985269 ) ) ;
#19497=DIRECTION ( 'NONE',  ( -2.698458740408365879E-16, 1.000000000000000000, 0.000000000000000000 ) ) ;
#19499=CARTESIAN_POINT ( 'NONE',  ( 177.2287565553229172, -9.999999999999994671, -29.49038105676660493 ) ) ;
#19501=DIRECTION ( 'NONE',  ( 0.3090169943749472292, 8.338696094057992503E-17, -0.9510565162951536422 ) ) ;
#19503=CARTESIAN_POINT ( 'NONE',  ( 143.6922820468854525, -10.00000000000000355, -26.58683881228715506 ) ) ;
#19504=FACE_OUTER_BOUND ( 'NONE', #10801, .T. ) ;
#19507=VECTOR ( 'NONE', #886, 1000.000000000000000 ) ;
#19512=ADVANCED_FACE ( 'NONE', ( #6647 ), #20973, .T. ) ;
#19514=ADVANCED_FACE ( 'NONE', ( #11659 ), #6952, .T. ) ;
#19516=FACE_BOUND ( 'NONE', #20146, .T. ) ;
#19518=ORIENTED_EDGE ( 'NONE', *, *, #7017, .F. ) ;
#19520=VERTEX_POINT ( 'NONE', #18693 ) ;
#19521=CARTESIAN_POINT ( 'NONE',  ( 147.0152310637605240, -4.999999999999977796, -8.721423840594312082 ) ) ;
#19523=FACE_OUTER_BOUND ( 'NONE', #15383, .T. ) ;
#19524=ORIENTED_EDGE ( 'NONE', *, *, #25290, .F. ) ;
#19525=FACE_OUTER_BOUND ( 'NONE', #19975, .T. ) ;
#19526=EDGE_LOOP ( 'NONE', ( #23517, #11490, #18848, #21935 ) ) ;
#19531=EDGE_LOOP ( 'NONE', ( #16018, #3059, #8356, #15389 ) ) ;
#19535=AXIS2_PLACEMENT_3D ( 'NONE', #15499, #6656, #10779 ) ;
#19537=VERTEX_POINT ( 'NONE', #23270 ) ;
#19539=AXIS2_PLACEMENT_3D ( 'NONE', #22468, #10997, #12994 ) ;
#19543=DIRECTION ( 'NONE',  ( 2.698458740408365879E-16, -1.000000000000000000, 0.000000000000000000 ) ) ;
#19544=CARTESIAN_POINT ( 'NONE',  ( 129.5152310637605524, -1.999999999999982236, -30.37205893520530964 ) ) ;
#19545=DIRECTION ( 'NONE',  ( -2.698458740408365879E-16, 1.000000000000000000, 0.000000000000000000 ) ) ;
#19546=CARTESIAN_POINT ( 'NONE',  ( 162.0152310637605240, -9.999999999999998224, -24.27857615940569502 ) ) ;
#19549=ADVANCED_FACE ( 'NONE', ( #7094 ), #28039, .T. ) ;
#19551=VECTOR ( 'NONE', #25562, 1000.000000000000000 ) ;
#19552=FACE_OUTER_BOUND ( 'NONE', #29129, .T. ) ;
#19553=ORIENTED_EDGE ( 'NONE', *, *, #29567, .T. ) ;
#19554=VECTOR ( 'NONE', #21451, 1000.000000000000000 ) ;
#19557=PLANE ( 'NONE',  #1507 ) ;
#19558=LINE ( 'NONE', #28926, #18868 ) ;
#19559=CARTESIAN_POINT ( 'NONE',  ( 162.2287565553228887, -10.00000000000000000, -3.509618943233403510 ) ) ;
#19560=ORIENTED_EDGE ( 'NONE', *, *, #20735, .T. ) ;
#19562=VERTEX_POINT ( 'NONE', #13656 ) ;
#19566=VERTEX_POINT ( 'NONE', #2083 ) ;
#19568=LINE ( 'NONE', #29398, #10614 ) ;
#19570=DIRECTION ( 'NONE',  ( -0.8090169943749474513, -2.183098979609982436E-16, 0.5877852522924731371 ) ) ;
#19571=CARTESIAN_POINT ( 'NONE',  ( 152.0152310637604671, -1.999999999999976241, -17.38167787843870826 ) ) ;
#19572=VERTEX_POINT ( 'NONE', #11502 ) ;
#19577=ORIENTED_EDGE ( 'NONE', *, *, #3746, .F. ) ;
#19578=EDGE_CURVE ( 'NONE', #8151, #20829, #20815, .T. ) ;
#19579=LINE ( 'NONE', #25226, #12769 ) ;
#19580=DIRECTION ( 'NONE',  ( -0.5877852522924731371, -1.586114251531760235E-16, 0.8090169943749474513 ) ) ;
#19583=DIRECTION ( 'NONE',  ( -2.698458740408365879E-16, 1.000000000000000000, 0.000000000000000000 ) ) ;
#19587=ORIENTED_EDGE ( 'NONE', *, *, #11041, .T. ) ;
#19588=LINE ( 'NONE', #10426, #6161 ) ;
#19592=VECTOR ( 'NONE', #28408, 1000.000000000000000 ) ;
#19593=LINE ( 'NONE', #21441, #29812 ) ;
#19594=FACE_OUTER_BOUND ( 'NONE', #19979, .T. ) ;
#19596=ORIENTED_EDGE ( 'NONE', *, *, #12444, .T. ) ;
#19597=CARTESIAN_POINT ( 'NONE',  ( 172.7287565553229456, -4.999999999999970690, -36.50000000000000711 ) ) ;
#19599=DIRECTION ( 'NONE',  ( -2.698458740408365879E-16, 1.000000000000000000, 0.000000000000000000 ) ) ;
#19600=PLANE ( 'NONE',  #3474 ) ;
#19602=CARTESIAN_POINT ( 'NONE',  ( 147.0152310637605240, -10.00000000000000355, 1.702185954127501066 ) ) ;
#19604=ORIENTED_EDGE ( 'NONE', *, *, #14261, .F. ) ;
#19605=CARTESIAN_POINT ( 'NONE',  ( 134.7287565553230024, -4.999999999999981348, -25.16025403784439973 ) ) ;
#19606=DIRECTION ( 'NONE',  ( 0.000000000000000000, 0.000000000000000000, 1.000000000000000000 ) ) ;
#19610=ORIENTED_EDGE ( 'NONE', *, *, #22492, .T. ) ;
#19611=EDGE_CURVE ( 'NONE', #15277, #1403, #9512, .T. ) ;
#19614=EDGE_CURVE ( 'NONE', #11987, #10350, #20521, .T. ) ;
#19615=VECTOR ( 'NONE', #28344, 999.9999999999998863 ) ;
#19616=EDGE_CURVE ( 'NONE', #25730, #1623, #25717, .T. ) ;
#19617=CARTESIAN_POINT ( 'NONE',  ( 133.6922820468854241, -10.00000000000000711, -17.92658477444275533 ) ) ;
#19618=ORIENTED_EDGE ( 'NONE', *, *, #6642, .T. ) ;
#19620=PLANE ( 'NONE',  #16785 ) ;
#19624=DIRECTION ( 'NONE',  ( -0.8090169943749474513, -2.183098979609982436E-16, 0.5877852522924731371 ) ) ;
#19625=DIRECTION ( 'NONE',  ( 0.9510565162951536422, 2.566386769018988816E-16, 0.3090169943749472292 ) ) ;
#19627=DIRECTION ( 'NONE',  ( 0.9510565162951536422, 0.000000000000000000, -0.3090169943749475623 ) ) ;
#19628=DIRECTION ( 'NONE',  ( 0.9510565162951536422, 2.566386769018988816E-16, 0.3090169943749472292 ) ) ;
#19630=LINE ( 'NONE', #17343, #11494 ) ;
#19631=DIRECTION ( 'NONE',  ( -2.698458740408365879E-16, 1.000000000000000000, 0.000000000000000000 ) ) ;
#19632=DIRECTION ( 'NONE',  ( -2.698458740408365879E-16, 1.000000000000000000, 0.000000000000000000 ) ) ;
#19633=AXIS2_PLACEMENT_3D ( 'NONE', #26396, #5475, #24097 ) ;
#19634=ORIENTED_EDGE ( 'NONE', *, *, #12760, .F. ) ;
#19635=VERTEX_POINT ( 'NONE', #11360 ) ;
#19636=VERTEX_POINT ( 'NONE', #9211 ) ;
#19638=VERTEX_POINT ( 'NONE', #25554 ) ;
#19641=LINE ( 'NONE', #8045, #12095 ) ;
#19643=CARTESIAN_POINT ( 'NONE',  ( 91.90913672266484014, -4.999999999999992006, -66.77589654127525876 ) ) ;
#19644=ADVANCED_FACE ( 'NONE', ( #21125 ), #27740, .T. ) ;
#19645=ORIENTED_EDGE ( 'NONE', *, *, #27215, .T. ) ;
#19646=EDGE_CURVE ( 'NONE', #16894, #11008, #27892, .T. ) ;
#19647=CARTESIAN_POINT ( 'NONE',  ( 162.0152310637605240, -1.999999999999972244, -24.27857615940569502 ) ) ;
#19648=ORIENTED_EDGE ( 'NONE', *, *, #27690, .F. ) ;
#19649=DIRECTION ( 'NONE',  ( -2.698458740408365879E-16, 1.000000000000000000, 0.000000000000000000 ) ) ;
#19650=DIRECTION ( 'NONE',  ( 6.938893903907227392E-16, -0.000000000000000000, 1.000000000000000000 ) ) ;
#19651=ORIENTED_EDGE ( 'NONE', *, *, #9887, .F. ) ;
#19652=DIRECTION ( 'NONE',  ( -0.9510565162951536422, -2.566386769018988816E-16, -0.3090169943749472292 ) ) ;
#19653=DIRECTION ( 'NONE',  ( -2.698458740408365879E-16, 1.000000000000000000, 0.000000000000000000 ) ) ;
#19657=ORIENTED_EDGE ( 'NONE', *, *, #20203, .F. ) ;
#19661=FACE_BOUND ( 'NONE', #12205, .T. ) ;
#19666=CARTESIAN_POINT ( 'NONE',  ( 142.0152310637605808, -1.999999999999978018, -26.04193191628310800 ) ) ;
#19667=ORIENTED_EDGE ( 'NONE', *, *, #483, .T. ) ;
#19668=VERTEX_POINT ( 'NONE', #26178 ) ;
#19669=DIRECTION ( 'NONE',  ( 0.5877852522924731371, 0.000000000000000000, 0.8090169943749474513 ) ) ;
#19670=EDGE_LOOP ( 'NONE', ( #12039, #30221, #16106, #29028 ) ) ;
#19675=ORIENTED_EDGE ( 'NONE', *, *, #18075, .F. ) ;
#19676=DIRECTION ( 'NONE',  ( -0.9510565162951536422, -2.566386769018988323E-16, 0.3090169943749475623 ) ) ;
#19678=EDGE_LOOP ( 'NONE', ( #23472, #7926, #4242, #30066 ) ) ;
#19683=ADVANCED_FACE ( 'NONE', ( #12266 ), #14842, .F. ) ;
#19684=ADVANCED_FACE ( 'NONE', ( #2831 ), #9971, .T. ) ;
#19686=EDGE_CURVE ( 'NONE', #11956, #6838, #21728, .T. ) ;
#19687=FACE_OUTER_BOUND ( 'NONE', #27460, .T. ) ;
#19689=FACE_BOUND ( 'NONE', #26765, .T. ) ;
#19690=DIRECTION ( 'NONE',  ( 0.000000000000000000, 0.000000000000000000, -1.000000000000000000 ) ) ;
#19691=CARTESIAN_POINT ( 'NONE',  ( 139.5152310637606092, -10.00000000000000533, -11.28819510263909542 ) ) ;
#19692=DIRECTION ( 'NONE',  ( 0.5877852522924731371, 1.586114251531760728E-16, -0.8090169943749474513 ) ) ;
#19693=ORIENTED_EDGE ( 'NONE', *, *, #7017, .T. ) ;
#19694=LINE ( 'NONE', #17405, #6598 ) ;
#19697=FACE_OUTER_BOUND ( 'NONE', #6284, .T. ) ;
#19700=EDGE_LOOP ( 'NONE', ( #24575, #26955, #24281, #27052 ) ) ;
#19702=ORIENTED_EDGE ( 'NONE', *, *, #16918, .F. ) ;
#19705=CARTESIAN_POINT ( 'NONE',  ( 162.0152310637604671, -1.999999999999972689, -17.38167787843871182 ) ) ;
#19706=PLANE ( 'NONE',  #9555 ) ;
#19711=VERTEX_POINT ( 'NONE', #19285 ) ;
#19712=CARTESIAN_POINT ( 'NONE',  ( 78.64359365793785628, -4.999999999999996447, 57.13791534766453140 ) ) ;
#19714=CARTESIAN_POINT ( 'NONE',  ( 173.6922820468852819, -9.999999999999996447, -6.413161187712876909 ) ) ;
#19715=DIRECTION ( 'NONE',  ( 0.9510565162951536422, 0.000000000000000000, -0.3090169943749475623 ) ) ;
#19719=VECTOR ( 'NONE', #1896, 1000.000000000000000 ) ;
#19720=ORIENTED_EDGE ( 'NONE', *, *, #9092, .T. ) ;
#19721=EDGE_CURVE ( 'NONE', #19118, #27148, #23734, .T. ) ;
#19722=EDGE_CURVE ( 'NONE', #24484, #9002, #24182, .T. ) ;
#19723=ORIENTED_EDGE ( 'NONE', *, *, #24318, .T. ) ;
#19725=DIRECTION ( 'NONE',  ( -0.5877852522924731371, -1.586114251531760235E-16, 0.8090169943749474513 ) ) ;
#19726=VECTOR ( 'NONE', #9560, 1000.000000000000000 ) ;
#19728=PLANE ( 'NONE',  #24817 ) ;
#19734=EDGE_LOOP ( 'NONE', ( #27208, #5651, #24984, #12143 ) ) ;
#19737=LINE ( 'NONE', #10132, #7748 ) ;
#19738=CARTESIAN_POINT ( 'NONE',  ( 172.0152310637604955, -1.999999999999969358, -34.70218595412750773 ) ) ;
#19742=ORIENTED_EDGE ( 'NONE', *, *, #25415, .F. ) ;
#19743=LINE ( 'NONE', #19597, #29600 ) ;
#19745=EDGE_CURVE ( 'NONE', #17144, #2569, #991, .T. ) ;
#19747=CARTESIAN_POINT ( 'NONE',  ( 156.1922820468853388, -1.999999999999974909, -2.083034168790677043 ) ) ;
#19749=CARTESIAN_POINT ( 'NONE',  ( 172.2287565553229456, -1.999999999999969358, -29.49038105676660493 ) ) ;
#19751=EDGE_LOOP ( 'NONE', ( #26687, #19758, #15380, #22583 ) ) ;
#19753=VECTOR ( 'NONE', #19770, 1000.000000000000000 ) ;
#19756=LINE ( 'NONE', #24511, #27361 ) ;
#19757=VECTOR ( 'NONE', #7448, 999.9999999999998863 ) ;
#19758=ORIENTED_EDGE ( 'NONE', *, *, #17654, .F. ) ;
#19762=CARTESIAN_POINT ( 'NONE',  ( 136.1922820468854241, -4.999999999999981348, -2.083034168790677043 ) ) ;
#19763=CARTESIAN_POINT ( 'NONE',  ( 154.5152310637605240, -1.999999999999974465, -21.71180489736091346 ) ) ;
#19764=DIRECTION ( 'NONE',  ( -0.8090169943749474513, -2.183098979609982436E-16, 0.5877852522924731371 ) ) ;
#19768=VECTOR ( 'NONE', #5308, 1000.000000000000000 ) ;
#19770=DIRECTION ( 'NONE',  ( -0.5877852522924731371, -1.586114251531760235E-16, 0.8090169943749474513 ) ) ;
#19772=CARTESIAN_POINT ( 'NONE',  ( 131.1922820468854241, -4.999999999999982236, -30.91696583120935671 ) ) ;
#19774=EDGE_CURVE ( 'NONE', #20748, #29240, #21584, .T. ) ;
#19776=EDGE_CURVE ( 'NONE', #29672, #30260, #7692, .T. ) ;
#19777=ORIENTED_EDGE ( 'NONE', *, *, #29006, .F. ) ;
#19778=AXIS2_PLACEMENT_3D ( 'NONE', #9074, #18245, #15659 ) ;
#19780=LINE ( 'NONE', #3625, #16119 ) ;
#19781=EDGE_CURVE ( 'NONE', #7028, #25406, #9825, .T. ) ;
#19784=ORIENTED_EDGE ( 'NONE', *, *, #21204, .T. ) ;
#19785=ORIENTED_EDGE ( 'NONE', *, *, #25835, .T. ) ;
#19786=ORIENTED_EDGE ( 'NONE', *, *, #3607, .T. ) ;
#19790=CARTESIAN_POINT ( 'NONE',  ( 153.6922820468853388, -10.00000000000000178, -15.07341522555727309 ) ) ;
#19791=CARTESIAN_POINT ( 'NONE',  ( 132.0152310637605808, -1.999999999999981348, -6.958068083716893781 ) ) ;
#19792=LINE ( 'NONE', #26393, #2113 ) ;
#19793=VECTOR ( 'NONE', #4373, 1000.000000000000000 ) ;
#19797=PLANE ( 'NONE',  #15739 ) ;
#19799=FACE_OUTER_BOUND ( 'NONE', #23675, .T. ) ;
#19801=VECTOR ( 'NONE', #6133, 1000.000000000000000 ) ;
#19803=LINE ( 'NONE', #14913, #16607 ) ;
#19805=LINE ( 'NONE', #24255, #6053 ) ;
#19808=ORIENTED_EDGE ( 'NONE', *, *, #10557, .F. ) ;
#19813=FACE_BOUND ( 'NONE', #6182, .T. ) ;
#19814=EDGE_CURVE ( 'NONE', #29971, #28006, #26634, .T. ) ;
#19815=ORIENTED_EDGE ( 'NONE', *, *, #7874, .F. ) ;
#19816=LINE ( 'NONE', #1836, #26629 ) ;
#19818=VECTOR ( 'NONE', #2663, 1000.000000000000000 ) ;
#19820=LINE ( 'NONE', #17236, #4756 ) ;
#19823=DIRECTION ( 'NONE',  ( -1.110223024625156540E-16, 0.000000000000000000, -1.000000000000000000 ) ) ;
#19830=AXIS2_PLACEMENT_3D ( 'NONE', #1043, #22084, #27149 ) ;
#19831=DIRECTION ( 'NONE',  ( 0.9510565162951536422, 2.566386769018988816E-16, 0.3090169943749472292 ) ) ;
#19833=CARTESIAN_POINT ( 'NONE',  ( 177.2287565553229172, -9.999999999999994671, -29.49038105676660493 ) ) ;
#19835=CARTESIAN_POINT ( 'NONE',  ( 112.8128711859804554, -4.999999999999986677, -81.96334862300538759 ) ) ;
#19836=FACE_BOUND ( 'NONE', #29955, .T. ) ;
#19837=VECTOR ( 'NONE', #11304, 1000.000000000000000 ) ;
#19838=ORIENTED_EDGE ( 'NONE', *, *, #10523, .F. ) ;
#19840=LINE ( 'NONE', #29205, #16962 ) ;
#19841=DIRECTION ( 'NONE',  ( 1.000000000000000000, 2.698458740408365879E-16, -1.110223024625156540E-16 ) ) ;
#19842=AXIS2_PLACEMENT_3D ( 'NONE', #4558, #23036, #13846 ) ;
#19843=CARTESIAN_POINT ( 'NONE',  ( 133.7287565553229172, -4.999999999999982236, -36.50000000000000711 ) ) ;
#19845=CARTESIAN_POINT ( 'NONE',  ( 147.2287565553230309, -10.00000000000000178, -29.49038105676660138 ) ) ;
#19846=ORIENTED_EDGE ( 'NONE', *, *, #23172, .T. ) ;
#19848=DIRECTION ( 'NONE',  ( -0.9510565162951536422, -2.566386769018988323E-16, 0.3090169943749475623 ) ) ;
#19849=ORIENTED_EDGE ( 'NONE', *, *, #10480, .T. ) ;
#19852=EDGE_CURVE ( 'NONE', #1397, #29646, #28805, .T. ) ;
#19854=DIRECTION ( 'NONE',  ( -0.8090169943749474513, -2.183098979609982436E-16, -0.5877852522924731371 ) ) ;
#19855=LINE ( 'NONE', #29385, #14951 ) ;
#19856=EDGE_CURVE ( 'NONE', #26851, #16252, #21274, .T. ) ;
#19860=EDGE_CURVE ( 'NONE', #10405, #25866, #17737, .T. ) ;
#19861=VERTEX_POINT ( 'NONE', #6007 ) ;
#19865=ORIENTED_EDGE ( 'NONE', *, *, #12830, .T. ) ;
#19869=ORIENTED_EDGE ( 'NONE', *, *, #11828, .F. ) ;
#19872=VECTOR ( 'NONE', #17137, 1000.000000000000000 ) ;
#19874=VERTEX_POINT ( 'NONE', #8436 ) ;
#19875=ORIENTED_EDGE ( 'NONE', *, *, #19070, .F. ) ;
#19877=AXIS2_PLACEMENT_3D ( 'NONE', #21234, #11619, #20930 ) ;
#19878=DIRECTION ( 'NONE',  ( 0.5877852522924731371, 1.586114251531760728E-16, 0.8090169943749474513 ) ) ;
#19879=LINE ( 'NONE', #10726, #17694 ) ;
#19880=EDGE_CURVE ( 'NONE', #14895, #7328, #29098, .T. ) ;
#19881=CARTESIAN_POINT ( 'NONE',  ( 142.0152310637606092, -1.999999999999978018, -24.27857615940569147 ) ) ;
#19882=DIRECTION ( 'NONE',  ( -0.9510565162951536422, -2.566386769018988816E-16, -0.3090169943749472292 ) ) ;
#19883=LINE ( 'NONE', #17442, #28047 ) ;
#19888=ORIENTED_EDGE ( 'NONE', *, *, #18481, .F. ) ;
#19890=LINE ( 'NONE', #24192, #1901 ) ;
#19893=EDGE_CURVE ( 'NONE', #22605, #20491, #29250, .T. ) ;
#19894=LINE ( 'NONE', #15763, #4412 ) ;
#19895=CARTESIAN_POINT ( 'NONE',  ( 159.5152310637605524, -4.999999999999975131, -28.60870317832789667 ) ) ;
#19896=EDGE_CURVE ( 'NONE', #6528, #11987, #5864, .T. ) ;
#19899=VECTOR ( 'NONE', #7755, 1000.000000000000000 ) ;
#19900=ORIENTED_EDGE ( 'NONE', *, *, #23165, .T. ) ;
#19904=VECTOR ( 'NONE', #2948, 1000.000000000000000 ) ;
#19905=CARTESIAN_POINT ( 'NONE',  ( 132.0152310637605524, -10.00000000000000711, -17.38167787843870826 ) ) ;
#19906=CARTESIAN_POINT ( 'NONE',  ( 148.6922820468854525, -10.00000000000000178, -35.24709285013155835 ) ) ;
#19907=EDGE_LOOP ( 'NONE', ( #17187, #5483, #18787, #26605, #17906 ) ) ;
#19909=DIRECTION ( 'NONE',  ( 0.9510565162951536422, 0.000000000000000000, -0.3090169943749475623 ) ) ;
#19911=EDGE_LOOP ( 'NONE', ( #9952, #10491, #6128, #12456 ) ) ;
#19917=VERTEX_POINT ( 'NONE', #18042 ) ;
#19918=DIRECTION ( 'NONE',  ( -2.698458740408365879E-16, 1.000000000000000000, 0.000000000000000000 ) ) ;
#19919=VECTOR ( 'NONE', #24486, 1000.000000000000000 ) ;
#19920=CARTESIAN_POINT ( 'NONE',  ( 154.7287565553230024, -4.999999999999976019, -25.16025403784439973 ) ) ;
#19923=VECTOR ( 'NONE', #8173, 1000.000000000000000 ) ;
#19924=DIRECTION ( 'NONE',  ( -0.9510565162951536422, -2.566386769018988816E-16, -0.3090169943749472292 ) ) ;
#19925=DIRECTION ( 'NONE',  ( -2.698458740408365879E-16, 1.000000000000000000, 0.000000000000000000 ) ) ;
#19927=CARTESIAN_POINT ( 'NONE',  ( 158.6922820468853388, -1.999999999999974465, -9.266330736598359152 ) ) ;
#19929=LINE ( 'NONE', #10775, #19481 ) ;
#19931=DIRECTION ( 'NONE',  ( 1.000000000000000000, 2.698458740408365879E-16, -1.110223024625156540E-16 ) ) ;
#19933=DIRECTION ( 'NONE',  ( -0.9510565162951536422, -2.566386769018988323E-16, 0.3090169943749475623 ) ) ;
#19934=LINE ( 'NONE', #1492, #22202 ) ;
#19936=CARTESIAN_POINT ( 'NONE',  ( 3.362531273473086113, -5.000000000000016875, 10.34880714360505038 ) ) ;
#19937=ORIENTED_EDGE ( 'NONE', *, *, #24280, .T. ) ;
#19940=ORIENTED_EDGE ( 'NONE', *, *, #22873, .F. ) ;
#19941=VECTOR ( 'NONE', #19692, 1000.000000000000000 ) ;
#19944=LINE ( 'NONE', #1049, #26379 ) ;
#19946=ORIENTED_EDGE ( 'NONE', *, *, #13248, .T. ) ;
#19949=ORIENTED_EDGE ( 'NONE', *, *, #15163, .F. ) ;
#19952=PLANE ( 'NONE',  #23337 ) ;
#19953=LINE ( 'NONE', #1355, #4802 ) ;
#19955=VERTEX_POINT ( 'NONE', #14995 ) ;
#19958=EDGE_CURVE ( 'NONE', #3010, #23457, #20182, .T. ) ;
#19959=VECTOR ( 'NONE', #8545, 1000.000000000000000 ) ;
#19963=DIRECTION ( 'NONE',  ( -0.9510565162951536422, 0.000000000000000000, -0.3090169943749472292 ) ) ;
#19965=AXIS2_PLACEMENT_3D ( 'NONE', #22252, #19351, #7760 ) ;
#19968=EDGE_LOOP ( 'NONE', ( #2532, #7146, #29354, #3480, #19082 ) ) ;
#19970=EDGE_LOOP ( 'NONE', ( #19587, #18070, #21985, #16581, #24964 ) ) ;
#19973=FACE_BOUND ( 'NONE', #10885, .T. ) ;
#19974=ORIENTED_EDGE ( 'NONE', *, *, #20073, .T. ) ;
#19975=EDGE_LOOP ( 'NONE', ( #8050, #22304, #11483, #29629 ) ) ;
#19979=EDGE_LOOP ( 'NONE', ( #28697, #3332, #11896, #16670 ) ) ;
#19980=CARTESIAN_POINT ( 'NONE',  ( 143.6922820468854525, -1.999999999999978018, -35.24709285013155835 ) ) ;
#19984=ORIENTED_EDGE ( 'NONE', *, *, #13188, .F. ) ;
#19985=VECTOR ( 'NONE', #11854, 1000.000000000000000 ) ;
#19989=LINE ( 'NONE', #5506, #10151 ) ;
#19990=EDGE_LOOP ( 'NONE', ( #9103, #10389, #11713, #23659 ) ) ;
#19991=AXIS2_PLACEMENT_3D ( 'NONE', #24072, #2869, #575 ) ;
#19996=EDGE_CURVE ( 'NONE', #357, #18105, #6160, .T. ) ;
#19997=FACE_BOUND ( 'NONE', #27639, .T. ) ;
#19998=EDGE_CURVE ( 'NONE', #5507, #10809, #19883, .T. ) ;
#19999=VECTOR ( 'NONE', #16366, 1000.000000000000000 ) ;
#20001=ADVANCED_FACE ( 'NONE', ( #3874 ), #17596, .T. ) ;
#20002=ORIENTED_EDGE ( 'NONE', *, *, #12550, .T. ) ;
#20003=FACE_OUTER_BOUND ( 'NONE', #28025, .T. ) ;
#20005=DIRECTION ( 'NONE',  ( -2.698458740408365879E-16, 1.000000000000000000, 0.000000000000000000 ) ) ;
#20006=EDGE_LOOP ( 'NONE', ( #21914, #180, #23684, #28563 ) ) ;
#20007=CARTESIAN_POINT ( 'NONE',  ( 137.0152310637605808, -1.999999999999979572, -34.70218595412750773 ) ) ;
#20011=VERTEX_POINT ( 'NONE', #26793 ) ;
#20014=FACE_OUTER_BOUND ( 'NONE', #9397, .T. ) ;
#20015=CARTESIAN_POINT ( 'NONE',  ( 157.2287565553229740, -4.999999999999975131, -12.16987298107780013 ) ) ;
#20016=CARTESIAN_POINT ( 'NONE',  ( 106.9380661249224715, -4.999999999999988454, 77.69505290240560669 ) ) ;
#20017=ORIENTED_EDGE ( 'NONE', *, *, #4156, .T. ) ;
#20019=VECTOR ( 'NONE', #27490, 1000.000000000000000 ) ;
#20023=ORIENTED_EDGE ( 'NONE', *, *, #22360, .T. ) ;
#20024=DIRECTION ( 'NONE',  ( 0.5877852522924731371, 1.586114251531760728E-16, -0.8090169943749474513 ) ) ;
#20026=CARTESIAN_POINT ( 'NONE',  ( 167.0152310637604671, -1.999999999999971356, -17.38167787843871182 ) ) ;
#20027=EDGE_CURVE ( 'NONE', #8429, #16190, #3575, .T. ) ;
#20031=ORIENTED_EDGE ( 'NONE', *, *, #7941, .F. ) ;
#20036=EDGE_CURVE ( 'NONE', #19188, #6532, #24330, .T. ) ;
#20037=EDGE_CURVE ( 'NONE', #17144, #28891, #15147, .T. ) ;
#20038=CARTESIAN_POINT ( 'NONE',  ( 144.5152310637606092, -10.00000000000000178, -28.60870317832789311 ) ) ;
#20040=CARTESIAN_POINT ( 'NONE',  ( 177.2287565553228603, -9.999999999999994671, -12.16987298107780369 ) ) ;
#20041=PLANE ( 'NONE',  #3852 ) ;
#20042=VECTOR ( 'NONE', #18102, 1000.000000000000000 ) ;
#20043=DIRECTION ( 'NONE',  ( -2.698458740408365879E-16, 1.000000000000000000, 0.000000000000000000 ) ) ;
#20048=VERTEX_POINT ( 'NONE', #1288 ) ;
#20051=VERTEX_POINT ( 'NONE', #30011 ) ;
#20053=CARTESIAN_POINT ( 'NONE',  ( 172.0152310637604671, -1.999999999999969580, -26.04193191628311155 ) ) ;
#20055=VERTEX_POINT ( 'NONE', #18657 ) ;
#20056=CARTESIAN_POINT ( 'NONE',  ( 146.1922820468853956, -1.999999999999978018, -4.936203717676158398 ) ) ;
#20059=CARTESIAN_POINT ( 'NONE',  ( 137.2287565553230309, -1.999999999999979572, -20.83012701892220164 ) ) ;
#20061=DIRECTION ( 'NONE',  ( 1.110223024625156540E-16, 2.995891024602366092E-32, 1.000000000000000000 ) ) ;
#20063=ORIENTED_EDGE ( 'NONE', *, *, #3790, .T. ) ;
#20065=ORIENTED_EDGE ( 'NONE', *, *, #20203, .T. ) ;
#20073=EDGE_CURVE ( 'NONE', #8429, #21438, #20776, .T. ) ;
#20074=EDGE_CURVE ( 'NONE', #12292, #28345, #25675, .T. ) ;
#20077=EDGE_CURVE ( 'NONE', #8074, #28209, #22788, .T. ) ;
#20078=CARTESIAN_POINT ( 'NONE',  ( 143.6922820468854525, -1.999999999999977573, -15.07341522555727664 ) ) ;
#20080=DIRECTION ( 'NONE',  ( -2.698458740408365879E-16, 1.000000000000000000, 0.000000000000000000 ) ) ;
#20081=VECTOR ( 'NONE', #22590, 999.9999999999998863 ) ;
#20086=CARTESIAN_POINT ( 'NONE',  ( 134.5152310637605808, -10.00000000000000533, -19.94844914048349338 ) ) ;
#20089=LINE ( 'NONE', #29465, #19753 ) ;
#20091=DIRECTION ( 'NONE',  ( -0.5877852522924731371, -1.586114251531760235E-16, 0.8090169943749474513 ) ) ;
#20094=ORIENTED_EDGE ( 'NONE', *, *, #8983, .F. ) ;
#20095=CARTESIAN_POINT ( 'NONE',  ( 172.7287565553229456, -9.999999999999980460, -33.50000000000000000 ) ) ;
#20096=DIRECTION ( 'NONE',  ( -1.110223024625156540E-16, 0.000000000000000000, -1.000000000000000000 ) ) ;
#20098=CARTESIAN_POINT ( 'NONE',  ( 146.1922820468854525, -10.00000000000000178, -19.40354224447947828 ) ) ;
#20104=LINE ( 'NONE', #27017, #939 ) ;
#20105=CARTESIAN_POINT ( 'NONE',  ( 22.60637239937631193, -5.000000000000011546, -69.57526016881355702 ) ) ;
#20106=AXIS2_PLACEMENT_3D ( 'NONE', #28869, #1202, #10486 ) ;
#20108=EDGE_LOOP ( 'NONE', ( #4044, #17831, #11785, #3376 ) ) ;
#20111=ADVANCED_FACE ( 'NONE', ( #9478 ), #9019, .T. ) ;
#20113=DIRECTION ( 'NONE',  ( 0.3090169943749472292, 8.338696094057992503E-17, -0.9510565162951536422 ) ) ;
#20114=DIRECTION ( 'NONE',  ( 0.3090169943749472292, 8.338696094057992503E-17, -0.9510565162951536422 ) ) ;
#20118=ORIENTED_EDGE ( 'NONE', *, *, #21201, .F. ) ;
#20119=LINE ( 'NONE', #29499, #20019 ) ;
#20121=FACE_BOUND ( 'NONE', #15630, .T. ) ;
#20122=VERTEX_POINT ( 'NONE', #11462 ) ;
#20123=ORIENTED_EDGE ( 'NONE', *, *, #28580, .F. ) ;
#20125=ORIENTED_EDGE ( 'NONE', *, *, #19345, .F. ) ;
#20127=LINE ( 'NONE', #4261, #16924 ) ;
#20129=ORIENTED_EDGE ( 'NONE', *, *, #23733, .T. ) ;
#20131=ADVANCED_FACE ( 'NONE', ( #7062 ), #23232, .T. ) ;
#20132=EDGE_CURVE ( 'NONE', #5003, #26592, #30167, .T. ) ;
#20135=DIRECTION ( 'NONE',  ( -0.5877852522924731371, 0.000000000000000000, 0.8090169943749474513 ) ) ;
#20136=VERTEX_POINT ( 'NONE', #21090 ) ;
#20137=CARTESIAN_POINT ( 'NONE',  ( 176.1922820468853104, -9.999999999999994671, -19.40354224447947828 ) ) ;
#20139=AXIS2_PLACEMENT_3D ( 'NONE', #7543, #24176, #2828 ) ;
#20140=LINE ( 'NONE', #15254, #13462 ) ;
#20143=DIRECTION ( 'NONE',  ( -0.8090169943749474513, -2.183098979609982436E-16, 0.5877852522924731371 ) ) ;
#20145=DIRECTION ( 'NONE',  ( -0.5877852522924731371, 0.000000000000000000, 0.8090169943749474513 ) ) ;
#20146=EDGE_LOOP ( 'NONE', ( #8821, #2964, #16332, #27485, #21977 ) ) ;
#20148=DIRECTION ( 'NONE',  ( 0.9510565162951536422, 2.566386769018988816E-16, 0.3090169943749472292 ) ) ;
#20153=VECTOR ( 'NONE', #29493, 1000.000000000000000 ) ;
#20157=FACE_OUTER_BOUND ( 'NONE', #17411, .T. ) ;
#20158=VERTEX_POINT ( 'NONE', #4314 ) ;
#20160=EDGE_CURVE ( 'NONE', #6062, #28330, #2503, .T. ) ;
#20161=EDGE_CURVE ( 'NONE', #4310, #23706, #16354, .T. ) ;
#20165=ORIENTED_EDGE ( 'NONE', *, *, #19781, .T. ) ;
#20166=EDGE_CURVE ( 'NONE', #28008, #26448, #9174, .T. ) ;
#20167=VERTEX_POINT ( 'NONE', #11324 ) ;
#20169=EDGE_CURVE ( 'NONE', #21151, #29771, #9328, .T. ) ;
#20170=CARTESIAN_POINT ( 'NONE',  ( 174.7287565553228603, -9.999999999999996447, -7.839745962155603820 ) ) ;
#20174=EDGE_LOOP ( 'NONE', ( #21028, #22472, #22300, #22509 ) ) ;
#20175=ORIENTED_EDGE ( 'NONE', *, *, #11834, .F. ) ;
#20176=DIRECTION ( 'NONE',  ( -0.5877852522924731371, -1.586114251531760235E-16, 0.8090169943749474513 ) ) ;
#20177=LINE ( 'NONE', #10724, #11634 ) ;
#20179=CARTESIAN_POINT ( 'NONE',  ( 151.1922820468854525, -1.999999999999975353, -30.91696583120936026 ) ) ;
#20180=CARTESIAN_POINT ( 'NONE',  ( 174.5152310637604387, -1.999999999999969358, -21.71180489736091346 ) ) ;
#20182=LINE ( 'NONE', #10578, #4137 ) ;
#20187=ORIENTED_EDGE ( 'NONE', *, *, #8936, .F. ) ;
#20188=DIRECTION ( 'NONE',  ( 1.000000000000000000, 2.698458740408365879E-16, -1.110223024625156540E-16 ) ) ;
#20192=FACE_OUTER_BOUND ( 'NONE', #23942, .T. ) ;
#20196=ORIENTED_EDGE ( 'NONE', *, *, #10994, .T. ) ;
#20197=ORIENTED_EDGE ( 'NONE', *, *, #13854, .F. ) ;
#20198=LINE ( 'NONE', #8598, #9077 ) ;
#20200=EDGE_CURVE ( 'NONE', #25023, #20167, #28001, .T. ) ;
#20202=LINE ( 'NONE', #19906, #1546 ) ;
#20203=EDGE_CURVE ( 'NONE', #16222, #1559, #198, .T. ) ;
#20210=ORIENTED_EDGE ( 'NONE', *, *, #20702, .F. ) ;
#20217=CARTESIAN_POINT ( 'NONE',  ( 164.5152310637604671, -9.999999999999998224, -13.05155085951651195 ) ) ;
#20218=LINE ( 'NONE', #4352, #6343 ) ;
#20219=LINE ( 'NONE', #25267, #22825 ) ;
#20220=CARTESIAN_POINT ( 'NONE',  ( 134.5152310637605524, -4.999999999999981348, -1.493419066897600538E-14 ) ) ;
#20222=PLANE ( 'NONE',  #15031 ) ;
#20228=DIRECTION ( 'NONE',  ( 0.9510565162951536422, 2.566386769018988816E-16, 0.3090169943749472292 ) ) ;
#20231=CARTESIAN_POINT ( 'NONE',  ( 92.57941663348161399, -4.999999999999992006, 67.26288340215127448 ) ) ;
#20232=DIRECTION ( 'NONE',  ( -2.698458740408365879E-16, 1.000000000000000000, 0.000000000000000000 ) ) ;
#20234=ORIENTED_EDGE ( 'NONE', *, *, #13818, .F. ) ;
#20235=DIRECTION ( 'NONE',  ( 0.9510565162951536422, 2.566386769018988816E-16, 0.3090169943749472292 ) ) ;
#20236=CARTESIAN_POINT ( 'NONE',  ( 158.6922820468853956, -4.999999999999975131, -26.58683881228715862 ) ) ;
#20238=DIRECTION ( 'NONE',  ( 0.3090169943749475623, 8.338696094058001131E-17, 0.9510565162951536422 ) ) ;
#20240=EDGE_CURVE ( 'NONE', #6553, #22621, #16507, .T. ) ;
#20241=ORIENTED_EDGE ( 'NONE', *, *, #7367, .T. ) ;
#20242=EDGE_CURVE ( 'NONE', #3218, #14970, #21395, .T. ) ;
#20247=LINE ( 'NONE', #29483, #2407 ) ;
#20251=DIRECTION ( 'NONE',  ( -0.5877852522924731371, -1.586114251531760728E-16, -0.8090169943749474513 ) ) ;
#20252=VECTOR ( 'NONE', #5423, 1000.000000000000000 ) ;
#20253=CARTESIAN_POINT ( 'NONE',  ( 146.1922820468853956, -10.00000000000000355, -2.083034168790677043 ) ) ;
#20255=PLANE ( 'NONE',  #28340 ) ;
#20257=AXIS2_PLACEMENT_3D ( 'NONE', #11551, #15992, #30250 ) ;
#20258=DIRECTION ( 'NONE',  ( 0.5877852522924731371, 1.586114251531760728E-16, 0.8090169943749474513 ) ) ;
#20261=VECTOR ( 'NONE', #2397, 1000.000000000000000 ) ;
#20267=LINE ( 'NONE', #6699, #19474 ) ;
#20268=ORIENTED_EDGE ( 'NONE', *, *, #5398, .T. ) ;
#20269=CARTESIAN_POINT ( 'NONE',  ( 129.5152310637605524, -1.999999999999982236, -4.391296821672111328 ) ) ;
#20275=EDGE_LOOP ( 'NONE', ( #22112, #28027, #13527, #28510 ) ) ;
#20280=VECTOR ( 'NONE', #9382, 1000.000000000000000 ) ;
#20281=PLANE ( 'NONE',  #19413 ) ;
#20282=LINE ( 'NONE', #16157, #13733 ) ;
#20283=VECTOR ( 'NONE', #16370, 1000.000000000000000 ) ;
#20285=AXIS2_PLACEMENT_3D ( 'NONE', #3581, #20188, #29569 ) ;
#20286=PLANE ( 'NONE',  #12992 ) ;
#20287=LINE ( 'NONE', #11289, #17666 ) ;
#20289=EDGE_CURVE ( 'NONE', #21069, #13830, #14510, .T. ) ;
#20290=CARTESIAN_POINT ( 'NONE',  ( 175.7287565553229456, -4.999999999999970690, 3.500000000000003109 ) ) ;
#20292=DIRECTION ( 'NONE',  ( -0.9510565162951536422, 0.000000000000000000, -0.3090169943749472292 ) ) ;
#20293=ORIENTED_EDGE ( 'NONE', *, *, #28413, .T. ) ;
#20294=LINE ( 'NONE', #16174, #5623 ) ;
#20299=ORIENTED_EDGE ( 'NONE', *, *, #22242, .F. ) ;
#20300=VECTOR ( 'NONE', #2922, 1000.000000000000000 ) ;
#20306=DIRECTION ( 'NONE',  ( 0.5877852522924731371, 0.000000000000000000, 0.8090169943749474513 ) ) ;
#20311=ORIENTED_EDGE ( 'NONE', *, *, #9412, .T. ) ;
#20312=VERTEX_POINT ( 'NONE', #14353 ) ;
#20313=DIRECTION ( 'NONE',  ( -0.5877852522924731371, -1.586114251531760235E-16, 0.8090169943749474513 ) ) ;
#20314=DIRECTION ( 'NONE',  ( 0.9510565162951535312, 2.566386769018988816E-16, -0.3090169943749475623 ) ) ;
#20320=ORIENTED_EDGE ( 'NONE', *, *, #12270, .T. ) ;
#20322=CARTESIAN_POINT ( 'NONE',  ( 180.7287565553229456, -9.999999999999968026, 0.5000000000000029976 ) ) ;
#20323=AXIS2_PLACEMENT_3D ( 'NONE', #20718, #5007, #14296 ) ;
#20324=LINE ( 'NONE', #15288, #4827 ) ;
#20326=EDGE_CURVE ( 'NONE', #13853, #22891, #23690, .T. ) ;
#20328=CARTESIAN_POINT ( 'NONE',  ( 114.7516306444886141, -4.999999999999985789, 83.37193982118418489 ) ) ;
#20329=EDGE_CURVE ( 'NONE', #29150, #22621, #21841, .T. ) ;
#20333=DIRECTION ( 'NONE',  ( -1.110223024625156540E-16, 0.000000000000000000, -1.000000000000000000 ) ) ;
#20334=ORIENTED_EDGE ( 'NONE', *, *, #26225, .F. ) ;
#20336=FACE_OUTER_BOUND ( 'NONE', #13291, .T. ) ;
#20337=EDGE_LOOP ( 'NONE', ( #28117, #4463, #11307, #7055 ) ) ;
#20341=CARTESIAN_POINT ( 'NONE',  ( 146.1922820468854525, -1.999999999999977573, -28.06379628232387446 ) ) ;
#20342=DIRECTION ( 'NONE',  ( -1.110223024625156540E-16, 0.000000000000000000, -1.000000000000000000 ) ) ;
#20344=VERTEX_POINT ( 'NONE', #5523 ) ;
#20345=ORIENTED_EDGE ( 'NONE', *, *, #977, .T. ) ;
#20346=CARTESIAN_POINT ( 'NONE',  ( 154.7287565553230024, -10.00000000000000000, -25.16025403784440329 ) ) ;
#20348=VECTOR ( 'NONE', #8386, 1000.000000000000000 ) ;
#20351=VERTEX_POINT ( 'NONE', #12372 ) ;
#20353=LINE ( 'NONE', #4490, #29664 ) ;
#20355=VERTEX_POINT ( 'NONE', #14659 ) ;
#20361=VECTOR ( 'NONE', #18083, 1000.000000000000000 ) ;
#20362=DIRECTION ( 'NONE',  ( -2.698458740408365879E-16, 1.000000000000000000, 0.000000000000000000 ) ) ;
#20363=ORIENTED_EDGE ( 'NONE', *, *, #23336, .T. ) ;
#20364=VERTEX_POINT ( 'NONE', #23851 ) ;
#20366=CARTESIAN_POINT ( 'NONE',  ( 172.0152310637604955, -1.999999999999969580, -24.27857615940569502 ) ) ;
#20367=VECTOR ( 'NONE', #28406, 1000.000000000000000 ) ;
#20369=EDGE_CURVE ( 'NONE', #11745, #12555, #9637, .T. ) ;
#20370=DIRECTION ( 'NONE',  ( -0.5877852522924731371, 0.000000000000000000, 0.8090169943749474513 ) ) ;
#20375=CARTESIAN_POINT ( 'NONE',  ( 172.0152310637605240, -1.999999999999969358, -32.93883019725009120 ) ) ;
#20377=CARTESIAN_POINT ( 'NONE',  ( 153.6922820468854525, -10.00000000000000000, -32.39392330124607611 ) ) ;
#20378=DIRECTION ( 'NONE',  ( 0.9510565162951535312, 2.566386769018988816E-16, -0.3090169943749475623 ) ) ;
#20382=FACE_OUTER_BOUND ( 'NONE', #2327, .T. ) ;
#20384=VERTEX_POINT ( 'NONE', #7507 ) ;
#20385=LINE ( 'NONE', #27605, #29116 ) ;
#20387=VECTOR ( 'NONE', #5345, 1000.000000000000000 ) ;
#20388=CARTESIAN_POINT ( 'NONE',  ( 163.6922820468853672, -9.999999999999998224, -26.58683881228715862 ) ) ;
#20389=ORIENTED_EDGE ( 'NONE', *, *, #27219, .T. ) ;
#20392=VECTOR ( 'NONE', #21432, 1000.000000000000000 ) ;
#20395=DIRECTION ( 'NONE',  ( -0.5877852522924731371, -1.586114251531760235E-16, 0.8090169943749474513 ) ) ;
#20397=CARTESIAN_POINT ( 'NONE',  ( 91.84383324292713269, -4.999999999999992006, 66.72845078601908142 ) ) ;
#20399=VECTOR ( 'NONE', #14314, 1000.000000000000000 ) ;
#20400=ORIENTED_EDGE ( 'NONE', *, *, #2566, .T. ) ;
#20404=EDGE_CURVE ( 'NONE', #5129, #28015, #14803, .T. ) ;
#20405=DIRECTION ( 'NONE',  ( 1.000000000000000000, 2.698458740408365879E-16, -1.110223024625156540E-16 ) ) ;
#20406=LINE ( 'NONE', #22718, #20153 ) ;
#20407=EDGE_CURVE ( 'NONE', #9856, #30027, #24143, .T. ) ;
#20408=ADVANCED_FACE ( 'NONE', ( #3247 ), #24006, .T. ) ;
#20409=ADVANCED_FACE ( 'NONE', ( #7658 ), #18800, .T. ) ;
#20410=DIRECTION ( 'NONE',  ( 0.9510565162951535312, 2.566386769018988816E-16, -0.3090169943749475623 ) ) ;
#20412=AXIS2_PLACEMENT_3D ( 'NONE', #3720, #8580, #7987 ) ;
#20413=ORIENTED_EDGE ( 'NONE', *, *, #18138, .T. ) ;
#20415=ORIENTED_EDGE ( 'NONE', *, *, #28621, .F. ) ;
#20417=CARTESIAN_POINT ( 'NONE',  ( 167.0152310637604103, -9.999999999999998224, -0.06116980274991495881 ) ) ;
#20419=DIRECTION ( 'NONE',  ( 0.9510565162951536422, 0.000000000000000000, -0.3090169943749475623 ) ) ;
#20422=DIRECTION ( 'NONE',  ( 0.5877852522924731371, 0.000000000000000000, 0.8090169943749474513 ) ) ;
#20423=CARTESIAN_POINT ( 'NONE',  ( 130.7287565553229456, -4.999999999999982236, -13.44584919360585928 ) ) ;
#20425=ORIENTED_EDGE ( 'NONE', *, *, #20702, .T. ) ;
#20426=VERTEX_POINT ( 'NONE', #17259 ) ;
#20427=LINE ( 'NONE', #3662, #6686 ) ;
#20428=EDGE_LOOP ( 'NONE', ( #26943, #23211, #29194, #6738 ) ) ;
#20433=LINE ( 'NONE', #10972, #4308 ) ;
#20435=AXIS2_PLACEMENT_3D ( 'NONE', #25022, #12160, #28083 ) ;
#20437=EDGE_LOOP ( 'NONE', ( #14064, #21804, #15876, #689 ) ) ;
#20438=VECTOR ( 'NONE', #25302, 1000.000000000000000 ) ;
#20439=DIRECTION ( 'NONE',  ( 0.9510565162951536422, 0.000000000000000000, -0.3090169943749475623 ) ) ;
#20440=CARTESIAN_POINT ( 'NONE',  ( 175.7287565553229456, -4.999999999999970690, 0.5000000000000029976 ) ) ;
#20441=EDGE_CURVE ( 'NONE', #1081, #6635, #17559, .T. ) ;
#20443=EDGE_CURVE ( 'NONE', #10703, #22891, #1404, .T. ) ;
#20446=DIRECTION ( 'NONE',  ( 1.110223024625156540E-16, 2.995891024602366092E-32, 1.000000000000000000 ) ) ;
#20448=ORIENTED_EDGE ( 'NONE', *, *, #19860, .T. ) ;
#20453=VECTOR ( 'NONE', #2132, 1000.000000000000000 ) ;
#20458=DIRECTION ( 'NONE',  ( -2.698458740408365879E-16, 1.000000000000000000, 0.000000000000000000 ) ) ;
#20460=AXIS2_PLACEMENT_3D ( 'NONE', #10006, #26370, #19028 ) ;
#20462=AXIS2_PLACEMENT_3D ( 'NONE', #29905, #8913, #18229 ) ;
#20463=CARTESIAN_POINT ( 'NONE',  ( 104.2637232758598316, -4.999999999999989342, -75.75202908809458791 ) ) ;
#20464=ORIENTED_EDGE ( 'NONE', *, *, #16518, .F. ) ;
#20469=DIRECTION ( 'NONE',  ( 0.3090169943749472292, 8.338696094057992503E-17, -0.9510565162951536422 ) ) ;
#20471=CIRCLE ( 'NONE', #28329, 8.000000000000003553 ) ;
#20475=VECTOR ( 'NONE', #7997, 1000.000000000000000 ) ;
#20477=ORIENTED_EDGE ( 'NONE', *, *, #22797, .F. ) ;
#20478=PLANE ( 'NONE',  #29396 ) ;
#20479=AXIS2_PLACEMENT_3D ( 'NONE', #5688, #5385, #9943 ) ;
#20480=VECTOR ( 'NONE', #2077, 1000.000000000000000 ) ;
#20481=EDGE_CURVE ( 'NONE', #22503, #2774, #22298, .T. ) ;
#20482=DIRECTION ( 'NONE',  ( -2.698458740408365879E-16, 1.000000000000000000, 0.000000000000000000 ) ) ;
#20483=PLANE ( 'NONE',  #7273 ) ;
#20484=DIRECTION ( 'NONE',  ( -0.9510565162951536422, -2.566386769018988323E-16, 0.3090169943749475623 ) ) ;
#20487=CARTESIAN_POINT ( 'NONE',  ( 162.0152310637604387, -9.999999999999998224, 1.702185954127501066 ) ) ;
#20488=AXIS2_PLACEMENT_3D ( 'NONE', #23778, #21019, #124 ) ;
#20490=LINE ( 'NONE', #15905, #14436 ) ;
#20491=VERTEX_POINT ( 'NONE', #10235 ) ;
#20495=CARTESIAN_POINT ( 'NONE',  ( 149.5152310637605240, -1.999999999999976241, -13.05155085951651195 ) ) ;
#20496=LINE ( 'NONE', #25088, #11769 ) ;
#20498=ORIENTED_EDGE ( 'NONE', *, *, #16268, .T. ) ;
#20500=CARTESIAN_POINT ( 'NONE',  ( 142.0152310637605808, -10.00000000000000355, -17.38167787843871182 ) ) ;
#20502=VECTOR ( 'NONE', #16915, 1000.000000000000000 ) ;
#20505=ORIENTED_EDGE ( 'NONE', *, *, #3958, .T. ) ;
#20509=ORIENTED_EDGE ( 'NONE', *, *, #12547, .T. ) ;
#20511=EDGE_CURVE ( 'NONE', #2212, #2121, #22141, .T. ) ;
#20515=ORIENTED_EDGE ( 'NONE', *, *, #7872, .F. ) ;
#20516=DIRECTION ( 'NONE',  ( 2.908569913943825554E-16, -1.000000000000000000, 0.000000000000000000 ) ) ;
#20517=CARTESIAN_POINT ( 'NONE',  ( 171.1922820468852819, -4.999999999999970690, -2.083034168790677043 ) ) ;
#20519=DIRECTION ( 'NONE',  ( 0.5877852522924731371, 1.586114251531760728E-16, 0.8090169943749474513 ) ) ;
#20520=CARTESIAN_POINT ( 'NONE',  ( 173.6922820468852819, -1.999999999999970468, -6.413161187712876909 ) ) ;
#20521=LINE ( 'NONE', #18231, #5095 ) ;
#20522=DIRECTION ( 'NONE',  ( 0.3090169943749472292, 8.338696094057992503E-17, -0.9510565162951536422 ) ) ;
#20527=DIRECTION ( 'NONE',  ( 0.5877852522924731371, 1.586114251531760728E-16, -0.8090169943749474513 ) ) ;
#20529=CARTESIAN_POINT ( 'NONE',  ( 149.7287565553229456, -4.999999999999976907, 0.8205080756888000204 ) ) ;
#20530=DIRECTION ( 'NONE',  ( -0.8090169943749474513, -2.183098979609982436E-16, -0.5877852522924731371 ) ) ;
#20533=ORIENTED_EDGE ( 'NONE', *, *, #22360, .F. ) ;
#20534=CARTESIAN_POINT ( 'NONE',  ( 149.5152310637605240, -10.00000000000000178, -13.05155085951651195 ) ) ;
#20537=CARTESIAN_POINT ( 'NONE',  ( 172.0152310637604671, -1.999999999999970024, -15.61832212156129707 ) ) ;
#20538=LINE ( 'NONE', #29626, #9285 ) ;
#20539=VERTEX_POINT ( 'NONE', #20007 ) ;
#20541=ORIENTED_EDGE ( 'NONE', *, *, #23769, .F. ) ;
#20544=EDGE_CURVE ( 'NONE', #1647, #19572, #12679, .T. ) ;
#20547=ADVANCED_FACE ( 'NONE', ( #29529 ), #8399, .T. ) ;
#20549=ADVANCED_FACE ( 'NONE', ( #10534 ), #27064, .T. ) ;
#20550=LINE ( 'NONE', #13381, #8887 ) ;
#20553=DIRECTION ( 'NONE',  ( 0.9510565162951536422, 0.000000000000000000, -0.3090169943749475623 ) ) ;
#20555=ORIENTED_EDGE ( 'NONE', *, *, #18156, .F. ) ;
#20557=LINE ( 'NONE', #4100, #28310 ) ;
#20563=ORIENTED_EDGE ( 'NONE', *, *, #12031, .T. ) ;
#20568=PLANE ( 'NONE',  #6816 ) ;
#20569=LINE ( 'NONE', #25597, #10574 ) ;
#20571=LINE ( 'NONE', #27941, #24175 ) ;
#20577=ORIENTED_EDGE ( 'NONE', *, *, #24705, .F. ) ;
#20579=EDGE_CURVE ( 'NONE', #26897, #6453, #12828, .T. ) ;
#20583=ADVANCED_FACE ( 'NONE', ( #15417 ), #24751, .T. ) ;
#20585=DIRECTION ( 'NONE',  ( -2.698458740408365879E-16, 1.000000000000000000, 0.000000000000000000 ) ) ;
#20586=ADVANCED_FACE ( 'NONE', ( #13288 ), #22461, .T. ) ;
#20587=LINE ( 'NONE', #6716, #16685 ) ;
#20590=DIRECTION ( 'NONE',  ( 1.110223024625156540E-16, 2.995891024602366092E-32, 1.000000000000000000 ) ) ;
#20591=DIRECTION ( 'NONE',  ( -2.698458740408365879E-16, 1.000000000000000000, 0.000000000000000000 ) ) ;
#20595=PLANE ( 'NONE',  #5826 ) ;
#20596=EDGE_LOOP ( 'NONE', ( #10612, #12500, #29120, #28884 ) ) ;
#20597=ORIENTED_EDGE ( 'NONE', *, *, #21683, .F. ) ;
#20598=LINE ( 'NONE', #15721, #12927 ) ;
#20602=ORIENTED_EDGE ( 'NONE', *, *, #27691, .T. ) ;
#20604=PLANE ( 'NONE',  #12184 ) ;
#20606=CARTESIAN_POINT ( 'NONE',  ( 148.6922820468854525, -10.00000000000000178, -23.73366926340167637 ) ) ;
#20609=PLANE ( 'NONE',  #5682 ) ;
#20610=EDGE_LOOP ( 'NONE', ( #24383, #27874, #10060, #23628 ) ) ;
#20614=ORIENTED_EDGE ( 'NONE', *, *, #10654, .T. ) ;
#20616=ORIENTED_EDGE ( 'NONE', *, *, #8201, .F. ) ;
#20617=EDGE_CURVE ( 'NONE', #12856, #27966, #1107, .T. ) ;
#20619=VERTEX_POINT ( 'NONE', #5972 ) ;
#20620=VECTOR ( 'NONE', #21343, 1000.000000000000000 ) ;
#20622=EDGE_CURVE ( 'NONE', #18644, #20136, #19694, .T. ) ;
#20623=DIRECTION ( 'NONE',  ( -2.698458740408365879E-16, 1.000000000000000000, 0.000000000000000000 ) ) ;
#20627=ORIENTED_EDGE ( 'NONE', *, *, #19646, .F. ) ;
#20628=DIRECTION ( 'NONE',  ( 0.5877852522924731371, 0.000000000000000000, 0.8090169943749474513 ) ) ;
#20629=DIRECTION ( 'NONE',  ( -0.9510565162951536422, -2.566386769018988323E-16, 0.3090169943749475623 ) ) ;
#20630=LINE ( 'NONE', #24937, #17028 ) ;
#20636=ORIENTED_EDGE ( 'NONE', *, *, #10381, .F. ) ;
#20639=DIRECTION ( 'NONE',  ( 0.3090169943749475623, 8.338696094058001131E-17, 0.9510565162951536422 ) ) ;
#20643=CARTESIAN_POINT ( 'NONE',  ( 104.0883501548822636, -4.999999999999989342, 75.62461305743535434 ) ) ;
#20647=EDGE_CURVE ( 'NONE', #19412, #14559, #3683, .T. ) ;
#20649=CARTESIAN_POINT ( 'NONE',  ( 172.7287565553229456, -4.999999999999971578, -36.50000000000000711 ) ) ;
#20651=EDGE_CURVE ( 'NONE', #11863, #19198, #2015, .T. ) ;
#20652=ORIENTED_EDGE ( 'NONE', *, *, #779, .F. ) ;
#20653=EDGE_CURVE ( 'NONE', #11084, #19168, #1703, .T. ) ;
#20654=PLANE ( 'NONE',  #23743 ) ;
#20659=ORIENTED_EDGE ( 'NONE', *, *, #1587, .T. ) ;
#20660=DIRECTION ( 'NONE',  ( 0.3090169943749475623, 8.338696094058001131E-17, 0.9510565162951536422 ) ) ;
#20661=DIRECTION ( 'NONE',  ( -2.698458740408365879E-16, 1.000000000000000000, 0.000000000000000000 ) ) ;
#20664=CARTESIAN_POINT ( 'NONE',  ( 168.6922820468853956, -4.999999999999971578, -32.39392330124607611 ) ) ;
#20665=DIRECTION ( 'NONE',  ( -2.698458740408365879E-16, 1.000000000000000000, 0.000000000000000000 ) ) ;
#20668=EDGE_CURVE ( 'NONE', #14905, #14471, #17803, .T. ) ;
#20669=EDGE_CURVE ( 'NONE', #29571, #12856, #3196, .T. ) ;
#20673=VECTOR ( 'NONE', #21917, 1000.000000000000000 ) ;
#20674=CARTESIAN_POINT ( 'NONE',  ( 157.2287565553229172, -1.999999999999974465, -3.509618943233403510 ) ) ;
#20677=CARTESIAN_POINT ( 'NONE',  ( 172.0152310637604955, -4.999999999999970690, -34.70218595412750773 ) ) ;
#20681=CARTESIAN_POINT ( 'NONE',  ( 158.6922820468853104, -1.999999999999974465, 2.247092850131519715 ) ) ;
#20682=PLANE ( 'NONE',  #14648 ) ;
#20683=LINE ( 'NONE', #27607, #8791 ) ;
#20684=ORIENTED_EDGE ( 'NONE', *, *, #17148, .F. ) ;
#20685=EDGE_CURVE ( 'NONE', #22122, #3594, #8847, .T. ) ;
#20686=ORIENTED_EDGE ( 'NONE', *, *, #9092, .F. ) ;
#20689=ORIENTED_EDGE ( 'NONE', *, *, #27170, .T. ) ;
#20694=VECTOR ( 'NONE', #15295, 1000.000000000000000 ) ;
#20695=ORIENTED_EDGE ( 'NONE', *, *, #24360, .T. ) ;
#20696=CARTESIAN_POINT ( 'NONE',  ( 156.1922820468853956, -4.999999999999975131, -22.25671179336496053 ) ) ;
#20697=LINE ( 'NONE', #16126, #23370 ) ;
#20698=ORIENTED_EDGE ( 'NONE', *, *, #16385, .F. ) ;
#20699=VERTEX_POINT ( 'NONE', #13429 ) ;
#20700=DIRECTION ( 'NONE',  ( -0.5877852522924731371, 0.000000000000000000, 0.8090169943749474513 ) ) ;
#20701=CARTESIAN_POINT ( 'NONE',  ( 142.2287565553230309, -4.999999999999979572, -20.83012701892219454 ) ) ;
#20702=EDGE_CURVE ( 'NONE', #11337, #23759, #13874, .T. ) ;
#20706=ORIENTED_EDGE ( 'NONE', *, *, #21385, .T. ) ;
#20710=FACE_BOUND ( 'NONE', #9343, .T. ) ;
#20711=LINE ( 'NONE', #18437, #18855 ) ;
#20713=PLANE ( 'NONE',  #20257 ) ;
#20714=VECTOR ( 'NONE', #13588, 1000.000000000000000 ) ;
#20717=ORIENTED_EDGE ( 'NONE', *, *, #12072, .T. ) ;
#20718=CARTESIAN_POINT ( 'NONE',  ( 172.7287565553229456, -1.999999999999970468, 6.499999999999977796 ) ) ;
#20719=ORIENTED_EDGE ( 'NONE', *, *, #26826, .T. ) ;
#20723=VERTEX_POINT ( 'NONE', #25195 ) ;
#20726=DIRECTION ( 'NONE',  ( -2.698458740408365879E-16, 1.000000000000000000, 0.000000000000000000 ) ) ;
#20727=VECTOR ( 'NONE', #91, 1000.000000000000000 ) ;
#20730=CARTESIAN_POINT ( 'NONE',  ( 139.7287565553230024, -1.999999999999979128, 0.8205080756887930260 ) ) ;
#20731=CARTESIAN_POINT ( 'NONE',  ( 168.6922820468852819, -4.999999999999971578, 2.247092850131519715 ) ) ;
#20732=VECTOR ( 'NONE', #25317, 1000.000000000000000 ) ;
#20733=VECTOR ( 'NONE', #5569, 1000.000000000000000 ) ;
#20735=EDGE_CURVE ( 'NONE', #2371, #9664, #20294, .T. ) ;
#20738=AXIS2_PLACEMENT_3D ( 'NONE', #23424, #21272, #18536 ) ;
#20740=EDGE_CURVE ( 'NONE', #14836, #22599, #20598, .T. ) ;
#20741=VERTEX_POINT ( 'NONE', #11584 ) ;
#20742=DIRECTION ( 'NONE',  ( 2.908569913943826047E-16, -1.000000000000000000, 6.826925868028107924E-18 ) ) ;
#20743=EDGE_CURVE ( 'NONE', #3603, #4340, #29981, .T. ) ;
#20748=VERTEX_POINT ( 'NONE', #29683 ) ;
#20749=VERTEX_POINT ( 'NONE', #20898 ) ;
#20751=VECTOR ( 'NONE', #23750, 1000.000000000000000 ) ;
#20754=ORIENTED_EDGE ( 'NONE', *, *, #25979, .T. ) ;
#20756=ORIENTED_EDGE ( 'NONE', *, *, #15683, .T. ) ;
#20758=AXIS2_PLACEMENT_3D ( 'NONE', #7420, #26040, #28658 ) ;
#20761=ORIENTED_EDGE ( 'NONE', *, *, #25489, .T. ) ;
#20762=AXIS2_PLACEMENT_3D ( 'NONE', #5109, #14400, #14847 ) ;
#20763=CARTESIAN_POINT ( 'NONE',  ( 137.0152310637606092, -10.00000000000000533, -15.61832212156129351 ) ) ;
#20764=CARTESIAN_POINT ( 'NONE',  ( 110.6987386064946293, -4.999999999999987566, -80.42734139416724304 ) ) ;
#20767=ORIENTED_EDGE ( 'NONE', *, *, #26361, .T. ) ;
#20768=EDGE_CURVE ( 'NONE', #22008, #24060, #16019, .T. ) ;
#20770=EDGE_CURVE ( 'NONE', #2286, #1194, #27819, .T. ) ;
#20771=DIRECTION ( 'NONE',  ( -0.5877852522924731371, -1.586114251531760728E-16, -0.8090169943749474513 ) ) ;
#20772=CARTESIAN_POINT ( 'NONE',  ( 147.2287565553230309, -1.999999999999976241, -29.49038105676660138 ) ) ;
#20774=EDGE_LOOP ( 'NONE', ( #20311, #28316, #16819, #14539 ) ) ;
#20775=EDGE_CURVE ( 'NONE', #17796, #2286, #4136, .T. ) ;
#20776=LINE ( 'NONE', #20934, #13875 ) ;
#20778=CIRCLE ( 'NONE', #7640, 3.000000000000002665 ) ;
#20780=ADVANCED_FACE ( 'NONE', ( #1868 ), #18620, .T. ) ;
#20783=EDGE_CURVE ( 'NONE', #16407, #19094, #18162, .T. ) ;
#20784=CARTESIAN_POINT ( 'NONE',  ( 175.7287565553229456, -4.999999999999970690, -28.21440484423853334 ) ) ;
#20785=EDGE_LOOP ( 'NONE', ( #12296, #13627, #13710, #26580 ) ) ;
#20786=PLANE ( 'NONE',  #23233 ) ;
#20787=ORIENTED_EDGE ( 'NONE', *, *, #9236, .T. ) ;
#20789=ORIENTED_EDGE ( 'NONE', *, *, #29829, .T. ) ;
#20792=CARTESIAN_POINT ( 'NONE',  ( 88.57129075698978227, -4.999999999999992895, 64.35080949528121153 ) ) ;
#20795=EDGE_LOOP ( 'NONE', ( #14742, #19080, #14421, #27981, #7519 ) ) ;
#20796=DIRECTION ( 'NONE',  ( 1.000000000000000000, 2.698458740408365879E-16, -1.110223024625156540E-16 ) ) ;
#20799=DIRECTION ( 'NONE',  ( -1.110223024625156540E-16, 0.000000000000000000, -1.000000000000000000 ) ) ;
#20800=VECTOR ( 'NONE', #25688, 1000.000000000000000 ) ;
#20804=CARTESIAN_POINT ( 'NONE',  ( 24.59515107160807190, -5.000000000000010658, -75.69609154742651924 ) ) ;
#20808=ORIENTED_EDGE ( 'NONE', *, *, #3068, .T. ) ;
#20809=EDGE_CURVE ( 'NONE', #2921, #17847, #22912, .T. ) ;
#20811=DIRECTION ( 'NONE',  ( -0.8090169943749474513, -2.183098979609982436E-16, 0.5877852522924731371 ) ) ;
#20812=CARTESIAN_POINT ( 'NONE',  ( 88.88404763164710687, -4.999999999999992895, 64.57804066564578704 ) ) ;
#20813=LINE ( 'NONE', #25085, #21347 ) ;
#20815=LINE ( 'NONE', #16242, #8008 ) ;
#20816=VECTOR ( 'NONE', #3076, 1000.000000000000000 ) ;
#20817=EDGE_CURVE ( 'NONE', #15401, #21438, #18766, .T. ) ;
#20819=EDGE_CURVE ( 'NONE', #12466, #30027, #16923, .T. ) ;
#20824=VECTOR ( 'NONE', #28335, 1000.000000000000000 ) ;
#20825=PLANE ( 'NONE',  #18535 ) ;
#20826=DIRECTION ( 'NONE',  ( -0.8090169943749474513, -2.183098979609982436E-16, -0.5877852522924731371 ) ) ;
#20827=FACE_OUTER_BOUND ( 'NONE', #27265, .T. ) ;
#20829=VERTEX_POINT ( 'NONE', #26254 ) ;
#20832=EDGE_LOOP ( 'NONE', ( #3701, #25028, #14346, #11991 ) ) ;
#20833=CARTESIAN_POINT ( 'NONE',  ( 168.6922820468853672, -4.999999999999971578, -26.58683881228715862 ) ) ;
#20837=VERTEX_POINT ( 'NONE', #23654 ) ;
#20843=VECTOR ( 'NONE', #13469, 1000.000000000000000 ) ;
#20844=LINE ( 'NONE', #12258, #27943 ) ;
#20846=ADVANCED_FACE ( 'NONE', ( #613 ), #7179, .T. ) ;
#20847=VECTOR ( 'NONE', #8420, 1000.000000000000000 ) ;
#20849=CARTESIAN_POINT ( 'NONE',  ( 153.6922820468853388, -10.00000000000000178, -17.92658477444275533 ) ) ;
#20853=CARTESIAN_POINT ( 'NONE',  ( 136.1922820468854241, -4.999999999999980460, -19.40354224447947473 ) ) ;
#20854=EDGE_CURVE ( 'NONE', #19668, #20364, #162, .T. ) ;
#20855=CARTESIAN_POINT ( 'NONE',  ( 142.2287565553230309, -1.999999999999978018, -29.49038105676660138 ) ) ;
#20859=AXIS2_PLACEMENT_3D ( 'NONE', #14953, #5371, #16960 ) ;
#20860=DIRECTION ( 'NONE',  ( -2.698458740408365879E-16, 1.000000000000000000, 0.000000000000000000 ) ) ;
#20861=CARTESIAN_POINT ( 'NONE',  ( 159.5152310637604671, -9.999999999999998224, -13.05155085951651195 ) ) ;
#20863=FACE_OUTER_BOUND ( 'NONE', #24568, .T. ) ;
#20864=LINE ( 'NONE', #13706, #5151 ) ;
#20866=VECTOR ( 'NONE', #25931, 1000.000000000000000 ) ;
#20867=DIRECTION ( 'NONE',  ( -2.698458740408365879E-16, 1.000000000000000000, 0.000000000000000000 ) ) ;
#20868=CARTESIAN_POINT ( 'NONE',  ( 177.2287565553228319, -9.999999999999994671, -3.509618943233403510 ) ) ;
#20869=ORIENTED_EDGE ( 'NONE', *, *, #17005, .T. ) ;
#20870=ORIENTED_EDGE ( 'NONE', *, *, #15518, .T. ) ;
#20871=LINE ( 'NONE', #27946, #11558 ) ;
#20872=VECTOR ( 'NONE', #7161, 1000.000000000000000 ) ;
#20875=AXIS2_PLACEMENT_3D ( 'NONE', #26988, #3762, #23810 ) ;
#20879=LINE ( 'NONE', #14157, #6752 ) ;
#20880=CARTESIAN_POINT ( 'NONE',  ( 152.0152310637604955, -10.00000000000000178, -8.721423840594312082 ) ) ;
#20881=CARTESIAN_POINT ( 'NONE',  ( 166.1922820468853104, -4.999999999999972466, -2.083034168790677043 ) ) ;
#20885=CARTESIAN_POINT ( 'NONE',  ( 7.738597516018001166, -5.000000000000015987, 23.81695417587389940 ) ) ;
#20886=DIRECTION ( 'NONE',  ( -0.9510565162951536422, 0.000000000000000000, -0.3090169943749472292 ) ) ;
#20887=VECTOR ( 'NONE', #3873, 1000.000000000000000 ) ;
#20889=CARTESIAN_POINT ( 'NONE',  ( 161.1922820468853672, -9.999999999999998224, -19.40354224447947828 ) ) ;
#20890=DIRECTION ( 'NONE',  ( -2.698458740408365879E-16, 1.000000000000000000, 0.000000000000000000 ) ) ;
#20891=VECTOR ( 'NONE', #29484, 1000.000000000000000 ) ;
#20895=ORIENTED_EDGE ( 'NONE', *, *, #8660, .F. ) ;
#20897=ORIENTED_EDGE ( 'NONE', *, *, #10800, .F. ) ;
#20898=CARTESIAN_POINT ( 'NONE',  ( 131.1922820468854241, -4.999999999999982236, -19.40354224447947473 ) ) ;
#20905=DIRECTION ( 'NONE',  ( -1.110223024625156540E-16, 0.000000000000000000, -1.000000000000000000 ) ) ;
#20907=LINE ( 'NONE', #19, #6396 ) ;
#20908=DIRECTION ( 'NONE',  ( -2.698458740408365879E-16, 1.000000000000000000, 0.000000000000000000 ) ) ;
#20909=ORIENTED_EDGE ( 'NONE', *, *, #22070, .T. ) ;
#20911=EDGE_LOOP ( 'NONE', ( #28051, #27008, #10157, #17130 ) ) ;
#20916=ORIENTED_EDGE ( 'NONE', *, *, #8530, .F. ) ;
#20917=DIRECTION ( 'NONE',  ( 2.908569913943825061E-16, -1.000000000000000000, -6.826925868028081731E-18 ) ) ;
#20918=VERTEX_POINT ( 'NONE', #28120 ) ;
#20921=EDGE_CURVE ( 'NONE', #288, #1987, #16471, .T. ) ;
#20922=EDGE_CURVE ( 'NONE', #2898, #24422, #16628, .T. ) ;
#20927=ORIENTED_EDGE ( 'NONE', *, *, #20579, .F. ) ;
#20928=CARTESIAN_POINT ( 'NONE',  ( 153.6922820468854241, -10.00000000000000000, -26.58683881228715862 ) ) ;
#20929=VERTEX_POINT ( 'NONE', #14174 ) ;
#20930=DIRECTION ( 'NONE',  ( -0.9510565162951536422, 0.000000000000000000, -0.3090169943749472292 ) ) ;
#20931=VECTOR ( 'NONE', #27493, 1000.000000000000000 ) ;
#20932=CARTESIAN_POINT ( 'NONE',  ( 131.1922820468854241, -4.999999999999982236, -22.25671179336495697 ) ) ;
#20934=CARTESIAN_POINT ( 'NONE',  ( 133.6922820468854241, -10.00000000000000711, -6.413161187712875133 ) ) ;
#20935=AXIS2_PLACEMENT_3D ( 'NONE', #4248, #4683, #18118 ) ;
#20937=DIRECTION ( 'NONE',  ( 0.3090169943749472292, 8.338696094057992503E-17, -0.9510565162951536422 ) ) ;
#20938=DIRECTION ( 'NONE',  ( 0.5877852522924731371, 1.586114251531760728E-16, 0.8090169943749474513 ) ) ;
#20939=ORIENTED_EDGE ( 'NONE', *, *, #27764, .F. ) ;
#20943=CARTESIAN_POINT ( 'NONE',  ( 156.1922820468853956, -1.999999999999974465, -22.25671179336496053 ) ) ;
#20944=LINE ( 'NONE', #208, #30132 ) ;
#20945=EDGE_LOOP ( 'NONE', ( #5747, #23651, #25696, #4526 ) ) ;
#20947=ORIENTED_EDGE ( 'NONE', *, *, #2861, .T. ) ;
#20948=EDGE_LOOP ( 'NONE', ( #29998, #15086, #8199, #23059, #22191 ) ) ;
#20953=EDGE_LOOP ( 'NONE', ( #26184, #8259, #16146, #24424 ) ) ;
#20956=ORIENTED_EDGE ( 'NONE', *, *, #19686, .T. ) ;
#20958=DIRECTION ( 'NONE',  ( 0.9510565162951536422, 2.566386769018988816E-16, 0.3090169943749472292 ) ) ;
#20960=VECTOR ( 'NONE', #5534, 1000.000000000000000 ) ;
#20963=EDGE_CURVE ( 'NONE', #30260, #14083, #7475, .T. ) ;
#20964=ADVANCED_FACE ( 'NONE', ( #25797 ), #23500, .T. ) ;
#20965=VERTEX_POINT ( 'NONE', #26102 ) ;
#20971=DIRECTION ( 'NONE',  ( -1.110223024625156540E-16, 0.000000000000000000, -1.000000000000000000 ) ) ;
#20972=VECTOR ( 'NONE', #28012, 999.9999999999998863 ) ;
#20973=PLANE ( 'NONE',  #21156 ) ;
#20978=ORIENTED_EDGE ( 'NONE', *, *, #16410, .T. ) ;
#20981=FACE_OUTER_BOUND ( 'NONE', #19032, .T. ) ;
#20982=CARTESIAN_POINT ( 'NONE',  ( 168.6922820468853672, -1.999999999999970912, -26.58683881228715862 ) ) ;
#20983=DIRECTION ( 'NONE',  ( -2.698458740408365879E-16, 1.000000000000000000, 0.000000000000000000 ) ) ;
#20985=ORIENTED_EDGE ( 'NONE', *, *, #20036, .F. ) ;
#20986=ORIENTED_EDGE ( 'NONE', *, *, #26433, .F. ) ;
#20987=DIRECTION ( 'NONE',  ( 0.9510565162951535312, 2.566386769018988816E-16, -0.3090169943749475623 ) ) ;
#20990=FACE_OUTER_BOUND ( 'NONE', #7831, .T. ) ;
#20991=LINE ( 'NONE', #23751, #2031 ) ;
#20993=ORIENTED_EDGE ( 'NONE', *, *, #7399, .T. ) ;
#20995=ORIENTED_EDGE ( 'NONE', *, *, #25040, .F. ) ;
#20997=AXIS2_PLACEMENT_3D ( 'NONE', #9406, #4841, #14139 ) ;
#20999=VECTOR ( 'NONE', #10846, 1000.000000000000000 ) ;
#21002=EDGE_CURVE ( 'NONE', #26592, #11825, #3061, .T. ) ;
#21004=EDGE_CURVE ( 'NONE', #2921, #12148, #9441, .T. ) ;
#21006=ADVANCED_FACE ( 'NONE', ( #28565 ), #748, .T. ) ;
#21009=CARTESIAN_POINT ( 'NONE',  ( 134.7287565553230024, -1.999999999999980460, -33.82050807568879947 ) ) ;
#21011=EDGE_LOOP ( 'NONE', ( #11688, #15835, #9976, #24714 ) ) ;
#21012=CARTESIAN_POINT ( 'NONE',  ( 132.0152310637605524, -4.999999999999982236, -0.06116980274991495881 ) ) ;
#21013=VECTOR ( 'NONE', #14853, 1000.000000000000000 ) ;
#21014=DIRECTION ( 'NONE',  ( -0.9510565162951536422, -2.566386769018988323E-16, 0.3090169943749475623 ) ) ;
#21016=VECTOR ( 'NONE', #26500, 1000.000000000000000 ) ;
#21018=ORIENTED_EDGE ( 'NONE', *, *, #11568, .F. ) ;
#21019=DIRECTION ( 'NONE',  ( 0.3090169943749475623, 8.338696094058001131E-17, 0.9510565162951536422 ) ) ;
#21020=LINE ( 'NONE', #125, #27035 ) ;
#21024=LINE ( 'NONE', #15264, #25140 ) ;
#21026=ORIENTED_EDGE ( 'NONE', *, *, #22317, .F. ) ;
#21027=DIRECTION ( 'NONE',  ( 1.110223024625156540E-16, 2.995891024602366092E-32, 1.000000000000000000 ) ) ;
#21028=ORIENTED_EDGE ( 'NONE', *, *, #5784, .T. ) ;
#21029=PLANE ( 'NONE',  #9282 ) ;
#21030=ORIENTED_EDGE ( 'NONE', *, *, #2009, .F. ) ;
#21031=DIRECTION ( 'NONE',  ( -0.9510565162951536422, 0.000000000000000000, -0.3090169943749472292 ) ) ;
#21032=ORIENTED_EDGE ( 'NONE', *, *, #15969, .F. ) ;
#21036=ORIENTED_EDGE ( 'NONE', *, *, #4611, .F. ) ;
#21038=DIRECTION ( 'NONE',  ( 0.5877852522924731371, 1.586114251531760728E-16, 0.8090169943749474513 ) ) ;
#21039=CARTESIAN_POINT ( 'NONE',  ( 148.6922820468853672, -4.999999999999978684, -0.6060766987539614181 ) ) ;
#21040=DIRECTION ( 'NONE',  ( 0.9510565162951535312, 2.566386769018988816E-16, -0.3090169943749475623 ) ) ;
#21041=EDGE_CURVE ( 'NONE', #18400, #21232, #29612, .T. ) ;
#21042=VECTOR ( 'NONE', #4178, 1000.000000000000000 ) ;
#21044=ORIENTED_EDGE ( 'NONE', *, *, #8281, .T. ) ;
#21047=VECTOR ( 'NONE', #17435, 1000.000000000000000 ) ;
#21048=DIRECTION ( 'NONE',  ( 0.9510565162951536422, 2.566386769018988816E-16, 0.3090169943749472292 ) ) ;
#21049=CARTESIAN_POINT ( 'NONE',  ( 133.7287565553229456, -1.999999999999980904, 6.499999999999978684 ) ) ;
#21051=DIRECTION ( 'NONE',  ( 0.9510565162951535312, 2.566386769018988816E-16, -0.3090169943749475623 ) ) ;
#21056=DIRECTION ( 'NONE',  ( -2.698458740408365879E-16, 1.000000000000000000, 0.000000000000000000 ) ) ;
#21057=VECTOR ( 'NONE', #21338, 999.9999999999998863 ) ;
#21060=LINE ( 'NONE', #28569, #18497 ) ;
#21061=VERTEX_POINT ( 'NONE', #1330 ) ;
#21063=ORIENTED_EDGE ( 'NONE', *, *, #4908, .T. ) ;
#21065=CARTESIAN_POINT ( 'NONE',  ( 172.0152310637604671, -1.999999999999969580, -26.04193191628311155 ) ) ;
#21067=CARTESIAN_POINT ( 'NONE',  ( 157.0152310637605240, -1.999999999999973577, -26.04193191628311155 ) ) ;
#21068=DIRECTION ( 'NONE',  ( -2.698458740408365879E-16, 1.000000000000000000, 0.000000000000000000 ) ) ;
#21069=VERTEX_POINT ( 'NONE', #12907 ) ;
#21070=PLANE ( 'NONE',  #27672 ) ;
#21076=AXIS2_PLACEMENT_3D ( 'NONE', #3979, #22597, #20591 ) ;
#21077=VERTEX_POINT ( 'NONE', #6504 ) ;
#21078=CARTESIAN_POINT ( 'NONE',  ( 159.5152310637605240, -1.999999999999972689, -30.37205893520531319 ) ) ;
#21079=ORIENTED_EDGE ( 'NONE', *, *, #2786, .F. ) ;
#21085=EDGE_LOOP ( 'NONE', ( #9205, #1279, #29207, #998, #17854 ) ) ;
#21086=FACE_BOUND ( 'NONE', #16672, .T. ) ;
#21088=LINE ( 'NONE', #16353, #1927 ) ;
#21089=VECTOR ( 'NONE', #1698, 1000.000000000000000 ) ;
#21090=CARTESIAN_POINT ( 'NONE',  ( 146.1922820468853956, -4.999999999999978684, -2.083034168790677043 ) ) ;
#21092=DIRECTION ( 'NONE',  ( -0.9510565162951536422, -2.566386769018988323E-16, 0.3090169943749475623 ) ) ;
#21094=EDGE_CURVE ( 'NONE', #15830, #5025, #3918, .T. ) ;
#21095=LINE ( 'NONE', #5221, #19325 ) ;
#21096=ORIENTED_EDGE ( 'NONE', *, *, #11030, .T. ) ;
#21099=ORIENTED_EDGE ( 'NONE', *, *, #16699, .T. ) ;
#21100=VECTOR ( 'NONE', #8804, 999.9999999999998863 ) ;
#21102=LINE ( 'NONE', #18510, #17080 ) ;
#21103=DIRECTION ( 'NONE',  ( -2.698458740408365879E-16, 1.000000000000000000, 0.000000000000000000 ) ) ;
#21105=ORIENTED_EDGE ( 'NONE', *, *, #20166, .F. ) ;
#21110=DIRECTION ( 'NONE',  ( -1.000000000000000000, -2.908569913943825554E-16, 0.000000000000000000 ) ) ;
#21111=ORIENTED_EDGE ( 'NONE', *, *, #19893, .F. ) ;
#21112=LINE ( 'NONE', #218, #13996 ) ;
#21114=VERTEX_POINT ( 'NONE', #29462 ) ;
#21115=DIRECTION ( 'NONE',  ( 0.3090169943749475623, 8.338696094058001131E-17, 0.9510565162951536422 ) ) ;
#21118=ORIENTED_EDGE ( 'NONE', *, *, #1590, .T. ) ;
#21119=ORIENTED_EDGE ( 'NONE', *, *, #4123, .F. ) ;
#21122=CARTESIAN_POINT ( 'NONE',  ( 134.7287565553230024, -10.00000000000000711, -25.16025403784439973 ) ) ;
#21123=CARTESIAN_POINT ( 'NONE',  ( 168.6922820468853388, -9.999999999999996447, -15.07341522555727664 ) ) ;
#21124=CARTESIAN_POINT ( 'NONE',  ( 164.5152310637604955, -4.999999999999973355, -1.826485974285146869E-14 ) ) ;
#21125=FACE_OUTER_BOUND ( 'NONE', #29598, .T. ) ;
#21131=EDGE_LOOP ( 'NONE', ( #10538, #29071, #6964, #25427 ) ) ;
#21132=LINE ( 'NONE', #11507, #29080 ) ;
#21134=EDGE_CURVE ( 'NONE', #8261, #28996, #1638, .T. ) ;
#21135=DIRECTION ( 'NONE',  ( -2.698458740408365879E-16, 1.000000000000000000, 0.000000000000000000 ) ) ;
#21136=CARTESIAN_POINT ( 'NONE',  ( 111.4790881585512494, -4.999999999999986677, 80.99429853044631500 ) ) ;
#21137=EDGE_CURVE ( 'NONE', #27103, #9856, #6359, .T. ) ;
#21139=DIRECTION ( 'NONE',  ( 1.000000000000000000, 2.698458740408365879E-16, -1.110223024625156540E-16 ) ) ;
#21141=VERTEX_POINT ( 'NONE', #15190 ) ;
#21142=CARTESIAN_POINT ( 'NONE',  ( 169.5152310637604955, -4.999999999999971578, -1.881997125516404696E-14 ) ) ;
#21143=DIRECTION ( 'NONE',  ( 1.000000000000000000, 0.000000000000000000, 0.000000000000000000 ) ) ;
#21151=VERTEX_POINT ( 'NONE', #15339 ) ;
#21152=CARTESIAN_POINT ( 'NONE',  ( 81.91613614387523512, -4.999999999999995559, 59.51555663840242261 ) ) ;
#21153=DIRECTION ( 'NONE',  ( 0.3090169943749472292, 8.338696094057992503E-17, -0.9510565162951536422 ) ) ;
#21154=ORIENTED_EDGE ( 'NONE', *, *, #13686, .F. ) ;
#21155=FACE_OUTER_BOUND ( 'NONE', #69, .T. ) ;
#21156=AXIS2_PLACEMENT_3D ( 'NONE', #6801, #9362, #2229 ) ;
#21157=CARTESIAN_POINT ( 'NONE',  ( 157.0152310637605524, -1.999999999999973577, -24.27857615940569502 ) ) ;
#21160=ORIENTED_EDGE ( 'NONE', *, *, #16064, .F. ) ;
#21161=EDGE_CURVE ( 'NONE', #21674, #23858, #4067, .T. ) ;
#21162=CARTESIAN_POINT ( 'NONE',  ( 157.0152310637604671, -10.00000000000000000, 1.702185954127501066 ) ) ;
#21164=EDGE_CURVE ( 'NONE', #8863, #9240, #29298, .T. ) ;
#21166=EDGE_CURVE ( 'NONE', #5527, #28746, #13510, .T. ) ;
#21168=LINE ( 'NONE', #18585, #24396 ) ;
#21169=EDGE_CURVE ( 'NONE', #3207, #968, #11225, .T. ) ;
#21170=PLANE ( 'NONE',  #8133 ) ;
#21171=EDGE_LOOP ( 'NONE', ( #18182, #24874, #6727, #9457 ) ) ;
#21173=CARTESIAN_POINT ( 'NONE',  ( 134.5152310637605808, -1.999999999999980460, -2.627941064794695691 ) ) ;
#21176=VERTEX_POINT ( 'NONE', #29913 ) ;
#21181=CARTESIAN_POINT ( 'NONE',  ( 146.1922820468854525, -1.999999999999976685, -28.06379628232387446 ) ) ;
#21184=DIRECTION ( 'NONE',  ( -0.8090169943749474513, -2.183098979609982436E-16, -0.5877852522924731371 ) ) ;
#21186=ORIENTED_EDGE ( 'NONE', *, *, #28106, .F. ) ;
#21187=CARTESIAN_POINT ( 'NONE',  ( 100.1455277581281536, -4.999999999999990230, -72.75998490582146871 ) ) ;
#21188=DIRECTION ( 'NONE',  ( -2.698458740408365879E-16, 1.000000000000000000, 0.000000000000000000 ) ) ;
#21189=DIRECTION ( 'NONE',  ( 0.000000000000000000, 0.000000000000000000, -1.000000000000000000 ) ) ;
#21190=DIRECTION ( 'NONE',  ( 0.3090169943749472292, 8.338696094057992503E-17, -0.9510565162951536422 ) ) ;
#21191=DIRECTION ( 'NONE',  ( 0.5877852522924731371, 0.000000000000000000, 0.8090169943749474513 ) ) ;
#21196=ORIENTED_EDGE ( 'NONE', *, *, #29954, .T. ) ;
#21197=ADVANCED_FACE ( 'NONE', ( #1488 ), #10622, .T. ) ;
#21198=DIRECTION ( 'NONE',  ( -2.698458740408365879E-16, 1.000000000000000000, 0.000000000000000000 ) ) ;
#21201=EDGE_CURVE ( 'NONE', #16627, #20539, #28203, .T. ) ;
#21203=FACE_BOUND ( 'NONE', #3879, .T. ) ;
#21204=EDGE_CURVE ( 'NONE', #2119, #6518, #21132, .T. ) ;
#21205=ORIENTED_EDGE ( 'NONE', *, *, #15479, .F. ) ;
#21206=ORIENTED_EDGE ( 'NONE', *, *, #25417, .F. ) ;
#21208=CARTESIAN_POINT ( 'NONE',  ( 139.5152310637605808, -10.00000000000000533, -13.05155085951651195 ) ) ;
#21211=LINE ( 'NONE', #27980, #21325 ) ;
#21212=ORIENTED_EDGE ( 'NONE', *, *, #23242, .F. ) ;
#21213=ORIENTED_EDGE ( 'NONE', *, *, #25976, .T. ) ;
#21214=CARTESIAN_POINT ( 'NONE',  ( 153.6922820468853104, -1.999999999999975797, 2.247092850131521491 ) ) ;
#21215=ORIENTED_EDGE ( 'NONE', *, *, #2351, .F. ) ;
#21221=ORIENTED_EDGE ( 'NONE', *, *, #29241, .T. ) ;
#21228=ORIENTED_EDGE ( 'NONE', *, *, #2179, .T. ) ;
#21229=EDGE_CURVE ( 'NONE', #29062, #16025, #25422, .T. ) ;
#21230=FACE_BOUND ( 'NONE', #28952, .T. ) ;
#21232=VERTEX_POINT ( 'NONE', #16557 ) ;
#21233=AXIS2_PLACEMENT_3D ( 'NONE', #15342, #10921, #10625 ) ;
#21234=CARTESIAN_POINT ( 'NONE',  ( 167.0152310637604387, -9.999999999999998224, 1.702185954127501066 ) ) ;
#21235=CARTESIAN_POINT ( 'NONE',  ( 157.0152310637605524, -1.999999999999973577, -24.27857615940569502 ) ) ;
#21236=DIRECTION ( 'NONE',  ( -0.9510565162951536422, -2.566386769018988816E-16, -0.3090169943749472292 ) ) ;
#21237=VECTOR ( 'NONE', #27351, 1000.000000000000000 ) ;
#21239=LINE ( 'NONE', #201, #22920 ) ;
#21240=ORIENTED_EDGE ( 'NONE', *, *, #1242, .T. ) ;
#21243=AXIS2_PLACEMENT_3D ( 'NONE', #5425, #24054, #11671 ) ;
#21247=VECTOR ( 'NONE', #10378, 1000.000000000000000 ) ;
#21249=FACE_OUTER_BOUND ( 'NONE', #4400, .T. ) ;
#21252=ORIENTED_EDGE ( 'NONE', *, *, #2594, .F. ) ;
#21253=LINE ( 'NONE', #7075, #6664 ) ;
#21255=VERTEX_POINT ( 'NONE', #25883 ) ;
#21258=CARTESIAN_POINT ( 'NONE',  ( 172.7287565553229456, -9.999999999999971578, -33.50000000000000000 ) ) ;
#21260=ORIENTED_EDGE ( 'NONE', *, *, #6342, .F. ) ;
#21267=LINE ( 'NONE', #14541, #1490 ) ;
#21268=AXIS2_PLACEMENT_3D ( 'NONE', #9001, #1877, #20306 ) ;
#21270=VECTOR ( 'NONE', #4715, 1000.000000000000000 ) ;
#21271=CARTESIAN_POINT ( 'NONE',  ( 164.5152310637604387, -9.999999999999998224, -4.391296821672111328 ) ) ;
#21272=DIRECTION ( 'NONE',  ( -0.8090169943749474513, -2.183098979609982436E-16, 0.5877852522924731371 ) ) ;
#21273=LINE ( 'NONE', #7251, #20392 ) ;
#21274=LINE ( 'NONE', #384, #26087 ) ;
#21280=ORIENTED_EDGE ( 'NONE', *, *, #24076, .T. ) ;
#21282=CARTESIAN_POINT ( 'NONE',  ( 154.5152310637605524, -4.999999999999976019, -19.94844914048349693 ) ) ;
#21284=LINE ( 'NONE', #28361, #7866 ) ;
#21285=LINE ( 'NONE', #14709, #20727 ) ;
#21287=ORIENTED_EDGE ( 'NONE', *, *, #9758, .T. ) ;
#21290=ORIENTED_EDGE ( 'NONE', *, *, #1109, .F. ) ;
#21292=DIRECTION ( 'NONE',  ( 1.000000000000000000, 2.698458740408365879E-16, -1.110223024625156540E-16 ) ) ;
#21293=DIRECTION ( 'NONE',  ( -0.9510565162951536422, -2.566386769018988323E-16, 0.3090169943749475623 ) ) ;
#21294=ORIENTED_EDGE ( 'NONE', *, *, #8271, .F. ) ;
#21295=VECTOR ( 'NONE', #23782, 1000.000000000000000 ) ;
#21297=ORIENTED_EDGE ( 'NONE', *, *, #17622, .T. ) ;
#21299=ORIENTED_EDGE ( 'NONE', *, *, #5086, .T. ) ;
#21304=EDGE_CURVE ( 'NONE', #11783, #27678, #19001, .T. ) ;
#21308=EDGE_CURVE ( 'NONE', #28060, #25015, #16857, .T. ) ;
#21309=CARTESIAN_POINT ( 'NONE',  ( 175.7287565553229172, -4.999999999999970690, -30.76635726929469783 ) ) ;
#21310=LINE ( 'NONE', #26060, #27788 ) ;
#21311=LINE ( 'NONE', #28231, #2666 ) ;
#21312=PLANE ( 'NONE',  #20460 ) ;
#21316=LINE ( 'NONE', #21162, #5915 ) ;
#21317=DIRECTION ( 'NONE',  ( -0.5877852522924731371, -1.586114251531760235E-16, 0.8090169943749474513 ) ) ;
#21319=CARTESIAN_POINT ( 'NONE',  ( 175.7287565553229456, -4.999999999999970690, -30.76635726929468362 ) ) ;
#21320=VERTEX_POINT ( 'NONE', #21591 ) ;
#21321=DIRECTION ( 'NONE',  ( -0.9510565162951536422, 0.000000000000000000, -0.3090169943749472292 ) ) ;
#21323=VERTEX_POINT ( 'NONE', #12125 ) ;
#21324=CARTESIAN_POINT ( 'NONE',  ( 151.1922820468854241, -10.00000000000000178, -19.40354224447947828 ) ) ;
#21325=VECTOR ( 'NONE', #23360, 1000.000000000000000 ) ;
#21326=PLANE ( 'NONE',  #15610 ) ;
#21328=DIRECTION ( 'NONE',  ( -0.5877852522924731371, -1.586114251531760235E-16, 0.8090169943749474513 ) ) ;
#21329=ORIENTED_EDGE ( 'NONE', *, *, #1458, .F. ) ;
#21333=VECTOR ( 'NONE', #28935, 1000.000000000000000 ) ;
#21336=CARTESIAN_POINT ( 'NONE',  ( 143.6922820468854525, -1.999999999999978018, -35.24709285013155835 ) ) ;
#21337=LINE ( 'NONE', #28407, #16500 ) ;
#21338=DIRECTION ( 'NONE',  ( -0.9510565162951536422, -2.566386769018988323E-16, 0.3090169943749475623 ) ) ;
#21340=EDGE_CURVE ( 'NONE', #13044, #25090, #26035, .T. ) ;
#21341=EDGE_CURVE ( 'NONE', #27148, #28119, #23900, .T. ) ;
#21343=DIRECTION ( 'NONE',  ( 6.938893903907227392E-16, -0.000000000000000000, 1.000000000000000000 ) ) ;
#21345=FACE_OUTER_BOUND ( 'NONE', #21752, .T. ) ;
#21346=CARTESIAN_POINT ( 'NONE',  ( 172.0152310637604671, -4.999999999999970690, -15.61832212156129707 ) ) ;
#21347=VECTOR ( 'NONE', #9608, 1000.000000000000000 ) ;
#21351=LINE ( 'NONE', #9895, #16989 ) ;
#21354=EDGE_LOOP ( 'NONE', ( #20400, #14349, #28188, #10513 ) ) ;
#21356=ORIENTED_EDGE ( 'NONE', *, *, #155, .T. ) ;
#21360=CARTESIAN_POINT ( 'NONE',  ( 159.5152310637604671, -1.999999999999973577, -13.05155085951651195 ) ) ;
#21361=ORIENTED_EDGE ( 'NONE', *, *, #1376, .F. ) ;
#21363=DIRECTION ( 'NONE',  ( -2.698458740408365879E-16, 1.000000000000000000, 0.000000000000000000 ) ) ;
#21365=DIRECTION ( 'NONE',  ( -0.5877852522924731371, -1.586114251531760235E-16, 0.8090169943749474513 ) ) ;
#21366=VERTEX_POINT ( 'NONE', #17301 ) ;
#21368=ORIENTED_EDGE ( 'NONE', *, *, #21201, .T. ) ;
#21370=EDGE_LOOP ( 'NONE', ( #11901, #71, #18626, #11145 ) ) ;
#21374=VERTEX_POINT ( 'NONE', #21439 ) ;
#21375=EDGE_LOOP ( 'NONE', ( #2220, #15828, #6536, #6093, #23907 ) ) ;
#21377=ORIENTED_EDGE ( 'NONE', *, *, #26644, .T. ) ;
#21378=CARTESIAN_POINT ( 'NONE',  ( 177.2287565553228887, -9.999999999999994671, -20.83012701892220520 ) ) ;
#21381=VECTOR ( 'NONE', #20395, 1000.000000000000000 ) ;
#21383=ADVANCED_FACE ( 'NONE', ( #22042 ), #24191, .T. ) ;
#21385=EDGE_CURVE ( 'NONE', #16231, #486, #19588, .T. ) ;
#21387=EDGE_CURVE ( 'NONE', #13253, #3275, #3144, .T. ) ;
#21388=ORIENTED_EDGE ( 'NONE', *, *, #25451, .F. ) ;
#21389=FACE_BOUND ( 'NONE', #14516, .T. ) ;
#21391=ORIENTED_EDGE ( 'NONE', *, *, #9165, .T. ) ;
#21392=DIRECTION ( 'NONE',  ( 0.9510565162951536422, 2.566386769018988816E-16, 0.3090169943749472292 ) ) ;
#21393=CARTESIAN_POINT ( 'NONE',  ( 167.0152310637604387, -4.999999999999972466, -1.854241549900775151E-14 ) ) ;
#21394=LINE ( 'NONE', #14052, #25309 ) ;
#21395=LINE ( 'NONE', #21688, #12902 ) ;
#21397=CARTESIAN_POINT ( 'NONE',  ( 169.5152310637605240, -9.999999999999994671, -28.60870317832789667 ) ) ;
#21399=VECTOR ( 'NONE', #14658, 1000.000000000000000 ) ;
#21400=CARTESIAN_POINT ( 'NONE',  ( 147.0152310637606092, -1.999999999999976241, -24.27857615940569502 ) ) ;
#21403=ORIENTED_EDGE ( 'NONE', *, *, #10939, .T. ) ;
#21405=LINE ( 'NONE', #28925, #14127 ) ;
#21408=VECTOR ( 'NONE', #21189, 1000.000000000000000 ) ;
#21411=ORIENTED_EDGE ( 'NONE', *, *, #24702, .F. ) ;
#21415=DIRECTION ( 'NONE',  ( -2.698458740408365879E-16, 1.000000000000000000, 0.000000000000000000 ) ) ;
#21418=ORIENTED_EDGE ( 'NONE', *, *, #20768, .F. ) ;
#21419=CARTESIAN_POINT ( 'NONE',  ( 131.1922820468854241, -10.00000000000000888, -30.91696583120935671 ) ) ;
#21422=VERTEX_POINT ( 'NONE', #12419 ) ;
#21423=LINE ( 'NONE', #12108, #14245 ) ;
#21425=EDGE_CURVE ( 'NONE', #21526, #10703, #24335, .T. ) ;
#21426=ORIENTED_EDGE ( 'NONE', *, *, #8919, .F. ) ;
#21427=LINE ( 'NONE', #9962, #17647 ) ;
#21428=AXIS2_PLACEMENT_3D ( 'NONE', #14322, #16631, #9902 ) ;
#21429=LINE ( 'NONE', #16846, #10394 ) ;
#21430=AXIS2_PLACEMENT_3D ( 'NONE', #24252, #5780, #5629 ) ;
#21431=LINE ( 'NONE', #3284, #11061 ) ;
#21432=DIRECTION ( 'NONE',  ( -2.698458740408365879E-16, 1.000000000000000000, 0.000000000000000000 ) ) ;
#21438=VERTEX_POINT ( 'NONE', #19292 ) ;
#21439=CARTESIAN_POINT ( 'NONE',  ( 137.2287565553230309, -4.999999999999980460, -29.49038105676659427 ) ) ;
#21441=CARTESIAN_POINT ( 'NONE',  ( 154.7287565553229172, -10.00000000000000178, -16.50000000000000000 ) ) ;
#21442=DIRECTION ( 'NONE',  ( -2.698458740408365879E-16, 1.000000000000000000, 0.000000000000000000 ) ) ;
#21446=DIRECTION ( 'NONE',  ( -2.698458740408365879E-16, 1.000000000000000000, 0.000000000000000000 ) ) ;
#21450=CARTESIAN_POINT ( 'NONE',  ( 133.7287565553229456, -84.33034373659253902, -33.50000000000000000 ) ) ;
#21451=DIRECTION ( 'NONE',  ( -1.110223024625156540E-16, 0.000000000000000000, -1.000000000000000000 ) ) ;
#21452=VECTOR ( 'NONE', #20516, 1000.000000000000000 ) ;
#21455=VERTEX_POINT ( 'NONE', #1146 ) ;
#21460=VECTOR ( 'NONE', #15155, 1000.000000000000000 ) ;
#21461=AXIS2_PLACEMENT_3D ( 'NONE', #24950, #10588, #29426 ) ;
#21462=ORIENTED_EDGE ( 'NONE', *, *, #26053, .T. ) ;
#21463=ORIENTED_EDGE ( 'NONE', *, *, #10520, .T. ) ;
#21464=DIRECTION ( 'NONE',  ( -1.000000000000000000, -2.891205793294689173E-16, 0.000000000000000000 ) ) ;
#21471=LINE ( 'NONE', #11851, #15638 ) ;
#21472=CARTESIAN_POINT ( 'NONE',  ( 146.1922820468854525, -1.999999999999976685, -19.40354224447947828 ) ) ;
#21474=CARTESIAN_POINT ( 'NONE',  ( 171.1922820468853104, -4.999999999999971578, -13.59645775552055902 ) ) ;
#21475=DIRECTION ( 'NONE',  ( 1.000000000000000000, 2.698458740408365879E-16, -1.110223024625156540E-16 ) ) ;
#21476=VECTOR ( 'NONE', #7746, 1000.000000000000000 ) ;
#21478=ADVANCED_FACE ( 'NONE', ( #3429 ), #19148, .T. ) ;
#21479=ORIENTED_EDGE ( 'NONE', *, *, #6778, .T. ) ;
#21481=DIRECTION ( 'NONE',  ( 0.3090169943749475623, 8.338696094058001131E-17, 0.9510565162951536422 ) ) ;
#21482=EDGE_CURVE ( 'NONE', #29149, #28465, #29724, .T. ) ;
#21483=CARTESIAN_POINT ( 'NONE',  ( 162.0152310637604671, -4.999999999999974243, -1.798730398669517640E-14 ) ) ;
#21487=EDGE_LOOP ( 'NONE', ( #29623, #16598, #12996, #28861 ) ) ;
#21489=STYLED_ITEM ( 'NONE', ( #13199 ), #13457 ) ;
#21492=DIRECTION ( 'NONE',  ( 0.5877852522924731371, 1.586114251531760728E-16, -0.8090169943749474513 ) ) ;
#21493=DIRECTION ( 'NONE',  ( 0.9510565162951535312, 2.566386769018988816E-16, -0.3090169943749475623 ) ) ;
#21494=CARTESIAN_POINT ( 'NONE',  ( 149.5152310637605808, -1.999999999999975797, -19.94844914048349693 ) ) ;
#21495=CARTESIAN_POINT ( 'NONE',  ( 171.1922820468852819, -1.999999999999970912, -2.083034168790677043 ) ) ;
#21497=CARTESIAN_POINT ( 'NONE',  ( 136.1922820468854241, -10.00000000000000533, -28.06379628232387446 ) ) ;
#21499=PLANE ( 'NONE',  #29756 ) ;
#21501=LINE ( 'NONE', #9286, #1995 ) ;
#21502=CARTESIAN_POINT ( 'NONE',  ( 147.0152310637605524, -4.999999999999977796, -1.632196944975745105E-14 ) ) ;
#21506=ORIENTED_EDGE ( 'NONE', *, *, #10827, .T. ) ;
#21508=DIRECTION ( 'NONE',  ( -2.698458740408365879E-16, 1.000000000000000000, 0.000000000000000000 ) ) ;
#21511=LINE ( 'NONE', #5184, #17044 ) ;
#21512=ADVANCED_FACE ( 'NONE', ( #29103 ), #4026, .T. ) ;
#21513=ORIENTED_EDGE ( 'NONE', *, *, #16619, .T. ) ;
#21519=DIRECTION ( 'NONE',  ( 0.5877852522924731371, 0.000000000000000000, 0.8090169943749474513 ) ) ;
#21520=EDGE_CURVE ( 'NONE', #2375, #12138, #15612, .T. ) ;
#21521=ORIENTED_EDGE ( 'NONE', *, *, #17996, .F. ) ;
#21522=EDGE_LOOP ( 'NONE', ( #29345, #25383, #22018, #6782 ) ) ;
#21524=ORIENTED_EDGE ( 'NONE', *, *, #26191, .F. ) ;
#21526=VERTEX_POINT ( 'NONE', #13321 ) ;
#21531=DIRECTION ( 'NONE',  ( 0.9510565162951536422, 2.566386769018988816E-16, 0.3090169943749472292 ) ) ;
#21532=EDGE_LOOP ( 'NONE', ( #2262, #28471, #15580, #12613 ) ) ;
#21533=CARTESIAN_POINT ( 'NONE',  ( 93.00224314937874226, -4.999999999999992006, 67.57008484791889202 ) ) ;
#21534=ORIENTED_EDGE ( 'NONE', *, *, #25697, .F. ) ;
#21538=LINE ( 'NONE', #28596, #27931 ) ;
#21540=EDGE_LOOP ( 'NONE', ( #12581, #29930, #16839, #8419 ) ) ;
#21541=LINE ( 'NONE', #17256, #18432 ) ;
#21543=CARTESIAN_POINT ( 'NONE',  ( 172.2287565553229172, -9.999999999999996447, -20.83012701892220520 ) ) ;
#21544=DIRECTION ( 'NONE',  ( -2.698458740408365879E-16, 1.000000000000000000, 0.000000000000000000 ) ) ;
#21546=FACE_OUTER_BOUND ( 'NONE', #27533, .T. ) ;
#21547=ORIENTED_EDGE ( 'NONE', *, *, #13011, .T. ) ;
#21551=ORIENTED_EDGE ( 'NONE', *, *, #7569, .T. ) ;
#21552=ADVANCED_FACE ( 'NONE', ( #22645 ), #13175, .T. ) ;
#21553=AXIS2_PLACEMENT_3D ( 'NONE', #8431, #3715, #3868 ) ;
#21557=CARTESIAN_POINT ( 'NONE',  ( 147.2287565553230309, -10.00000000000000178, -20.83012701892220520 ) ) ;
#21558=EDGE_CURVE ( 'NONE', #22270, #26851, #15459, .T. ) ;
#21559=PLANE ( 'NONE',  #26346 ) ;
#21563=ORIENTED_EDGE ( 'NONE', *, *, #11995, .F. ) ;
#21566=DIRECTION ( 'NONE',  ( 0.9510565162951536422, 0.000000000000000000, -0.3090169943749475623 ) ) ;
#21567=VECTOR ( 'NONE', #17065, 1000.000000000000000 ) ;
#21569=EDGE_LOOP ( 'NONE', ( #5380, #30110, #21260, #20627 ) ) ;
#21570=DIRECTION ( 'NONE',  ( 0.9510565162951535312, 2.566386769018988816E-16, -0.3090169943749475623 ) ) ;
#21574=ORIENTED_EDGE ( 'NONE', *, *, #14358, .T. ) ;
#21575=LINE ( 'NONE', #18568, #19615 ) ;
#21577=ORIENTED_EDGE ( 'NONE', *, *, #5468, .T. ) ;
#21578=DIRECTION ( 'NONE',  ( -0.9510565162951536422, -2.566386769018988816E-16, -0.3090169943749472292 ) ) ;
#21580=DIRECTION ( 'NONE',  ( -0.9510565162951536422, -2.566386769018988816E-16, -0.3090169943749472292 ) ) ;
#21581=EDGE_CURVE ( 'NONE', #11833, #14866, #24789, .T. ) ;
#21582=CARTESIAN_POINT ( 'NONE',  ( 107.7837191567167565, -4.999999999999987566, 78.30945579394082756 ) ) ;
#21584=LINE ( 'NONE', #543, #12401 ) ;
#21590=VERTEX_POINT ( 'NONE', #24632 ) ;
#21591=CARTESIAN_POINT ( 'NONE',  ( 130.7287565553228887, -4.999999999999982236, -10.89389676854976585 ) ) ;
#21594=ADVANCED_FACE ( 'NONE', ( #1744 ), #24485, .T. ) ;
#21595=DIRECTION ( 'NONE',  ( -2.698458740408365879E-16, 1.000000000000000000, 0.000000000000000000 ) ) ;
#21599=LINE ( 'NONE', #4966, #8562 ) ;
#21602=DIRECTION ( 'NONE',  ( 1.110223024625156540E-16, 2.995891024602366092E-32, 1.000000000000000000 ) ) ;
#21603=CARTESIAN_POINT ( 'NONE',  ( 171.1922820468853388, -9.999999999999996447, -22.25671179336496053 ) ) ;
#21604=AXIS2_PLACEMENT_3D ( 'NONE', #7909, #899, #17068 ) ;
#21607=EDGE_LOOP ( 'NONE', ( #11945, #15171, #30143, #3866, #4434 ) ) ;
#21611=AXIS2_PLACEMENT_3D ( 'NONE', #20217, #22371, #26983 ) ;
#21612=DIRECTION ( 'NONE',  ( -2.698458740408365879E-16, 1.000000000000000000, 0.000000000000000000 ) ) ;
#21613=ADVANCED_FACE ( 'NONE', ( #3729 ), #5366, .T. ) ;
#21615=ORIENTED_EDGE ( 'NONE', *, *, #23847, .T. ) ;
#21616=CARTESIAN_POINT ( 'NONE',  ( 159.5152310637605240, -1.999999999999972689, -30.37205893520531319 ) ) ;
#21617=DIRECTION ( 'NONE',  ( 0.9510565162951536422, 0.000000000000000000, -0.3090169943749475623 ) ) ;
#21620=AXIS2_PLACEMENT_3D ( 'NONE', #8363, #29941, #10804 ) ;
#21621=FACE_OUTER_BOUND ( 'NONE', #21894, .T. ) ;
#21622=LINE ( 'NONE', #17048, #15348 ) ;
#21624=CARTESIAN_POINT ( 'NONE',  ( 149.5152310637605240, -1.999999999999976685, -2.627941064794695691 ) ) ;
#21625=LINE ( 'NONE', #10168, #19757 ) ;
#21626=VERTEX_POINT ( 'NONE', #17254 ) ;
#21628=DIRECTION ( 'NONE',  ( -0.8090169943749474513, -2.183098979609982436E-16, -0.5877852522924731371 ) ) ;
#21629=EDGE_LOOP ( 'NONE', ( #23977, #4725, #21814, #7130, #626 ) ) ;
#21634=DIRECTION ( 'NONE',  ( 0.3090169943749475623, 8.338696094058001131E-17, 0.9510565162951536422 ) ) ;
#21636=DIRECTION ( 'NONE',  ( -2.698458740408365879E-16, 1.000000000000000000, 0.000000000000000000 ) ) ;
#21638=CARTESIAN_POINT ( 'NONE',  ( 132.2287565553230024, -1.999999999999981348, -12.16987298107780013 ) ) ;
#21642=EDGE_CURVE ( 'NONE', #7383, #22052, #24136, .T. ) ;
#21643=CARTESIAN_POINT ( 'NONE',  ( 129.5152310637605808, -1.999999999999982236, -2.627941064794695691 ) ) ;
#21644=DIRECTION ( 'NONE',  ( -2.698458740408365879E-16, 1.000000000000000000, 0.000000000000000000 ) ) ;
#21648=ORIENTED_EDGE ( 'NONE', *, *, #9838, .F. ) ;
#21653=DIRECTION ( 'NONE',  ( -0.5877852522924731371, -1.586114251531760235E-16, 0.8090169943749474513 ) ) ;
#21654=EDGE_LOOP ( 'NONE', ( #3482, #27817, #17745, #29709 ) ) ;
#21655=ORIENTED_EDGE ( 'NONE', *, *, #14443, .F. ) ;
#21661=ORIENTED_EDGE ( 'NONE', *, *, #10034, .T. ) ;
#21662=LINE ( 'NONE', #625, #10081 ) ;
#21663=ORIENTED_EDGE ( 'NONE', *, *, #8168, .T. ) ;
#21665=ORIENTED_EDGE ( 'NONE', *, *, #27011, .T. ) ;
#21669=VERTEX_POINT ( 'NONE', #14653 ) ;
#21670=CARTESIAN_POINT ( 'NONE',  ( 132.0152310637605524, -1.999999999999981348, -0.06116980274991495881 ) ) ;
#21671=ORIENTED_EDGE ( 'NONE', *, *, #11615, .F. ) ;
#21674=VERTEX_POINT ( 'NONE', #12223 ) ;
#21677=EDGE_LOOP ( 'NONE', ( #933, #27432, #25348, #19675 ) ) ;
#21678=DIRECTION ( 'NONE',  ( -2.698458740408365879E-16, 1.000000000000000000, 0.000000000000000000 ) ) ;
#21679=FACE_BOUND ( 'NONE', #2588, .T. ) ;
#21680=EDGE_CURVE ( 'NONE', #7265, #436, #2941, .T. ) ;
#21681=ADVANCED_FACE ( 'NONE', ( #19687 ), #24435, .T. ) ;
#21683=EDGE_CURVE ( 'NONE', #19068, #12130, #26435, .T. ) ;
#21684=ORIENTED_EDGE ( 'NONE', *, *, #29502, .T. ) ;
#21685=DIRECTION ( 'NONE',  ( -0.8090169943749474513, -2.183098979609982436E-16, -0.5877852522924731371 ) ) ;
#21686=DIRECTION ( 'NONE',  ( -0.8090169943749474513, -2.183098979609982436E-16, 0.5877852522924731371 ) ) ;
#21688=CARTESIAN_POINT ( 'NONE',  ( 176.1922820468853104, -9.999999999999994671, -22.25671179336496053 ) ) ;
#21690=PLANE ( 'NONE',  #27997 ) ;
#21691=VERTEX_POINT ( 'NONE', #10074 ) ;
#21692=CARTESIAN_POINT ( 'NONE',  ( 11.07703429628124958, -5.000000000000015099, 34.09160609439044975 ) ) ;
#21693=VERTEX_POINT ( 'NONE', #8087 ) ;
#21695=ORIENTED_EDGE ( 'NONE', *, *, #4499, .T. ) ;
#21697=LINE ( 'NONE', #23702, #1002 ) ;
#21699=CARTESIAN_POINT ( 'NONE',  ( 169.7287565553229456, -1.999999999999970024, -25.16025403784440329 ) ) ;
#21703=ORIENTED_EDGE ( 'NONE', *, *, #11376, .T. ) ;
#21706=VECTOR ( 'NONE', #20148, 1000.000000000000000 ) ;
#21709=EDGE_LOOP ( 'NONE', ( #22809, #10635, #16475, #22864 ) ) ;
#21710=DIRECTION ( 'NONE',  ( -0.5877852522924731371, 0.000000000000000000, 0.8090169943749474513 ) ) ;
#21714=LINE ( 'NONE', #26318, #6953 ) ;
#21715=ORIENTED_EDGE ( 'NONE', *, *, #4408, .T. ) ;
#21716=VECTOR ( 'NONE', #11820, 1000.000000000000000 ) ;
#21717=PLANE ( 'NONE',  #2078 ) ;
#21719=EDGE_LOOP ( 'NONE', ( #13672, #15508, #3511, #12391 ) ) ;
#21720=AXIS2_PLACEMENT_3D ( 'NONE', #21324, #10018, #587 ) ;
#21721=EDGE_CURVE ( 'NONE', #12612, #1753, #12365, .T. ) ;
#21722=EDGE_CURVE ( 'NONE', #117, #17394, #29050, .T. ) ;
#21723=CARTESIAN_POINT ( 'NONE',  ( 86.03433166160688472, -4.999999999999993783, 62.50760082067552048 ) ) ;
#21724=EDGE_CURVE ( 'NONE', #13408, #13174, #7801, .T. ) ;
#21725=CARTESIAN_POINT ( 'NONE',  ( 132.0152310637605524, -10.00000000000000711, -8.721423840594310306 ) ) ;
#21726=CARTESIAN_POINT ( 'NONE',  ( 159.5152310637604387, -10.00000000000000000, -4.391296821672111328 ) ) ;
#21727=VECTOR ( 'NONE', #4812, 1000.000000000000000 ) ;
#21728=LINE ( 'NONE', #10122, #25582 ) ;
#21729=VECTOR ( 'NONE', #14474, 1000.000000000000000 ) ;
#21734=ORIENTED_EDGE ( 'NONE', *, *, #3283, .F. ) ;
#21735=DIRECTION ( 'NONE',  ( 0.9510565162951535312, 2.566386769018988816E-16, -0.3090169943749475623 ) ) ;
#21736=AXIS2_PLACEMENT_3D ( 'NONE', #21725, #14544, #3136 ) ;
#21740=DIRECTION ( 'NONE',  ( -0.5877852522924731371, -1.586114251531760235E-16, 0.8090169943749474513 ) ) ;
#21742=DIRECTION ( 'NONE',  ( -2.698458740408365879E-16, 1.000000000000000000, 0.000000000000000000 ) ) ;
#21745=CARTESIAN_POINT ( 'NONE',  ( 171.1922820468852819, -9.999999999999996447, -2.083034168790677043 ) ) ;
#21747=PLANE ( 'NONE',  #12964 ) ;
#21748=DIRECTION ( 'NONE',  ( -2.698458740408365879E-16, 1.000000000000000000, 0.000000000000000000 ) ) ;
#21749=CIRCLE ( 'NONE', #16383, 5.999999999999977796 ) ;
#21752=EDGE_LOOP ( 'NONE', ( #2730, #22849, #13562, #9042 ) ) ;
#21754=EDGE_CURVE ( 'NONE', #1397, #12383, #21989, .T. ) ;
#21755=ORIENTED_EDGE ( 'NONE', *, *, #22840, .T. ) ;
#21758=AXIS2_PLACEMENT_3D ( 'NONE', #7821, #17129, #15121 ) ;
#21761=EDGE_LOOP ( 'NONE', ( #4442, #4972, #15248, #10085, #15122 ) ) ;
#21766=CARTESIAN_POINT ( 'NONE',  ( 94.33602617680786295, -4.999999999999992006, -68.53913494047789357 ) ) ;
#21769=CARTESIAN_POINT ( 'NONE',  ( 142.0152310637605808, -1.999999999999978018, -17.38167787843871182 ) ) ;
#21771=AXIS2_PLACEMENT_3D ( 'NONE', #14684, #9660, #7529 ) ;
#21774=VECTOR ( 'NONE', #2623, 1000.000000000000000 ) ;
#21776=VECTOR ( 'NONE', #4863, 1000.000000000000000 ) ;
#21777=DIRECTION ( 'NONE',  ( -0.8090169943749474513, -2.183098979609982436E-16, 0.5877852522924731371 ) ) ;
#21778=CARTESIAN_POINT ( 'NONE',  ( 154.5152310637604955, -4.999999999999975131, -2.627941064794695691 ) ) ;
#21780=LINE ( 'NONE', #19936, #15088 ) ;
#21781=CARTESIAN_POINT ( 'NONE',  ( 169.5152310637604103, -4.999999999999971578, -1.881997125516403749E-14 ) ) ;
#21783=PLANE ( 'NONE',  #25621 ) ;
#21784=CARTESIAN_POINT ( 'NONE',  ( 152.0152310637606092, -4.999999999999976019, -32.93883019725009120 ) ) ;
#21785=CARTESIAN_POINT ( 'NONE',  ( 131.1922820468854241, -10.00000000000000888, -28.06379628232387446 ) ) ;
#21786=ORIENTED_EDGE ( 'NONE', *, *, #16125, .F. ) ;
#21788=VERTEX_POINT ( 'NONE', #29521 ) ;
#21791=EDGE_CURVE ( 'NONE', #436, #6429, #1394, .T. ) ;
#21794=VECTOR ( 'NONE', #26152, 1000.000000000000000 ) ;
#21795=CARTESIAN_POINT ( 'NONE',  ( 166.1922820468853672, -4.999999999999973355, -22.25671179336496053 ) ) ;
#21796=DIRECTION ( 'NONE',  ( 0.3090169943749472292, 8.338696094057992503E-17, -0.9510565162951536422 ) ) ;
#21797=DIRECTION ( 'NONE',  ( -0.5877852522924731371, -1.586114251531760728E-16, -0.8090169943749474513 ) ) ;
#21799=ORIENTED_EDGE ( 'NONE', *, *, #7021, .F. ) ;
#21800=CARTESIAN_POINT ( 'NONE',  ( 147.0152310637606092, -10.00000000000000178, -24.27857615940569502 ) ) ;
#21801=ADVANCED_FACE ( 'NONE', ( #13277 ), #22596, .T. ) ;
#21802=LINE ( 'NONE', #12324, #5504 ) ;
#21803=CARTESIAN_POINT ( 'NONE',  ( 159.7287565553228887, -1.999999999999974021, 0.8205080756887930260 ) ) ;
#21804=ORIENTED_EDGE ( 'NONE', *, *, #6086, .F. ) ;
#21805=DIRECTION ( 'NONE',  ( -0.9510565162951536422, 0.000000000000000000, -0.3090169943749472292 ) ) ;
#21806=DIRECTION ( 'NONE',  ( 1.110223024625156540E-16, 2.995891024602366092E-32, 1.000000000000000000 ) ) ;
#21813=FACE_BOUND ( 'NONE', #26080, .T. ) ;
#21814=ORIENTED_EDGE ( 'NONE', *, *, #12933, .T. ) ;
#21818=DIRECTION ( 'NONE',  ( -0.5877852522924731371, -1.586114251531760728E-16, -0.8090169943749474513 ) ) ;
#21820=CARTESIAN_POINT ( 'NONE',  ( 176.1922820468853388, -1.999999999999968914, -30.91696583120936026 ) ) ;
#21821=ORIENTED_EDGE ( 'NONE', *, *, #25339, .T. ) ;
#21823=ADVANCED_FACE ( 'NONE', ( #8538 ), #22903, .T. ) ;
#21828=ADVANCED_FACE ( 'NONE', ( #27055 ), #20286, .T. ) ;
#21829=CARTESIAN_POINT ( 'NONE',  ( 159.7287565553229740, -1.999999999999972689, -25.16025403784440329 ) ) ;
#21831=ORIENTED_EDGE ( 'NONE', *, *, #8240, .T. ) ;
#21837=FACE_BOUND ( 'NONE', #6035, .T. ) ;
#21839=FACE_OUTER_BOUND ( 'NONE', #14974, .T. ) ;
#21840=LINE ( 'NONE', #9930, #17929 ) ;
#21841=LINE ( 'NONE', #28308, #3676 ) ;
#21843=CARTESIAN_POINT ( 'NONE',  ( 167.0152310637604955, -4.999999999999972466, -1.854241549900775782E-14 ) ) ;
#21847=ORIENTED_EDGE ( 'NONE', *, *, #680, .T. ) ;
#21848=AXIS2_PLACEMENT_3D ( 'NONE', #8673, #3657, #29349 ) ;
#21850=CARTESIAN_POINT ( 'NONE',  ( 159.7287565553229172, -1.999999999999973577, -7.839745962155603820 ) ) ;
#21851=DIRECTION ( 'NONE',  ( 0.5877852522924731371, 0.000000000000000000, 0.8090169943749474513 ) ) ;
#21853=CARTESIAN_POINT ( 'NONE',  ( 166.1922820468853104, -9.999999999999998224, -2.083034168790677043 ) ) ;
#21857=EDGE_CURVE ( 'NONE', #23142, #10211, #13122, .T. ) ;
#21858=VECTOR ( 'NONE', #28867, 1000.000000000000000 ) ;
#21861=ORIENTED_EDGE ( 'NONE', *, *, #6468, .T. ) ;
#21862=EDGE_CURVE ( 'NONE', #4141, #13418, #12975, .T. ) ;
#21863=CARTESIAN_POINT ( 'NONE',  ( 175.7287565553229456, -9.999999999999971578, 3.500000000000003109 ) ) ;
#21867=AXIS2_PLACEMENT_3D ( 'NONE', #6225, #29322, #1510 ) ;
#21868=LINE ( 'NONE', #22480, #344 ) ;
#21872=ORIENTED_EDGE ( 'NONE', *, *, #17787, .F. ) ;
#21873=CARTESIAN_POINT ( 'NONE',  ( 171.1922820468852819, -1.999999999999970912, -2.083034168790677043 ) ) ;
#21874=LINE ( 'NONE', #17293, #13791 ) ;
#21875=CARTESIAN_POINT ( 'NONE',  ( 164.5152310637604955, -4.999999999999973355, -30.37205893520531319 ) ) ;
#21876=VECTOR ( 'NONE', #22706, 1000.000000000000000 ) ;
#21877=CARTESIAN_POINT ( 'NONE',  ( 154.5152310637605808, -10.00000000000000000, -28.60870317832789667 ) ) ;
#21878=CARTESIAN_POINT ( 'NONE',  ( 169.7287565553228887, -1.999999999999970912, -7.839745962155603820 ) ) ;
#21879=ORIENTED_EDGE ( 'NONE', *, *, #1971, .F. ) ;
#21881=VECTOR ( 'NONE', #30123, 1000.000000000000000 ) ;
#21886=CLOSED_SHELL ( 'NONE', ( #13508, #28939, #7409, #28879, #26214, #28032, #23048, #9022, #14609, #21994, #6193, #7155, #8418, #21478, #22239, #5585, #14650, #3154, #27693, #11653, #7644, #28360, #18297, #15328, #16006, #28666, #29083, #19683, #1765, #7462, #12686, #8793, #29446, #28496, #25286, #8796, #15243, #15889, #26360, #4290, #14095, #29010, #14125, #17954, #22525, #20549, #12474, #10690, #9332, #19062, #6012, #25042, #11760, #19236, #27553, #4782, #5946, #14675, #15631, #4501, #2761, #21828, #17659, #29975, #30198, #16344, #6681, #13278, #21383, #19514, #25607, #5673, #1077, #9928, #29994, #576, #17371, #3610, #30162, #9125, #27523, #5925, #27397, #1134, #15126, #12960, #12593, #9927, #17038, #10941, #10177, #29471, #28103, #17407, #25738, #15752, #29004, #25911, #19102, #29833, #19684, #1718, #27770, #6984, #16204, #3107, #4571, #4569, #28528, #12412, #18486, #24935, #2858, #22791, #6190, #13283, #2148, #23418, #16055, #17109, #13928, #19644, #524, #22107, #13694, #4952, #607, #22281, #25010, #23994, #12971, #21613, #27433, #23995, #860, #4866, #14011, #2564, #19143, #13142, #26778, #17282, #1800, #30160, #15169, #13977, #346, #12176, #16866, #3898, #4232, #23560, #21681, #13822, #5566, #28557, #28699, #29042, #24873, #28187, #17712, #6230, #3199, #13726, #18242, #29754, #20547, #11859, #22498, #10694, #11715, #21801, #25663, #1626, #24356, #12030, #9584, #1342, #12104, #23770, #25798, #1171, #237, #8033, #8381, #13849, #18103, #29481, #27867, #25661, #13581, #23460, #17284, #10180, #8146, #17035, #24028, #25108, #24323, #24320, #3240, #13695, #25796, #8495, #21823, #16617, #4694, #21594, #27904, #27328, #606, #26434, #28494, #21006, #29325, #24483, #5161, #14341, #8724, #19103, #4441, #2758, #20964, #2940, #99, #19445, #3708, #934, #28585, #28091, #29363, #6912, #6859, #20780, #18725, #14745, #7330, #17318, #14815, #26243, #26395, #23286, #22710, #21512, #526, #19234, #11989, #25612, #22877, #5640, #9371, #18998, #1551, #29865, #28663, #9161, #25452, #1862, #1007, #3859, #21902, #3531, #27901, #10209, #16140, #7288, #29407, #30230, #4663, #195, #26967, #7059, #10267, #2720, #26823, #16306, #1844, #24660, #3823, #17110, #6570, #21552, #23803, #14992, #8655, #17824, #5642, #29208, #12375, #29789, #7940, #17547, #14713, #408, #6443, #6436, #24877, #2213, #8870, #24073, #20586, #5080, #25109, #2531, #10735, #20111, #27181, #28979, #12728, #27859, #15027, #862, #22131, #25288, #13387, #9996, #17399, #27168, #18796, #4610, #18861, #10729, #22843, #10173, #19100, #10272, #23010, #10901, #11409, #6268, #8414, #17957, #4772, #8455, #15514, #9543, #25722, #8241, #3318, #19137, #27184, #25251, #20846, #25700, #17509, #14741, #7153, #3316, #7285, #23735, #8659, #7981, #21197, #7080, #4472, #26260, #17995, #6092, #734, #13980, #8278, #18865, #615, #6367, #18898, #27095, #17956, #4405, #28693, #8109, #19549, #7661, #15515, #12248, #26394, #2141, #7238, #18301, #29791, #19347, #25578, #17679, #24566, #27805, #22135, #24916, #3280, #20409, #30120, #4365, #14654, #15371, #8658, #22668, #24620, #65, #9546, #22940, #20131, #12972, #14504, #10562, #15967, #1173, #10889, #8953, #20001, #22418, #1517, #25791, #20408, #3517, #12034, #26127, #6228, #23282, #1204, #13281, #16441, #30019, #2183, #9018, #17661, #14388, #16702, #18130, #7500, #11315, #11172, #24739, #2492, #29288, #11248, #17625, #4236, #24482, #17249, #13311, #14989, #22708, #16060, #22626, #10374, #1930, #6368, #9440, #7257, #4195, #5195, #23920, #29788, #7740, #27004, #29618, #5253, #25873, #5252, #20583, #19512, #4732 ) ) ;
#21888=DIRECTION ( 'NONE',  ( -2.698458740408365879E-16, 1.000000000000000000, 0.000000000000000000 ) ) ;
#21891=CARTESIAN_POINT ( 'NONE',  ( 138.6922820468854241, -10.00000000000000533, 2.247092850131519715 ) ) ;
#21892=CARTESIAN_POINT ( 'NONE',  ( 129.5152310637605808, -10.00000000000000888, -11.28819510263909187 ) ) ;
#21894=EDGE_LOOP ( 'NONE', ( #15425, #26694, #7955, #26380 ) ) ;
#21895=ORIENTED_EDGE ( 'NONE', *, *, #26018, .T. ) ;
#21900=EDGE_CURVE ( 'NONE', #15422, #29696, #29673, .T. ) ;
#21902=ADVANCED_FACE ( 'NONE', ( #17999 ), #25187, .T. ) ;
#21910=VECTOR ( 'NONE', #18114, 1000.000000000000000 ) ;
#21913=CARTESIAN_POINT ( 'NONE',  ( 16.08363025263714263, -5.000000000000013323, -49.50032404655522811 ) ) ;
#21914=ORIENTED_EDGE ( 'NONE', *, *, #11992, .T. ) ;
#21916=CARTESIAN_POINT ( 'NONE',  ( 130.7287565553229172, -4.999999999999983125, -19.55415080639416203 ) ) ;
#21917=DIRECTION ( 'NONE',  ( -2.698458740408365879E-16, 1.000000000000000000, 0.000000000000000000 ) ) ;
#21923=DIRECTION ( 'NONE',  ( -0.9510565162951536422, -2.566386769018988323E-16, 0.3090169943749475623 ) ) ;
#21924=CARTESIAN_POINT ( 'NONE',  ( 158.6922820468853672, -10.00000000000000000, -17.92658477444275889 ) ) ;
#21929=ORIENTED_EDGE ( 'NONE', *, *, #27009, .F. ) ;
#21930=CARTESIAN_POINT ( 'NONE',  ( 144.5152310637605808, -4.999999999999978684, -1.604441369360116507E-14 ) ) ;
#21931=DIRECTION ( 'NONE',  ( -0.9510565162951536422, -2.566386769018988323E-16, 0.3090169943749475623 ) ) ;
#21933=EDGE_CURVE ( 'NONE', #12771, #30193, #20140, .T. ) ;
#21934=CARTESIAN_POINT ( 'NONE',  ( 147.0152310637605524, -4.999999999999977796, -17.38167787843871182 ) ) ;
#21935=ORIENTED_EDGE ( 'NONE', *, *, #2042, .F. ) ;
#21937=VERTEX_POINT ( 'NONE', #2152 ) ;
#21938=EDGE_CURVE ( 'NONE', #619, #9664, #23051, .T. ) ;
#21942=VECTOR ( 'NONE', #8298, 1000.000000000000000 ) ;
#21944=CARTESIAN_POINT ( 'NONE',  ( 164.5152310637604671, -1.999999999999972244, -11.28819510263909542 ) ) ;
#21945=LINE ( 'NONE', #29157, #8216 ) ;
#21947=LINE ( 'NONE', #12928, #26465 ) ;
#21948=VECTOR ( 'NONE', #27937, 1000.000000000000000 ) ;
#21949=ORIENTED_EDGE ( 'NONE', *, *, #12144, .T. ) ;
#21950=DIRECTION ( 'NONE',  ( 0.5877852522924731371, 1.586114251531760728E-16, 0.8090169943749474513 ) ) ;
#21951=CARTESIAN_POINT ( 'NONE',  ( 168.6922820468853956, -1.999999999999970024, -32.39392330124607611 ) ) ;
#21952=PLANE ( 'NONE',  #30247 ) ;
#21953=ORIENTED_EDGE ( 'NONE', *, *, #19276, .T. ) ;
#21954=CARTESIAN_POINT ( 'NONE',  ( 134.7287565553230024, -1.999999999999980460, -16.50000000000000000 ) ) ;
#21956=AXIS2_PLACEMENT_3D ( 'NONE', #8933, #13232, #18104 ) ;
#21958=EDGE_CURVE ( 'NONE', #25168, #10075, #18753, .T. ) ;
#21961=VECTOR ( 'NONE', #27606, 1000.000000000000000 ) ;
#21965=FACE_BOUND ( 'NONE', #9818, .T. ) ;
#21966=EDGE_LOOP ( 'NONE', ( #641, #21929, #27106, #18652 ) ) ;
#21967=ORIENTED_EDGE ( 'NONE', *, *, #1373, .F. ) ;
#21968=ORIENTED_EDGE ( 'NONE', *, *, #4631, .T. ) ;
#21971=CARTESIAN_POINT ( 'NONE',  ( 111.5443916382889569, -4.999999999999986677, -81.04174428570250655 ) ) ;
#21973=LINE ( 'NONE', #3080, #13015 ) ;
#21974=EDGE_LOOP ( 'NONE', ( #22265, #16066, #1028, #17227, #21221 ) ) ;
#21975=EDGE_CURVE ( 'NONE', #21788, #2498, #7014, .T. ) ;
#21977=ORIENTED_EDGE ( 'NONE', *, *, #5599, .T. ) ;
#21981=VERTEX_POINT ( 'NONE', #6719 ) ;
#21983=VECTOR ( 'NONE', #19326, 1000.000000000000000 ) ;
#21985=ORIENTED_EDGE ( 'NONE', *, *, #13137, .T. ) ;
#21987=AXIS2_PLACEMENT_3D ( 'NONE', #216, #16533, #11641 ) ;
#21989=LINE ( 'NONE', #5817, #7123 ) ;
#21990=FACE_BOUND ( 'NONE', #7244, .T. ) ;
#21992=MANIFOLD_SOLID_BREP ( 'Fill Pattern1', #21886 ) ;
#21993=ORIENTED_EDGE ( 'NONE', *, *, #22492, .F. ) ;
#21994=ADVANCED_FACE ( 'NONE', ( #9128 ), #25623, .T. ) ;
#21995=DIRECTION ( 'NONE',  ( -0.8090169943749474513, -2.183098979609982436E-16, -0.5877852522924731371 ) ) ;
#21996=LINE ( 'NONE', #2790, #7213 ) ;
#21997=CARTESIAN_POINT ( 'NONE',  ( 161.1922820468853388, -1.999999999999973577, -10.74328820663507678 ) ) ;
#21999=CARTESIAN_POINT ( 'NONE',  ( 158.6922820468853672, -1.999999999999973577, -15.07341522555727664 ) ) ;
#22003=ORIENTED_EDGE ( 'NONE', *, *, #11861, .F. ) ;
#22004=LINE ( 'NONE', #5379, #10497 ) ;
#22005=ORIENTED_EDGE ( 'NONE', *, *, #11570, .T. ) ;
#22008=VERTEX_POINT ( 'NONE', #4573 ) ;
#22012=PLANE ( 'NONE',  #20479 ) ;
#22014=ORIENTED_EDGE ( 'NONE', *, *, #5600, .F. ) ;
#22018=ORIENTED_EDGE ( 'NONE', *, *, #25411, .F. ) ;
#22020=DIRECTION ( 'NONE',  ( -0.5877852522924731371, -1.586114251531760728E-16, -0.8090169943749474513 ) ) ;
#22022=DIRECTION ( 'NONE',  ( -0.5877852522924731371, -1.586114251531760728E-16, -0.8090169943749474513 ) ) ;
#22023=LINE ( 'NONE', #8124, #4491 ) ;
#22027=ORIENTED_EDGE ( 'NONE', *, *, #21002, .F. ) ;
#22028=EDGE_LOOP ( 'NONE', ( #27636, #25716, #11446, #28243 ) ) ;
#22030=LINE ( 'NONE', #20179, #4547 ) ;
#22031=EDGE_CURVE ( 'NONE', #5352, #16324, #27657, .T. ) ;
#22032=EDGE_CURVE ( 'NONE', #25023, #5352, #25481, .T. ) ;
#22033=CARTESIAN_POINT ( 'NONE',  ( 158.6922820468853104, -1.999999999999974909, -0.6060766987539614181 ) ) ;
#22036=CARTESIAN_POINT ( 'NONE',  ( 143.6922820468854525, -10.00000000000000355, -15.07341522555727664 ) ) ;
#22037=ORIENTED_EDGE ( 'NONE', *, *, #10994, .F. ) ;
#22041=ORIENTED_EDGE ( 'NONE', *, *, #21938, .F. ) ;
#22042=FACE_OUTER_BOUND ( 'NONE', #24012, .T. ) ;
#22043=DIRECTION ( 'NONE',  ( -0.5877852522924731371, -1.586114251531760235E-16, 0.8090169943749474513 ) ) ;
#22044=DIRECTION ( 'NONE',  ( -0.9510565162951536422, 0.000000000000000000, -0.3090169943749472292 ) ) ;
#22048=LINE ( 'NONE', #5573, #21013 ) ;
#22049=DIRECTION ( 'NONE',  ( 0.5877852522924731371, 1.586114251531760728E-16, 0.8090169943749474513 ) ) ;
#22051=VERTEX_POINT ( 'NONE', #16162 ) ;
#22052=VERTEX_POINT ( 'NONE', #25337 ) ;
#22055=DIRECTION ( 'NONE',  ( -0.8090169943749474513, -2.183098979609982436E-16, 0.5877852522924731371 ) ) ;
#22056=CARTESIAN_POINT ( 'NONE',  ( 143.6922820468854525, -10.00000000000000355, -26.58683881228715506 ) ) ;
#22058=CARTESIAN_POINT ( 'NONE',  ( 137.0152310637605808, -1.999999999999979572, -34.70218595412750773 ) ) ;
#22060=VERTEX_POINT ( 'NONE', #11874 ) ;
#22061=DIRECTION ( 'NONE',  ( 0.3090169943749472292, 8.338696094057992503E-17, -0.9510565162951536422 ) ) ;
#22063=VECTOR ( 'NONE', #8392, 1000.000000000000000 ) ;
#22065=ORIENTED_EDGE ( 'NONE', *, *, #6571, .T. ) ;
#22067=EDGE_LOOP ( 'NONE', ( #8247, #27775, #3486, #2614 ) ) ;
#22070=EDGE_CURVE ( 'NONE', #14866, #25730, #28259, .T. ) ;
#22071=ORIENTED_EDGE ( 'NONE', *, *, #18422, .F. ) ;
#22074=EDGE_CURVE ( 'NONE', #17531, #12785, #9428, .T. ) ;
#22075=CARTESIAN_POINT ( 'NONE',  ( 162.0152310637604387, -1.999999999999973133, -8.721423840594312082 ) ) ;
#22076=EDGE_CURVE ( 'NONE', #2523, #13085, #12026, .T. ) ;
#22081=LINE ( 'NONE', #17785, #1769 ) ;
#22083=FACE_OUTER_BOUND ( 'NONE', #13116, .T. ) ;
#22084=DIRECTION ( 'NONE',  ( -1.000000000000000000, -2.908569913943825554E-16, 0.000000000000000000 ) ) ;
#22085=VERTEX_POINT ( 'NONE', #13721 ) ;
#22086=DIRECTION ( 'NONE',  ( 0.9510565162951535312, 2.566386769018988816E-16, -0.3090169943749475623 ) ) ;
#22087=DIRECTION ( 'NONE',  ( -0.5877852522924731371, -1.586114251531760728E-16, -0.8090169943749474513 ) ) ;
#22090=VERTEX_POINT ( 'NONE', #20730 ) ;
#22091=ORIENTED_EDGE ( 'NONE', *, *, #12802, .F. ) ;
#22095=CARTESIAN_POINT ( 'NONE',  ( 144.5152310637606092, -4.999999999999978684, -28.60870317832789311 ) ) ;
#22097=DIRECTION ( 'NONE',  ( 0.000000000000000000, 0.000000000000000000, -1.000000000000000000 ) ) ;
#22098=VECTOR ( 'NONE', #25313, 1000.000000000000000 ) ;
#22101=CARTESIAN_POINT ( 'NONE',  ( 166.1922820468853672, -9.999999999999996447, -30.91696583120936026 ) ) ;
#22102=VERTEX_POINT ( 'NONE', #23184 ) ;
#22104=CARTESIAN_POINT ( 'NONE',  ( 137.2287565553230309, -4.999999999999980460, -12.16987298107779303 ) ) ;
#22105=PLANE ( 'NONE',  #9933 ) ;
#22106=AXIS2_PLACEMENT_3D ( 'NONE', #17475, #11062, #1321 ) ;
#22107=ADVANCED_FACE ( 'NONE', ( #20336 ), #25234, .T. ) ;
#22109=EDGE_CURVE ( 'NONE', #7751, #29440, #6318, .T. ) ;
#22112=ORIENTED_EDGE ( 'NONE', *, *, #16939, .T. ) ;
#22116=FACE_BOUND ( 'NONE', #13177, .T. ) ;
#22118=DIRECTION ( 'NONE',  ( 1.110223024625156540E-16, 2.995891024602366092E-32, 1.000000000000000000 ) ) ;
#22119=ORIENTED_EDGE ( 'NONE', *, *, #23958, .T. ) ;
#22121=CARTESIAN_POINT ( 'NONE',  ( 139.5152310637605524, -10.00000000000000533, -4.391296821672111328 ) ) ;
#22122=VERTEX_POINT ( 'NONE', #6465 ) ;
#22123=DIRECTION ( 'NONE',  ( -0.9510565162951536422, -2.566386769018988816E-16, -0.3090169943749472292 ) ) ;
#22124=ORIENTED_EDGE ( 'NONE', *, *, #27766, .F. ) ;
#22128=DIRECTION ( 'NONE',  ( -0.9510565162951536422, -2.566386769018988816E-16, -0.3090169943749472292 ) ) ;
#22129=VECTOR ( 'NONE', #5632, 1000.000000000000000 ) ;
#22131=ADVANCED_FACE ( 'NONE', ( #29877 ), #27559, .T. ) ;
#22135=ADVANCED_FACE ( 'NONE', ( #29422 ), #13766, .T. ) ;
#22136=EDGE_CURVE ( 'NONE', #26624, #20158, #8589, .T. ) ;
#22138=LINE ( 'NONE', #5819, #9884 ) ;
#22140=DIRECTION ( 'NONE',  ( -0.5877852522924731371, -1.586114251531760235E-16, 0.8090169943749474513 ) ) ;
#22141=LINE ( 'NONE', #24591, #2702 ) ;
#22142=VECTOR ( 'NONE', #23155, 1000.000000000000000 ) ;
#22144=DIRECTION ( 'NONE',  ( -2.698458740408365879E-16, 1.000000000000000000, 0.000000000000000000 ) ) ;
#22145=VERTEX_POINT ( 'NONE', #22949 ) ;
#22147=ORIENTED_EDGE ( 'NONE', *, *, #4948, .F. ) ;
#22149=ORIENTED_EDGE ( 'NONE', *, *, #4699, .F. ) ;
#22151=DIRECTION ( 'NONE',  ( 1.000000000000000000, 2.908569913943825554E-16, -6.938893903907227392E-16 ) ) ;
#22153=DIRECTION ( 'NONE',  ( -2.698458740408365879E-16, 1.000000000000000000, 0.000000000000000000 ) ) ;
#22156=VERTEX_POINT ( 'NONE', #17747 ) ;
#22159=ORIENTED_EDGE ( 'NONE', *, *, #23339, .F. ) ;
#22161=VERTEX_POINT ( 'NONE', #27105 ) ;
#22162=DIRECTION ( 'NONE',  ( -1.110223024625156540E-16, 0.000000000000000000, -1.000000000000000000 ) ) ;
#22170=VECTOR ( 'NONE', #21544, 1000.000000000000000 ) ;
#22171=ORIENTED_EDGE ( 'NONE', *, *, #11652, .F. ) ;
#22172=VERTEX_POINT ( 'NONE', #25384 ) ;
#22175=CARTESIAN_POINT ( 'NONE',  ( 139.5152310637605808, -1.999999999999978684, -21.71180489736090991 ) ) ;
#22176=FACE_OUTER_BOUND ( 'NONE', #25772, .T. ) ;
#22177=DIRECTION ( 'NONE',  ( -0.9510565162951536422, 0.000000000000000000, -0.3090169943749472292 ) ) ;
#22178=DIRECTION ( 'NONE',  ( -2.698458740408365879E-16, 1.000000000000000000, 0.000000000000000000 ) ) ;
#22184=CARTESIAN_POINT ( 'NONE',  ( 152.0152310637605524, -10.00000000000000000, -26.04193191628311155 ) ) ;
#22187=VECTOR ( 'NONE', #19069, 1000.000000000000000 ) ;
#22189=PLANE ( 'NONE',  #2944 ) ;
#22191=ORIENTED_EDGE ( 'NONE', *, *, #12111, .T. ) ;
#22192=CARTESIAN_POINT ( 'NONE',  ( 147.0152310637605808, -1.999999999999976241, -26.04193191628311155 ) ) ;
#22194=DIRECTION ( 'NONE',  ( -2.698458740408366372E-16, 1.000000000000000000, 0.000000000000000000 ) ) ;
#22196=ORIENTED_EDGE ( 'NONE', *, *, #8104, .F. ) ;
#22198=DIRECTION ( 'NONE',  ( 0.3090169943749475623, 8.338696094058001131E-17, 0.9510565162951536422 ) ) ;
#22200=ORIENTED_EDGE ( 'NONE', *, *, #11318, .F. ) ;
#22202=VECTOR ( 'NONE', #10780, 999.9999999999998863 ) ;
#22207=VECTOR ( 'NONE', #15695, 1000.000000000000000 ) ;
#22208=ORIENTED_EDGE ( 'NONE', *, *, #27967, .F. ) ;
#22210=VECTOR ( 'NONE', #28084, 1000.000000000000000 ) ;
#22211=VECTOR ( 'NONE', #1786, 1000.000000000000000 ) ;
#22212=CARTESIAN_POINT ( 'NONE',  ( 161.1922820468853956, -1.999999999999972689, -30.91696583120936026 ) ) ;
#22213=ORIENTED_EDGE ( 'NONE', *, *, #21137, .F. ) ;
#22214=LINE ( 'NONE', #7880, #25838 ) ;
#22215=DIRECTION ( 'NONE',  ( -2.698458740408365879E-16, 1.000000000000000000, 0.000000000000000000 ) ) ;
#22216=DIRECTION ( 'NONE',  ( -0.9510565162951536422, -2.566386769018988323E-16, 0.3090169943749475623 ) ) ;
#22217=DIRECTION ( 'NONE',  ( 0.9510565162951535312, 2.566386769018988816E-16, -0.3090169943749475623 ) ) ;
#22221=CARTESIAN_POINT ( 'NONE',  ( 95.85195911941896441, -4.999999999999991118, 69.64052469288915859 ) ) ;
#22225=CARTESIAN_POINT ( 'NONE',  ( 161.1922820468853104, -10.00000000000000000, -2.083034168790677043 ) ) ;
#22227=CARTESIAN_POINT ( 'NONE',  ( 152.0152310637605808, -4.999999999999976907, -34.70218595412750773 ) ) ;
#22228=LINE ( 'NONE', #15197, #11953 ) ;
#22230=EDGE_LOOP ( 'NONE', ( #21368, #17478, #964, #21524 ) ) ;
#22231=AXIS2_PLACEMENT_3D ( 'NONE', #6365, #11081, #8928 ) ;
#22232=DIRECTION ( 'NONE',  ( -2.698458740408365879E-16, 1.000000000000000000, -0.000000000000000000 ) ) ;
#22233=CARTESIAN_POINT ( 'NONE',  ( 144.5152310637605524, -1.999999999999978018, -2.627941064794695691 ) ) ;
#22237=EDGE_LOOP ( 'NONE', ( #17990, #15198, #17997, #21099, #10503 ) ) ;
#22239=ADVANCED_FACE ( 'NONE', ( #1602 ), #15758, .T. ) ;
#22240=EDGE_CURVE ( 'NONE', #15364, #26933, #25082, .T. ) ;
#22242=EDGE_CURVE ( 'NONE', #27200, #12000, #22794, .T. ) ;
#22244=DIRECTION ( 'NONE',  ( -2.698458740408365879E-16, 1.000000000000000000, 0.000000000000000000 ) ) ;
#22245=DIRECTION ( 'NONE',  ( -0.5877852522924731371, 0.000000000000000000, 0.8090169943749474513 ) ) ;
#22246=EDGE_CURVE ( 'NONE', #26241, #18105, #20490, .T. ) ;
#22247=FACE_OUTER_BOUND ( 'NONE', #9960, .T. ) ;
#22248=AXIS2_PLACEMENT_3D ( 'NONE', #97, #8785, #15806 ) ;
#22250=ORIENTED_EDGE ( 'NONE', *, *, #9367, .T. ) ;
#22251=LINE ( 'NONE', #17807, #1627 ) ;
#22252=CARTESIAN_POINT ( 'NONE',  ( 169.5152310637604103, -9.999999999999996447, -4.391296821672111328 ) ) ;
#22253=VECTOR ( 'NONE', #29886, 1000.000000000000000 ) ;
#22254=CARTESIAN_POINT ( 'NONE',  ( 146.1922820468853956, -10.00000000000000355, -4.936203717676158398 ) ) ;
#22258=VERTEX_POINT ( 'NONE', #27862 ) ;
#22260=ORIENTED_EDGE ( 'NONE', *, *, #29445, .T. ) ;
#22263=FACE_BOUND ( 'NONE', #10660, .T. ) ;
#22264=ORIENTED_EDGE ( 'NONE', *, *, #21169, .F. ) ;
#22265=ORIENTED_EDGE ( 'NONE', *, *, #21724, .T. ) ;
#22266=PLANE ( 'NONE',  #771 ) ;
#22270=VERTEX_POINT ( 'NONE', #16359 ) ;
#22271=ORIENTED_EDGE ( 'NONE', *, *, #29135, .T. ) ;
#22272=PLANE ( 'NONE',  #28157 ) ;
#22273=ORIENTED_EDGE ( 'NONE', *, *, #22462, .T. ) ;
#22279=EDGE_CURVE ( 'NONE', #6635, #18739, #25682, .T. ) ;
#22280=CARTESIAN_POINT ( 'NONE',  ( 149.7287565553229456, -1.999999999999976685, 0.8205080756887930260 ) ) ;
#22281=ADVANCED_FACE ( 'NONE', ( #356 ), #23694, .T. ) ;
#22282=VERTEX_POINT ( 'NONE', #4920 ) ;
#22284=DIRECTION ( 'NONE',  ( -2.698458740408365879E-16, 1.000000000000000000, 0.000000000000000000 ) ) ;
#22286=ORIENTED_EDGE ( 'NONE', *, *, #5974, .F. ) ;
#22288=FACE_BOUND ( 'NONE', #23381, .T. ) ;
#22291=ORIENTED_EDGE ( 'NONE', *, *, #4908, .F. ) ;
#22292=DIRECTION ( 'NONE',  ( 0.3090169943749475623, 8.338696094058001131E-17, 0.9510565162951536422 ) ) ;
#22294=DIRECTION ( 'NONE',  ( -2.698458740408365879E-16, 1.000000000000000000, 0.000000000000000000 ) ) ;
#22295=VECTOR ( 'NONE', #13194, 1000.000000000000000 ) ;
#22296=ORIENTED_EDGE ( 'NONE', *, *, #21134, .T. ) ;
#22297=VERTEX_POINT ( 'NONE', #30171 ) ;
#22298=LINE ( 'NONE', #3536, #21706 ) ;
#22300=ORIENTED_EDGE ( 'NONE', *, *, #16738, .F. ) ;
#22301=DIRECTION ( 'NONE',  ( 1.110223024625156540E-16, 2.995891024602366092E-32, 1.000000000000000000 ) ) ;
#22302=ORIENTED_EDGE ( 'NONE', *, *, #12374, .T. ) ;
#22304=ORIENTED_EDGE ( 'NONE', *, *, #155, .F. ) ;
#22306=CARTESIAN_POINT ( 'NONE',  ( 168.6922820468853672, -9.999999999999996447, -23.73366926340167637 ) ) ;
#22307=CARTESIAN_POINT ( 'NONE',  ( 111.9672181541861278, -4.999999999999986677, -81.34894573147012409 ) ) ;
#22309=LINE ( 'NONE', #7671, #2775 ) ;
#22310=ORIENTED_EDGE ( 'NONE', *, *, #27256, .F. ) ;
#22315=EDGE_CURVE ( 'NONE', #929, #18003, #28313, .T. ) ;
#22316=EDGE_LOOP ( 'NONE', ( #24066, #21872, #14323, #8207 ) ) ;
#22317=EDGE_CURVE ( 'NONE', #4321, #17684, #14214, .T. ) ;
#22318=VECTOR ( 'NONE', #19925, 1000.000000000000000 ) ;
#22321=EDGE_CURVE ( 'NONE', #27966, #21114, #20778, .T. ) ;
#22323=EDGE_CURVE ( 'NONE', #6890, #27640, #14513, .T. ) ;
#22328=VERTEX_POINT ( 'NONE', #16213 ) ;
#22330=AXIS2_PLACEMENT_3D ( 'NONE', #10384, #21686, #10079 ) ;
#22332=FACE_OUTER_BOUND ( 'NONE', #4051, .T. ) ;
#22333=LINE ( 'NONE', #4015, #12526 ) ;
#22341=ORIENTED_EDGE ( 'NONE', *, *, #25662, .F. ) ;
#22342=CARTESIAN_POINT ( 'NONE',  ( 133.6922820468854241, -10.00000000000000711, -35.24709285013155835 ) ) ;
#22344=DIRECTION ( 'NONE',  ( -2.698458740408365879E-16, 1.000000000000000000, 0.000000000000000000 ) ) ;
#22345=ORIENTED_EDGE ( 'NONE', *, *, #12895, .T. ) ;
#22347=DIRECTION ( 'NONE',  ( -0.8090169943749474513, -2.183098979609982436E-16, -0.5877852522924731371 ) ) ;
#22350=AXIS2_PLACEMENT_3D ( 'NONE', #18603, #23180, #4005 ) ;
#22352=CARTESIAN_POINT ( 'NONE',  ( 12.90791573655052282, -5.000000000000014211, 39.72647976162691918 ) ) ;
#22355=CARTESIAN_POINT ( 'NONE',  ( 144.7287565553230309, -10.00000000000000355, -25.16025403784439973 ) ) ;
#22356=CARTESIAN_POINT ( 'NONE',  ( 79.06642017383501297, -4.999999999999995559, 57.44511679343214894 ) ) ;
#22358=CARTESIAN_POINT ( 'NONE',  ( 172.2287565553229456, -9.999999999999994671, -29.49038105676660493 ) ) ;
#22360=EDGE_CURVE ( 'NONE', #7643, #18212, #2508, .T. ) ;
#22361=ORIENTED_EDGE ( 'NONE', *, *, #13179, .T. ) ;
#22363=LINE ( 'NONE', #3899, #22756 ) ;
#22368=VERTEX_POINT ( 'NONE', #2354 ) ;
#22371=DIRECTION ( 'NONE',  ( 1.000000000000000000, 2.698458740408365879E-16, -1.110223024625156540E-16 ) ) ;
#22372=VECTOR ( 'NONE', #22486, 1000.000000000000000 ) ;
#22373=ORIENTED_EDGE ( 'NONE', *, *, #28760, .F. ) ;
#22375=DIRECTION ( 'NONE',  ( -2.698458740408365879E-16, 1.000000000000000000, 0.000000000000000000 ) ) ;
#22377=LINE ( 'NONE', #24823, #29012 ) ;
#22378=DIRECTION ( 'NONE',  ( -1.110223024625156540E-16, 0.000000000000000000, -1.000000000000000000 ) ) ;
#22381=EDGE_CURVE ( 'NONE', #11253, #3713, #21095, .T. ) ;
#22383=DIRECTION ( 'NONE',  ( -0.9510565162951536422, -2.566386769018988816E-16, -0.3090169943749472292 ) ) ;
#22385=LINE ( 'NONE', #6506, #1044 ) ;
#22386=DIRECTION ( 'NONE',  ( 0.9510565162951536422, 0.000000000000000000, -0.3090169943749475623 ) ) ;
#22388=CARTESIAN_POINT ( 'NONE',  ( 167.0152310637604387, -1.999999999999971800, -8.721423840594312082 ) ) ;
#22389=ORIENTED_EDGE ( 'NONE', *, *, #18980, .T. ) ;
#22392=ORIENTED_EDGE ( 'NONE', *, *, #28365, .T. ) ;
#22393=VECTOR ( 'NONE', #7363, 1000.000000000000000 ) ;
#22395=CARTESIAN_POINT ( 'NONE',  ( 129.5152310637605524, -10.00000000000000888, -4.391296821672111328 ) ) ;
#22397=ORIENTED_EDGE ( 'NONE', *, *, #6601, .T. ) ;
#22399=ORIENTED_EDGE ( 'NONE', *, *, #27764, .T. ) ;
#22404=DIRECTION ( 'NONE',  ( -0.5877852522924731371, 0.000000000000000000, 0.8090169943749474513 ) ) ;
#22405=DIRECTION ( 'NONE',  ( 0.3090169943749475623, 8.338696094058001131E-17, 0.9510565162951536422 ) ) ;
#22406=LINE ( 'NONE', #13534, #5485 ) ;
#22407=ORIENTED_EDGE ( 'NONE', *, *, #8422, .T. ) ;
#22408=ORIENTED_EDGE ( 'NONE', *, *, #2384, .F. ) ;
#22410=AXIS2_PLACEMENT_3D ( 'NONE', #30098, #18276, #20419 ) ;
#22411=VECTOR ( 'NONE', #6609, 1000.000000000000000 ) ;
#22412=CARTESIAN_POINT ( 'NONE',  ( 167.0152310637604387, -4.999999999999971578, 1.702185954127501066 ) ) ;
#22418=ADVANCED_FACE ( 'NONE', ( #11626 ), #20786, .T. ) ;
#22420=VERTEX_POINT ( 'NONE', #5068 ) ;
#22422=EDGE_CURVE ( 'NONE', #9840, #16411, #7219, .T. ) ;
#22423=EDGE_LOOP ( 'NONE', ( #2362, #16290, #18278, #17095, #17806 ) ) ;
#22427=FACE_BOUND ( 'NONE', #2178, .T. ) ;
#22428=ORIENTED_EDGE ( 'NONE', *, *, #17211, .F. ) ;
#22429=VERTEX_POINT ( 'NONE', #18959 ) ;
#22430=DIRECTION ( 'NONE',  ( -0.8090169943749474513, -2.183098979609982436E-16, -0.5877852522924731371 ) ) ;
#22433=LINE ( 'NONE', #11126, #13957 ) ;
#22434=EDGE_LOOP ( 'NONE', ( #7143, #19524, #16994, #28673 ) ) ;
#22437=ORIENTED_EDGE ( 'NONE', *, *, #13818, .T. ) ;
#22438=AXIS2_PLACEMENT_3D ( 'NONE', #12690, #12241, #19407 ) ;
#22441=VECTOR ( 'NONE', #28191, 1000.000000000000000 ) ;
#22442=LINE ( 'NONE', #1999, #18916 ) ;
#22443=EDGE_LOOP ( 'NONE', ( #13124, #24859, #28811, #5389 ) ) ;
#22444=CARTESIAN_POINT ( 'NONE',  ( 6.306224973830111935, -5.000000000000015987, 19.40856478368036875 ) ) ;
#22446=ORIENTED_EDGE ( 'NONE', *, *, #1417, .T. ) ;
#22447=CARTESIAN_POINT ( 'NONE',  ( 159.7287565553228887, -10.00000000000000000, 0.8205080756887930260 ) ) ;
#22448=VECTOR ( 'NONE', #1149, 1000.000000000000000 ) ;
#22449=FACE_OUTER_BOUND ( 'NONE', #21654, .T. ) ;
#22450=AXIS2_PLACEMENT_3D ( 'NONE', #28774, #26451, #2806 ) ;
#22451=VERTEX_POINT ( 'NONE', #7373 ) ;
#22452=PLANE ( 'NONE',  #148 ) ;
#22453=EDGE_CURVE ( 'NONE', #563, #9294, #25991, .T. ) ;
#22455=VECTOR ( 'NONE', #20971, 1000.000000000000000 ) ;
#22456=LINE ( 'NONE', #5821, #12633 ) ;
#22457=ORIENTED_EDGE ( 'NONE', *, *, #10478, .T. ) ;
#22460=EDGE_CURVE ( 'NONE', #22503, #10636, #28920, .T. ) ;
#22461=PLANE ( 'NONE',  #25117 ) ;
#22462=EDGE_CURVE ( 'NONE', #26251, #4310, #5827, .T. ) ;
#22466=CARTESIAN_POINT ( 'NONE',  ( 164.5152310637604671, -9.999999999999998224, -11.28819510263909542 ) ) ;
#22468=CARTESIAN_POINT ( 'NONE',  ( 156.1922820468853388, -10.00000000000000178, -4.936203717676158398 ) ) ;
#22469=CARTESIAN_POINT ( 'NONE',  ( 133.6922820468854241, -4.999999999999981348, -23.73366926340167282 ) ) ;
#22470=ORIENTED_EDGE ( 'NONE', *, *, #3113, .T. ) ;
#22471=CARTESIAN_POINT ( 'NONE',  ( 147.2287565553230309, -4.999999999999977796, -29.49038105676659427 ) ) ;
#22472=ORIENTED_EDGE ( 'NONE', *, *, #11075, .F. ) ;
#22475=VECTOR ( 'NONE', #13231, 999.9999999999998863 ) ;
#22477=ORIENTED_EDGE ( 'NONE', *, *, #6746, .F. ) ;
#22478=LINE ( 'NONE', #18030, #28703 ) ;
#22479=CARTESIAN_POINT ( 'NONE',  ( 96.45015875629363222, -4.999999999999991118, -70.07514216931596707 ) ) ;
#22480=CARTESIAN_POINT ( 'NONE',  ( 130.7287565553229456, -4.999999999999983125, 0.5000000000000052180 ) ) ;
#22484=ORIENTED_EDGE ( 'NONE', *, *, #16733, .T. ) ;
#22486=DIRECTION ( 'NONE',  ( 0.9510565162951535312, 2.566386769018988816E-16, -0.3090169943749475623 ) ) ;
#22487=CARTESIAN_POINT ( 'NONE',  ( 153.6922820468854525, -1.999999999999974021, -32.39392330124607611 ) ) ;
#22488=VECTOR ( 'NONE', #21923, 999.9999999999998863 ) ;
#22491=AXIS2_PLACEMENT_3D ( 'NONE', #5118, #4666, #11827 ) ;
#22492=EDGE_CURVE ( 'NONE', #23715, #5737, #22004, .T. ) ;
#22493=EDGE_CURVE ( 'NONE', #18100, #24253, #17410, .T. ) ;
#22498=ADVANCED_FACE ( 'NONE', ( #19552 ), #5975, .T. ) ;
#22500=VERTEX_POINT ( 'NONE', #24009 ) ;
#22501=DIRECTION ( 'NONE',  ( 0.9510565162951536422, 0.000000000000000000, -0.3090169943749475623 ) ) ;
#22503=VERTEX_POINT ( 'NONE', #10390 ) ;
#22505=CARTESIAN_POINT ( 'NONE',  ( 159.5152310637604955, -1.999999999999973133, -21.71180489736091346 ) ) ;
#22507=LINE ( 'NONE', #1608, #29658 ) ;
#22509=ORIENTED_EDGE ( 'NONE', *, *, #1042, .F. ) ;
#22510=ORIENTED_EDGE ( 'NONE', *, *, #15932, .T. ) ;
#22511=DIRECTION ( 'NONE',  ( -2.698458740408365879E-16, 1.000000000000000000, 0.000000000000000000 ) ) ;
#22514=CARTESIAN_POINT ( 'NONE',  ( 167.2287565553229172, -1.999999999999971356, -12.16987298107780369 ) ) ;
#22518=VERTEX_POINT ( 'NONE', #12683 ) ;
#22521=EDGE_LOOP ( 'NONE', ( #285, #29267, #19657, #11841 ) ) ;
#22525=ADVANCED_FACE ( 'NONE', ( #15114 ), #24445, .T. ) ;
#22526=ORIENTED_EDGE ( 'NONE', *, *, #9235, .F. ) ;
#22528=DIRECTION ( 'NONE',  ( -2.698458740408365879E-16, 1.000000000000000000, 0.000000000000000000 ) ) ;
#22530=DIRECTION ( 'NONE',  ( -0.9510565162951536422, -2.566386769018988816E-16, -0.3090169943749472292 ) ) ;
#22531=CARTESIAN_POINT ( 'NONE',  ( 153.6922820468853388, -10.00000000000000178, -0.6060766987539614181 ) ) ;
#22532=EDGE_CURVE ( 'NONE', #19023, #20837, #795, .T. ) ;
#22533=CARTESIAN_POINT ( 'NONE',  ( 132.2287565553230024, -10.00000000000000888, -20.83012701892220164 ) ) ;
#22534=AXIS2_PLACEMENT_3D ( 'NONE', #21378, #7351, #25821 ) ;
#22535=CARTESIAN_POINT ( 'NONE',  ( 149.5152310637605524, -1.999999999999975797, -21.71180489736091346 ) ) ;
#22545=CARTESIAN_POINT ( 'NONE',  ( 158.6922820468853388, -4.999999999999975131, -9.266330736598359152 ) ) ;
#22546=ORIENTED_EDGE ( 'NONE', *, *, #3403, .F. ) ;
#22547=CARTESIAN_POINT ( 'NONE',  ( 131.1922820468854241, -1.999999999999981792, -10.74328820663507322 ) ) ;
#22550=LINE ( 'NONE', #8638, #13907 ) ;
#22551=LINE ( 'NONE', #8932, #1026 ) ;
#22552=AXIS2_PLACEMENT_3D ( 'NONE', #23533, #14655, #7209 ) ;
#22553=CARTESIAN_POINT ( 'NONE',  ( 164.7287565553228603, -4.999999999999972466, 0.8205080756888000204 ) ) ;
#22554=ORIENTED_EDGE ( 'NONE', *, *, #1376, .T. ) ;
#22555=ORIENTED_EDGE ( 'NONE', *, *, #20685, .F. ) ;
#22562=FACE_OUTER_BOUND ( 'NONE', #16995, .T. ) ;
#22564=CARTESIAN_POINT ( 'NONE',  ( 171.1922820468853672, -1.999999999999969580, -28.06379628232387802 ) ) ;
#22566=EDGE_CURVE ( 'NONE', #19566, #30087, #10086, .T. ) ;
#22567=ORIENTED_EDGE ( 'NONE', *, *, #20770, .T. ) ;
#22574=ORIENTED_EDGE ( 'NONE', *, *, #24912, .F. ) ;
#22575=VECTOR ( 'NONE', #2704, 1000.000000000000000 ) ;
#22578=DIRECTION ( 'NONE',  ( -0.7071067811865490160, -0.7071067811865460184, 0.000000000000000000 ) ) ;
#22579=ORIENTED_EDGE ( 'NONE', *, *, #29997, .F. ) ;
#22580=DIRECTION ( 'NONE',  ( 0.3090169943749475623, 8.338696094058001131E-17, 0.9510565162951536422 ) ) ;
#22582=DIRECTION ( 'NONE',  ( -2.698458740408365879E-16, 1.000000000000000000, 0.000000000000000000 ) ) ;
#22583=ORIENTED_EDGE ( 'NONE', *, *, #15891, .F. ) ;
#22590=DIRECTION ( 'NONE',  ( -0.9510565162951536422, -2.566386769018988323E-16, 0.3090169943749475623 ) ) ;
#22591=EDGE_CURVE ( 'NONE', #14514, #11139, #19399, .T. ) ;
#22594=VECTOR ( 'NONE', #20362, 1000.000000000000000 ) ;
#22595=ORIENTED_EDGE ( 'NONE', *, *, #2177, .F. ) ;
#22596=PLANE ( 'NONE',  #23700 ) ;
#22597=DIRECTION ( 'NONE',  ( 1.000000000000000000, 2.698458740408365879E-16, -1.110223024625156540E-16 ) ) ;
#22599=VERTEX_POINT ( 'NONE', #2955 ) ;
#22600=CARTESIAN_POINT ( 'NONE',  ( 174.5152310637603819, -9.999999999999994671, -4.391296821672111328 ) ) ;
#22601=VECTOR ( 'NONE', #12231, 1000.000000000000000 ) ;
#22602=CARTESIAN_POINT ( 'NONE',  ( 138.6922820468854525, -4.999999999999980460, -15.07341522555727309 ) ) ;
#22603=LINE ( 'NONE', #17846, #22899 ) ;
#22604=ORIENTED_EDGE ( 'NONE', *, *, #8492, .T. ) ;
#22605=VERTEX_POINT ( 'NONE', #29063 ) ;
#22606=DIRECTION ( 'NONE',  ( -0.8090169943749474513, -2.183098979609982436E-16, 0.5877852522924731371 ) ) ;
#22608=LINE ( 'NONE', #8701, #15572 ) ;
#22611=VECTOR ( 'NONE', #21806, 1000.000000000000000 ) ;
#22614=CARTESIAN_POINT ( 'NONE',  ( 163.6922820468853388, -1.999999999999972689, -17.92658477444275889 ) ) ;
#22615=EDGE_LOOP ( 'NONE', ( #28057, #3415, #28586, #10114, #21968 ) ) ;
#22616=FACE_OUTER_BOUND ( 'NONE', #4451, .T. ) ;
#22617=ORIENTED_EDGE ( 'NONE', *, *, #1277, .T. ) ;
#22621=VERTEX_POINT ( 'NONE', #12233 ) ;
#22622=ORIENTED_EDGE ( 'NONE', *, *, #19196, .T. ) ;
#22623=DIRECTION ( 'NONE',  ( -0.8090169943749474513, -2.183098979609982436E-16, -0.5877852522924731371 ) ) ;
#22625=DIRECTION ( 'NONE',  ( -0.9510565162951536422, -2.566386769018988323E-16, 0.3090169943749475623 ) ) ;
#22626=ADVANCED_FACE ( 'NONE', ( #652 ), #26445, .T. ) ;
#22628=EDGE_CURVE ( 'NONE', #13085, #17128, #4553, .T. ) ;
#22630=ORIENTED_EDGE ( 'NONE', *, *, #27696, .T. ) ;
#22631=EDGE_CURVE ( 'NONE', #28890, #12774, #18586, .T. ) ;
#22632=ORIENTED_EDGE ( 'NONE', *, *, #7240, .T. ) ;
#22638=CARTESIAN_POINT ( 'NONE',  ( 167.0152310637604671, -4.999999999999972466, -17.38167787843871182 ) ) ;
#22642=AXIS2_PLACEMENT_3D ( 'NONE', #3103, #24443, #29212 ) ;
#22645=FACE_OUTER_BOUND ( 'NONE', #20437, .T. ) ;
#22646=DIRECTION ( 'NONE',  ( -1.000000000000000000, 0.000000000000000000, 0.000000000000000000 ) ) ;
#22647=ORIENTED_EDGE ( 'NONE', *, *, #23954, .T. ) ;
#22649=LINE ( 'NONE', #7186, #7693 ) ;
#22650=LINE ( 'NONE', #8889, #21942 ) ;
#22651=CARTESIAN_POINT ( 'NONE',  ( 169.5152310637604955, -9.999999999999994671, -30.37205893520531319 ) ) ;
#22653=ORIENTED_EDGE ( 'NONE', *, *, #13757, .F. ) ;
#22655=FACE_OUTER_BOUND ( 'NONE', #3363, .T. ) ;
#22661=PLANE ( 'NONE',  #9606 ) ;
#22663=EDGE_LOOP ( 'NONE', ( #3689, #2013, #18015, #28174, #25968 ) ) ;
#22664=DIRECTION ( 'NONE',  ( 0.9510565162951535312, 2.566386769018988816E-16, -0.3090169943749475623 ) ) ;
#22665=VERTEX_POINT ( 'NONE', #13841 ) ;
#22668=ADVANCED_FACE ( 'NONE', ( #16286 ), #4409, .T. ) ;
#22669=EDGE_CURVE ( 'NONE', #22621, #10540, #11549, .T. ) ;
#22670=EDGE_CURVE ( 'NONE', #19094, #20748, #20569, .T. ) ;
#22671=EDGE_CURVE ( 'NONE', #26944, #24422, #20864, .T. ) ;
#22672=ORIENTED_EDGE ( 'NONE', *, *, #6263, .F. ) ;
#22674=PLANE ( 'NONE',  #22106 ) ;
#22675=VERTEX_POINT ( 'NONE', #23316 ) ;
#22676=ORIENTED_EDGE ( 'NONE', *, *, #8799, .T. ) ;
#22679=CARTESIAN_POINT ( 'NONE',  ( 176.1922820468852819, -9.999999999999994671, -13.59645775552055902 ) ) ;
#22680=VECTOR ( 'NONE', #26910, 1000.000000000000000 ) ;
#22681=LINE ( 'NONE', #6500, #9677 ) ;
#22685=CARTESIAN_POINT ( 'NONE',  ( 83.18461569156667679, -4.999999999999994671, 60.43716097570526102 ) ) ;
#22687=DIRECTION ( 'NONE',  ( 0.9510565162951536422, 0.000000000000000000, -0.3090169943749475623 ) ) ;
#22688=CARTESIAN_POINT ( 'NONE',  ( 142.0152310637606092, -1.999999999999978018, -15.61832212156129707 ) ) ;
#22690=DIRECTION ( 'NONE',  ( 1.000000000000000000, 2.698458740408365879E-16, -1.110223024625156540E-16 ) ) ;
#22694=VERTEX_POINT ( 'NONE', #27789 ) ;
#22695=DIRECTION ( 'NONE',  ( 0.9510565162951535312, 2.566386769018988816E-16, -0.3090169943749475623 ) ) ;
#22696=FACE_OUTER_BOUND ( 'NONE', #10001, .T. ) ;
#22697=ORIENTED_EDGE ( 'NONE', *, *, #13691, .T. ) ;
#22699=VERTEX_POINT ( 'NONE', #17709 ) ;
#22703=AXIS2_PLACEMENT_3D ( 'NONE', #9937, #5526, #19249 ) ;
#22704=EDGE_CURVE ( 'NONE', #12785, #13256, #8961, .T. ) ;
#22706=DIRECTION ( 'NONE',  ( 1.000000000000000000, 2.698458740408365879E-16, -1.779203565104417375E-16 ) ) ;
#22707=AXIS2_PLACEMENT_3D ( 'NONE', #26838, #28721, #21056 ) ;
#22708=ADVANCED_FACE ( 'NONE', ( #23031 ), #9258, .T. ) ;
#22710=ADVANCED_FACE ( 'NONE', ( #6997 ), #18277, .T. ) ;
#22712=ORIENTED_EDGE ( 'NONE', *, *, #18596, .F. ) ;
#22713=CARTESIAN_POINT ( 'NONE',  ( 18.70776367089402825, -5.000000000000012434, -57.57657626727587541 ) ) ;
#22714=AXIS2_PLACEMENT_3D ( 'NONE', #3922, #13219, #17196 ) ;
#22716=ORIENTED_EDGE ( 'NONE', *, *, #3135, .T. ) ;
#22718=CARTESIAN_POINT ( 'NONE',  ( 93.42506966527585632, -4.999999999999992006, 67.87728629368646693 ) ) ;
#22719=VECTOR ( 'NONE', #29146, 1000.000000000000000 ) ;
#22725=VECTOR ( 'NONE', #784, 1000.000000000000000 ) ;
#22727=CARTESIAN_POINT ( 'NONE',  ( 139.7287565553230309, -4.999999999999980460, -16.49999999999999289 ) ) ;
#22729=FACE_BOUND ( 'NONE', #24303, .T. ) ;
#22730=ORIENTED_EDGE ( 'NONE', *, *, #15163, .T. ) ;
#22731=CARTESIAN_POINT ( 'NONE',  ( 149.5152310637605240, -4.999999999999976907, -1.659952520591373703E-14 ) ) ;
#22732=DIRECTION ( 'NONE',  ( 0.000000000000000000, 0.000000000000000000, 1.000000000000000000 ) ) ;
#22740=VECTOR ( 'NONE', #2100, 1000.000000000000000 ) ;
#22742=DIRECTION ( 'NONE',  ( -2.698458740408365879E-16, 1.000000000000000000, 0.000000000000000000 ) ) ;
#22743=EDGE_CURVE ( 'NONE', #28787, #5689, #20711, .T. ) ;
#22744=VECTOR ( 'NONE', #22958, 1000.000000000000000 ) ;
#22748=LINE ( 'NONE', #11425, #6459 ) ;
#22749=ORIENTED_EDGE ( 'NONE', *, *, #23845, .T. ) ;
#22750=LINE ( 'NONE', #15861, #1470 ) ;
#22752=DIRECTION ( 'NONE',  ( -0.9510565162951536422, -2.566386769018988323E-16, 0.3090169943749475623 ) ) ;
#22753=ORIENTED_EDGE ( 'NONE', *, *, #8980, .F. ) ;
#22754=EDGE_LOOP ( 'NONE', ( #24618, #2158, #10931, #20927 ) ) ;
#22755=DIRECTION ( 'NONE',  ( 0.9510565162951535312, 2.566386769018988816E-16, -0.3090169943749475623 ) ) ;
#22756=VECTOR ( 'NONE', #22664, 1000.000000000000000 ) ;
#22760=EDGE_CURVE ( 'NONE', #11002, #29409, #21024, .T. ) ;
#22761=VERTEX_POINT ( 'NONE', #6851 ) ;
#22762=ORIENTED_EDGE ( 'NONE', *, *, #30163, .F. ) ;
#22764=CARTESIAN_POINT ( 'NONE',  ( 143.6922820468853956, -4.999999999999979572, -0.6060766987539614181 ) ) ;
#22766=AXIS2_PLACEMENT_3D ( 'NONE', #1111, #3104, #12833 ) ;
#22768=LINE ( 'NONE', #17415, #23452 ) ;
#22769=CARTESIAN_POINT ( 'NONE',  ( 157.2287565553229456, -10.00000000000000000, -12.16987298107780369 ) ) ;
#22770=VERTEX_POINT ( 'NONE', #16145 ) ;
#22772=ORIENTED_EDGE ( 'NONE', *, *, #16902, .F. ) ;
#22777=ORIENTED_EDGE ( 'NONE', *, *, #11476, .T. ) ;
#22778=CARTESIAN_POINT ( 'NONE',  ( 162.0152310637605524, -9.999999999999998224, -32.93883019725009120 ) ) ;
#22779=CARTESIAN_POINT ( 'NONE',  ( 167.2287565553229172, -9.999999999999998224, -12.16987298107780369 ) ) ;
#22783=ORIENTED_EDGE ( 'NONE', *, *, #18205, .T. ) ;
#22786=FACE_OUTER_BOUND ( 'NONE', #4415, .T. ) ;
#22788=LINE ( 'NONE', #11772, #1704 ) ;
#22790=DIRECTION ( 'NONE',  ( -1.110223024625156540E-16, 0.000000000000000000, -1.000000000000000000 ) ) ;
#22791=ADVANCED_FACE ( 'NONE', ( #25461 ), #2430, .T. ) ;
#22792=EDGE_CURVE ( 'NONE', #23986, #7041, #6125, .T. ) ;
#22794=LINE ( 'NONE', #1902, #23727 ) ;
#22795=ORIENTED_EDGE ( 'NONE', *, *, #22381, .T. ) ;
#22797=EDGE_CURVE ( 'NONE', #17495, #29391, #9413, .T. ) ;
#22798=VECTOR ( 'NONE', #19371, 1000.000000000000000 ) ;
#22799=LINE ( 'NONE', #27977, #4304 ) ;
#22801=LINE ( 'NONE', #27419, #28333 ) ;
#22809=ORIENTED_EDGE ( 'NONE', *, *, #11652, .T. ) ;
#22812=FACE_OUTER_BOUND ( 'NONE', #20275, .T. ) ;
#22814=FACE_OUTER_BOUND ( 'NONE', #24432, .T. ) ;
#22817=LINE ( 'NONE', #20804, #1815 ) ;
#22822=ORIENTED_EDGE ( 'NONE', *, *, #12331, .T. ) ;
#22824=DIRECTION ( 'NONE',  ( 1.110223024625156540E-16, 2.995891024602366092E-32, 1.000000000000000000 ) ) ;
#22825=VECTOR ( 'NONE', #13654, 1000.000000000000000 ) ;
#22826=LINE ( 'NONE', #18380, #25038 ) ;
#22827=EDGE_LOOP ( 'NONE', ( #21695, #16358, #25282, #30170 ) ) ;
#22828=DIRECTION ( 'NONE',  ( -0.9510565162951536422, 0.000000000000000000, -0.3090169943749472292 ) ) ;
#22830=DIRECTION ( 'NONE',  ( -2.698458740408365879E-16, 1.000000000000000000, 0.000000000000000000 ) ) ;
#22831=CARTESIAN_POINT ( 'NONE',  ( 167.2287565553229456, -9.999999999999998224, -20.83012701892220520 ) ) ;
#22837=ORIENTED_EDGE ( 'NONE', *, *, #6479, .T. ) ;
#22840=EDGE_CURVE ( 'NONE', #12109, #4141, #21625, .T. ) ;
#22841=DIRECTION ( 'NONE',  ( -0.9510565162951536422, -2.566386769018988816E-16, -0.3090169943749472292 ) ) ;
#22842=PLANE ( 'NONE',  #10489 ) ;
#22843=ADVANCED_FACE ( 'NONE', ( #19183 ), #21170, .T. ) ;
#22845=LINE ( 'NONE', #4072, #23411 ) ;
#22847=CARTESIAN_POINT ( 'NONE',  ( 80.33489972152645464, -4.999999999999995559, 58.36672113073498736 ) ) ;
#22849=ORIENTED_EDGE ( 'NONE', *, *, #24493, .F. ) ;
#22850=DIRECTION ( 'NONE',  ( -2.698458740408365879E-16, 1.000000000000000000, 0.000000000000000000 ) ) ;
#22852=CARTESIAN_POINT ( 'NONE',  ( 175.7287565553229456, -9.999999999999994671, -30.76635726929469783 ) ) ;
#22853=ORIENTED_EDGE ( 'NONE', *, *, #13280, .T. ) ;
#22856=AXIS2_PLACEMENT_3D ( 'NONE', #596, #21634, #12925 ) ;
#22859=CARTESIAN_POINT ( 'NONE',  ( 137.0152310637605808, -4.999999999999980460, -34.70218595412750773 ) ) ;
#22862=ORIENTED_EDGE ( 'NONE', *, *, #1075, .T. ) ;
#22863=FACE_OUTER_BOUND ( 'NONE', #22434, .T. ) ;
#22864=ORIENTED_EDGE ( 'NONE', *, *, #26709, .F. ) ;
#22865=CARTESIAN_POINT ( 'NONE',  ( 153.6922820468854525, -10.00000000000000000, -32.39392330124607611 ) ) ;
#22866=PLANE ( 'NONE',  #21620 ) ;
#22867=LINE ( 'NONE', #15979, #26324 ) ;
#22869=VECTOR ( 'NONE', #17880, 999.9999999999998863 ) ;
#22870=ORIENTED_EDGE ( 'NONE', *, *, #17039, .F. ) ;
#22872=ORIENTED_EDGE ( 'NONE', *, *, #13962, .F. ) ;
#22873=EDGE_CURVE ( 'NONE', #14794, #23543, #429, .T. ) ;
#22874=EDGE_CURVE ( 'NONE', #22770, #11670, #12007, .T. ) ;
#22876=DIRECTION ( 'NONE',  ( 0.5877852522924731371, 0.000000000000000000, 0.8090169943749474513 ) ) ;
#22877=ADVANCED_FACE ( 'NONE', ( #2722 ), #14739, .T. ) ;
#22879=DIRECTION ( 'NONE',  ( 1.000000000000000000, 2.698458740408365879E-16, -1.110223024625156540E-16 ) ) ;
#22881=EDGE_CURVE ( 'NONE', #29503, #10414, #18883, .T. ) ;
#22884=EDGE_LOOP ( 'NONE', ( #12766, #11298, #8183, #29064 ) ) ;
#22885=CARTESIAN_POINT ( 'NONE',  ( 162.2287565553229172, -4.999999999999974243, -12.16987298107780013 ) ) ;
#22887=DIRECTION ( 'NONE',  ( 0.3090169943749475623, 8.338696094058001131E-17, 0.9510565162951536422 ) ) ;
#22888=ORIENTED_EDGE ( 'NONE', *, *, #10771, .F. ) ;
#22889=ORIENTED_EDGE ( 'NONE', *, *, #23593, .F. ) ;
#22890=DIRECTION ( 'NONE',  ( -2.698458740408365879E-16, 1.000000000000000000, 0.000000000000000000 ) ) ;
#22891=VERTEX_POINT ( 'NONE', #12455 ) ;
#22897=LINE ( 'NONE', #27362, #28718 ) ;
#22898=CARTESIAN_POINT ( 'NONE',  ( 6.941579719855231367, -5.000000000000015987, 21.36398562578804317 ) ) ;
#22899=VECTOR ( 'NONE', #22752, 999.9999999999998863 ) ;
#22901=ORIENTED_EDGE ( 'NONE', *, *, #20651, .F. ) ;
#22903=PLANE ( 'NONE',  #30118 ) ;
#22904=CARTESIAN_POINT ( 'NONE',  ( 174.5152310637604103, -9.999999999999994671, -2.627941064794695691 ) ) ;
#22908=CARTESIAN_POINT ( 'NONE',  ( 129.5152310637605808, -10.00000000000000888, -11.28819510263909187 ) ) ;
#22909=ORIENTED_EDGE ( 'NONE', *, *, #8956, .T. ) ;
#22910=ORIENTED_EDGE ( 'NONE', *, *, #20169, .T. ) ;
#22911=EDGE_CURVE ( 'NONE', #20344, #19263, #16751, .T. ) ;
#22912=LINE ( 'NONE', #30131, #28069 ) ;
#22917=VECTOR ( 'NONE', #25787, 1000.000000000000000 ) ;
#22918=ORIENTED_EDGE ( 'NONE', *, *, #16833, .T. ) ;
#22920=VECTOR ( 'NONE', #21092, 999.9999999999998863 ) ;
#22922=DIRECTION ( 'NONE',  ( -0.8090169943749474513, -2.183098979609982436E-16, -0.5877852522924731371 ) ) ;
#22923=DIRECTION ( 'NONE',  ( 1.000000000000000000, 0.000000000000000000, 0.000000000000000000 ) ) ;
#22924=VECTOR ( 'NONE', #12979, 1000.000000000000000 ) ;
#22925=ORIENTED_EDGE ( 'NONE', *, *, #22422, .F. ) ;
#22927=ORIENTED_EDGE ( 'NONE', *, *, #18210, .T. ) ;
#22931=ORIENTED_EDGE ( 'NONE', *, *, #27554, .T. ) ;
#22932=CARTESIAN_POINT ( 'NONE',  ( 152.2287565553229456, -1.999999999999975797, -3.509618943233403510 ) ) ;
#22933=CARTESIAN_POINT ( 'NONE',  ( 8.295003646061877234, -5.000000000000015099, 25.52939616229333097 ) ) ;
#22934=VECTOR ( 'NONE', #1449, 1000.000000000000000 ) ;
#22939=ORIENTED_EDGE ( 'NONE', *, *, #21161, .F. ) ;
#22940=ADVANCED_FACE ( 'NONE', ( #10015 ), #16596, .T. ) ;
#22941=LINE ( 'NONE', #23226, #12290 ) ;
#22943=DIRECTION ( 'NONE',  ( 1.000000000000000000, 2.698458740408365879E-16, -1.110223024625156540E-16 ) ) ;
#22949=CARTESIAN_POINT ( 'NONE',  ( 133.7287565553229172, -9.999999999999991118, -41.50000000000000000 ) ) ;
#22951=AXIS2_PLACEMENT_3D ( 'NONE', #25504, #11594, #4594 ) ;
#22954=CARTESIAN_POINT ( 'NONE',  ( 153.6922820468854241, -10.00000000000000000, -26.58683881228715862 ) ) ;
#22955=FACE_OUTER_BOUND ( 'NONE', #8111, .T. ) ;
#22957=ORIENTED_EDGE ( 'NONE', *, *, #18656, .T. ) ;
#22958=DIRECTION ( 'NONE',  ( -1.110223024625156540E-16, 0.000000000000000000, -1.000000000000000000 ) ) ;
#22963=VERTEX_POINT ( 'NONE', #9713 ) ;
#22965=DIRECTION ( 'NONE',  ( 0.5877852522924731371, 1.586114251531760728E-16, -0.8090169943749474513 ) ) ;
#22967=EDGE_LOOP ( 'NONE', ( #13884, #10456, #28648, #8514 ) ) ;
#22968=DIRECTION ( 'NONE',  ( -0.9510565162951536422, 0.000000000000000000, -0.3090169943749472292 ) ) ;
#22972=EDGE_LOOP ( 'NONE', ( #1861, #3814, #10320, #6150, #8722 ) ) ;
#22974=EDGE_CURVE ( 'NONE', #10414, #2375, #2582, .T. ) ;
#22976=VECTOR ( 'NONE', #1953, 1000.000000000000000 ) ;
#22978=CARTESIAN_POINT ( 'NONE',  ( 152.2287565553229740, -10.00000000000000178, -12.16987298107780369 ) ) ;
#22981=CARTESIAN_POINT ( 'NONE',  ( 158.6922820468854241, -9.999999999999998224, -35.24709285013155835 ) ) ;
#22982=CARTESIAN_POINT ( 'NONE',  ( 9.328867290168380677, -5.000000000000015099, 28.71130127944392640 ) ) ;
#22986=ORIENTED_EDGE ( 'NONE', *, *, #20743, .F. ) ;
#22989=CARTESIAN_POINT ( 'NONE',  ( 148.6922820468853672, -10.00000000000000355, -0.6060766987539614181 ) ) ;
#22994=ORIENTED_EDGE ( 'NONE', *, *, #8360, .F. ) ;
#22995=CARTESIAN_POINT ( 'NONE',  ( 12.58353042223624918, -5.000000000000014211, -38.72812442006048883 ) ) ;
#22997=ORIENTED_EDGE ( 'NONE', *, *, #23729, .T. ) ;
#22999=CARTESIAN_POINT ( 'NONE',  ( 163.6922820468852819, -1.999999999999973577, -0.6060766987539614181 ) ) ;
#23000=CARTESIAN_POINT ( 'NONE',  ( 14.49818551070089967, -5.000000000000013323, 44.62082686519693908 ) ) ;
#23002=VERTEX_POINT ( 'NONE', #25764 ) ;
#23003=ORIENTED_EDGE ( 'NONE', *, *, #3036, .F. ) ;
#23008=DIRECTION ( 'NONE',  ( -0.8090169943749474513, -2.183098979609982436E-16, 0.5877852522924731371 ) ) ;
#23010=ADVANCED_FACE ( 'NONE', ( #26378 ), #23940, .T. ) ;
#23012=VECTOR ( 'NONE', #187, 1000.000000000000000 ) ;
#23014=EDGE_CURVE ( 'NONE', #26487, #15051, #12309, .T. ) ;
#23015=CARTESIAN_POINT ( 'NONE',  ( 132.0152310637605524, -10.00000000000000711, -0.06116980274991495881 ) ) ;
#23016=AXIS2_PLACEMENT_3D ( 'NONE', #6323, #13624, #18204 ) ;
#23017=VERTEX_POINT ( 'NONE', #29469 ) ;
#23018=ORIENTED_EDGE ( 'NONE', *, *, #13248, .F. ) ;
#23019=PLANE ( 'NONE',  #3159 ) ;
#23020=CARTESIAN_POINT ( 'NONE',  ( 174.7287565553229456, -1.999999999999968470, -33.82050807568879947 ) ) ;
#23021=ORIENTED_EDGE ( 'NONE', *, *, #485, .T. ) ;
#23026=VECTOR ( 'NONE', #12556, 1000.000000000000000 ) ;
#23028=CARTESIAN_POINT ( 'NONE',  ( 151.1922820468854241, -1.999999999999975797, -22.25671179336496053 ) ) ;
#23030=LINE ( 'NONE', #24872, #26818 ) ;
#23031=FACE_OUTER_BOUND ( 'NONE', #12530, .T. ) ;
#23032=ORIENTED_EDGE ( 'NONE', *, *, #13945, .T. ) ;
#23033=LINE ( 'NONE', #2135, #3227 ) ;
#23035=ORIENTED_EDGE ( 'NONE', *, *, #23085, .F. ) ;
#23036=DIRECTION ( 'NONE',  ( 0.3090169943749475623, 8.338696094058001131E-17, 0.9510565162951536422 ) ) ;
#23037=VERTEX_POINT ( 'NONE', #29306 ) ;
#23042=ORIENTED_EDGE ( 'NONE', *, *, #6879, .F. ) ;
#23044=DIRECTION ( 'NONE',  ( -0.8090169943749474513, -2.183098979609982436E-16, 0.5877852522924731371 ) ) ;
#23045=CARTESIAN_POINT ( 'NONE',  ( 138.6922820468854525, -1.999999999999979128, -6.413161187712876909 ) ) ;
#23048=ADVANCED_FACE ( 'NONE', ( #10467 ), #5609, .T. ) ;
#23049=EDGE_CURVE ( 'NONE', #22599, #19874, #26686, .T. ) ;
#23050=EDGE_CURVE ( 'NONE', #20351, #26883, #10628, .T. ) ;
#23051=LINE ( 'NONE', #25783, #1801 ) ;
#23052=EDGE_CURVE ( 'NONE', #11337, #21626, #10321, .T. ) ;
#23054=VECTOR ( 'NONE', #3168, 1000.000000000000000 ) ;
#23058=ORIENTED_EDGE ( 'NONE', *, *, #14749, .F. ) ;
#23059=ORIENTED_EDGE ( 'NONE', *, *, #13657, .T. ) ;
#23065=EDGE_LOOP ( 'NONE', ( #11016, #12012, #372, #30015 ) ) ;
#23067=AXIS2_PLACEMENT_3D ( 'NONE', #12823, #22292, #17844 ) ;
#23069=CARTESIAN_POINT ( 'NONE',  ( 180.7287565553229456, -3.999999999999994671, 0.5000000000000029976 ) ) ;
#23070=CARTESIAN_POINT ( 'NONE',  ( 11.31764596240014598, -5.000000000000014211, 34.83213265805688508 ) ) ;
#23072=LINE ( 'NONE', #29852, #17361 ) ;
#23073=ORIENTED_EDGE ( 'NONE', *, *, #29578, .F. ) ;
#23077=VERTEX_POINT ( 'NONE', #24232 ) ;
#23078=FACE_OUTER_BOUND ( 'NONE', #667, .T. ) ;
#23079=VECTOR ( 'NONE', #3317, 999.9999999999998863 ) ;
#23080=CARTESIAN_POINT ( 'NONE',  ( 148.6922820468854241, -10.00000000000000178, -17.92658477444275889 ) ) ;
#23084=EDGE_CURVE ( 'NONE', #27188, #29946, #1495, .T. ) ;
#23085=EDGE_CURVE ( 'NONE', #26148, #20749, #3471, .T. ) ;
#23086=VERTEX_POINT ( 'NONE', #17494 ) ;
#23088=CARTESIAN_POINT ( 'NONE',  ( 99.29987472633386858, -4.999999999999990230, -72.14558201428623363 ) ) ;
#23089=CARTESIAN_POINT ( 'NONE',  ( 172.7287565553229456, -4.999999999999970690, 3.500000000000003109 ) ) ;
#23090=CARTESIAN_POINT ( 'NONE',  ( 129.5152310637605808, -10.00000000000000888, -2.627941064794695691 ) ) ;
#23091=VECTOR ( 'NONE', #6156, 1000.000000000000000 ) ;
#23093=LINE ( 'NONE', #27102, #22411 ) ;
#23094=ORIENTED_EDGE ( 'NONE', *, *, #29210, .F. ) ;
#23096=ORIENTED_EDGE ( 'NONE', *, *, #9926, .F. ) ;
#23102=ORIENTED_EDGE ( 'NONE', *, *, #10410, .T. ) ;
#23103=VERTEX_POINT ( 'NONE', #22547 ) ;
#23104=LINE ( 'NONE', #20500, #11519 ) ;
#23106=EDGE_CURVE ( 'NONE', #22675, #24876, #12913, .T. ) ;
#23108=CARTESIAN_POINT ( 'NONE',  ( 148.6922820468853956, -1.999999999999977129, -9.266330736598359152 ) ) ;
#23109=DIRECTION ( 'NONE',  ( 0.5877852522924731371, 0.000000000000000000, 0.8090169943749474513 ) ) ;
#23112=CARTESIAN_POINT ( 'NONE',  ( 158.6922820468853104, -4.999999999999974243, 2.247092850131519715 ) ) ;
#23116=VERTEX_POINT ( 'NONE', #26846 ) ;
#23117=CARTESIAN_POINT ( 'NONE',  ( 162.0152310637604671, -9.999999999999998224, -6.958068083716895558 ) ) ;
#23118=CARTESIAN_POINT ( 'NONE',  ( 132.0152310637605524, -4.999999999999982236, -26.04193191628310800 ) ) ;
#23119=DIRECTION ( 'NONE',  ( 0.5877852522924731371, 1.586114251531760728E-16, -0.8090169943749474513 ) ) ;
#23120=LINE ( 'NONE', #22531, #8666 ) ;
#23126=ORIENTED_EDGE ( 'NONE', *, *, #7945, .T. ) ;
#23129=VECTOR ( 'NONE', #29607, 1000.000000000000000 ) ;
#23131=DIRECTION ( 'NONE',  ( 0.9510565162951536422, 2.566386769018988816E-16, 0.3090169943749472292 ) ) ;
#23133=ORIENTED_EDGE ( 'NONE', *, *, #10559, .T. ) ;
#23134=CARTESIAN_POINT ( 'NONE',  ( 149.7287565553230309, -4.999999999999976907, -25.16025403784439973 ) ) ;
#23136=EDGE_CURVE ( 'NONE', #1908, #4171, #22228, .T. ) ;
#23137=ORIENTED_EDGE ( 'NONE', *, *, #7058, .F. ) ;
#23142=VERTEX_POINT ( 'NONE', #6060 ) ;
#23147=CARTESIAN_POINT ( 'NONE',  ( 157.2287565553230024, -4.999999999999975131, -29.49038105676660138 ) ) ;
#23149=VECTOR ( 'NONE', #19583, 1000.000000000000000 ) ;
#23152=LINE ( 'NONE', #25446, #15067 ) ;
#23154=ORIENTED_EDGE ( 'NONE', *, *, #29248, .F. ) ;
#23155=DIRECTION ( 'NONE',  ( -2.698458740408365879E-16, 1.000000000000000000, 0.000000000000000000 ) ) ;
#23156=DIRECTION ( 'NONE',  ( -2.698458740408365879E-16, 1.000000000000000000, 0.000000000000000000 ) ) ;
#23159=VERTEX_POINT ( 'NONE', #24683 ) ;
#23160=PLANE ( 'NONE',  #18563 ) ;
#23161=LINE ( 'NONE', #25458, #5033 ) ;
#23163=DIRECTION ( 'NONE',  ( -1.000000000000000000, -2.698458740408365879E-16, 0.000000000000000000 ) ) ;
#23164=CARTESIAN_POINT ( 'NONE',  ( 152.0152310637605808, -1.999999999999974465, -34.70218595412750773 ) ) ;
#23165=EDGE_CURVE ( 'NONE', #12496, #17958, #3773, .T. ) ;
#23167=VERTEX_POINT ( 'NONE', #15503 ) ;
#23168=DIRECTION ( 'NONE',  ( 0.9510565162951536422, 2.566386769018988816E-16, 0.3090169943749472292 ) ) ;
#23169=EDGE_CURVE ( 'NONE', #1890, #29392, #24834, .T. ) ;
#23170=VECTOR ( 'NONE', #25050, 1000.000000000000000 ) ;
#23172=EDGE_CURVE ( 'NONE', #25866, #12094, #28852, .T. ) ;
#23173=LINE ( 'NONE', #7300, #14956 ) ;
#23174=ORIENTED_EDGE ( 'NONE', *, *, #22881, .F. ) ;
#23179=DIRECTION ( 'NONE',  ( -2.698458740408365879E-16, 1.000000000000000000, 0.000000000000000000 ) ) ;
#23180=DIRECTION ( 'NONE',  ( -0.8090169943749474513, -2.183098979609982436E-16, -0.5877852522924731371 ) ) ;
#23183=VECTOR ( 'NONE', #16288, 1000.000000000000000 ) ;
#23184=CARTESIAN_POINT ( 'NONE',  ( 132.0152310637605808, -1.999999999999981348, 1.702185954127501066 ) ) ;
#23185=CARTESIAN_POINT ( 'NONE',  ( 13.94177938065702804, -5.000000000000014211, 42.90838487877751817 ) ) ;
#23186=PLANE ( 'NONE',  #16039 ) ;
#23187=VECTOR ( 'NONE', #28966, 1000.000000000000000 ) ;
#23188=DIRECTION ( 'NONE',  ( -2.698458740408365879E-16, 1.000000000000000000, 0.000000000000000000 ) ) ;
#23193=LINE ( 'NONE', #29526, #19959 ) ;
#23194=ORIENTED_EDGE ( 'NONE', *, *, #10098, .F. ) ;
#23196=ORIENTED_EDGE ( 'NONE', *, *, #21900, .T. ) ;
#23197=DIRECTION ( 'NONE',  ( -0.9510565162951536422, -2.566386769018988323E-16, 0.3090169943749475623 ) ) ;
#23201=ORIENTED_EDGE ( 'NONE', *, *, #23481, .F. ) ;
#23207=DIRECTION ( 'NONE',  ( -0.9510565162951536422, -2.566386769018988323E-16, 0.3090169943749475623 ) ) ;
#23208=DIRECTION ( 'NONE',  ( 0.5877852522924731371, 1.586114251531760728E-16, -0.8090169943749474513 ) ) ;
#23209=EDGE_CURVE ( 'NONE', #10712, #12856, #4220, .T. ) ;
#23211=ORIENTED_EDGE ( 'NONE', *, *, #7736, .T. ) ;
#23212=FACE_OUTER_BOUND ( 'NONE', #5337, .T. ) ;
#23213=EDGE_LOOP ( 'NONE', ( #28578, #27499, #17825, #27689 ) ) ;
#23221=LINE ( 'NONE', #27688, #4981 ) ;
#23226=CARTESIAN_POINT ( 'NONE',  ( 159.5152310637604671, -4.999999999999974243, -1.770974823053888726E-14 ) ) ;
#23228=ORIENTED_EDGE ( 'NONE', *, *, #2596, .F. ) ;
#23230=DIRECTION ( 'NONE',  ( 0.5877852522924731371, 1.586114251531760728E-16, 0.8090169943749474513 ) ) ;
#23231=VECTOR ( 'NONE', #9190, 1000.000000000000000 ) ;
#23232=PLANE ( 'NONE',  #9474 ) ;
#23233=AXIS2_PLACEMENT_3D ( 'NONE', #11922, #18804, #6920 ) ;
#23236=PLANE ( 'NONE',  #18735 ) ;
#23237=ORIENTED_EDGE ( 'NONE', *, *, #25287, .F. ) ;
#23239=VERTEX_POINT ( 'NONE', #27461 ) ;
#23241=ORIENTED_EDGE ( 'NONE', *, *, #16099, .T. ) ;
#23242=EDGE_CURVE ( 'NONE', #14016, #12198, #4518, .T. ) ;
#23243=EDGE_CURVE ( 'NONE', #10342, #16735, #13806, .T. ) ;
#23245=CARTESIAN_POINT ( 'NONE',  ( 152.0152310637604955, -4.999999999999976907, -1.687708096207002301E-14 ) ) ;
#23246=DIRECTION ( 'NONE',  ( 0.9510565162951536422, 2.566386769018988816E-16, 0.3090169943749472292 ) ) ;
#23247=EDGE_CURVE ( 'NONE', #21669, #19668, #1948, .T. ) ;
#23250=ORIENTED_EDGE ( 'NONE', *, *, #27617, .F. ) ;
#23251=DIRECTION ( 'NONE',  ( 0.5877852522924731371, 1.586114251531760728E-16, 0.8090169943749474513 ) ) ;
#23252=EDGE_CURVE ( 'NONE', #4418, #10720, #23285, .T. ) ;
#23256=LINE ( 'NONE', #13780, #5437 ) ;
#23257=AXIS2_PLACEMENT_3D ( 'NONE', #1260, #3112, #21851 ) ;
#23258=CARTESIAN_POINT ( 'NONE',  ( 164.5152310637604387, -9.999999999999998224, -4.391296821672111328 ) ) ;
#23262=ORIENTED_EDGE ( 'NONE', *, *, #6151, .T. ) ;
#23264=VECTOR ( 'NONE', #12204, 1000.000000000000000 ) ;
#23266=ORIENTED_EDGE ( 'NONE', *, *, #15965, .F. ) ;
#23267=DIRECTION ( 'NONE',  ( -1.000000000000000000, 0.000000000000000000, 0.000000000000000000 ) ) ;
#23269=CARTESIAN_POINT ( 'NONE',  ( 173.6922820468853388, -9.999999999999994671, -26.58683881228715862 ) ) ;
#23270=CARTESIAN_POINT ( 'NONE',  ( 169.7287565553229172, -4.999999999999972466, -7.839745962155600267 ) ) ;
#23276=ORIENTED_EDGE ( 'NONE', *, *, #14091, .F. ) ;
#23280=DIRECTION ( 'NONE',  ( -0.5877852522924731371, 0.000000000000000000, 0.8090169943749474513 ) ) ;
#23281=CARTESIAN_POINT ( 'NONE',  ( 134.5152310637605524, -1.999999999999980460, -30.37205893520530964 ) ) ;
#23282=ADVANCED_FACE ( 'NONE', ( #29921 ), #18550, .T. ) ;
#23284=ORIENTED_EDGE ( 'NONE', *, *, #26974, .F. ) ;
#23285=LINE ( 'NONE', #8635, #20261 ) ;
#23286=ADVANCED_FACE ( 'NONE', ( #20382 ), #30213, .T. ) ;
#23288=VERTEX_POINT ( 'NONE', #23134 ) ;
#23289=PLANE ( 'NONE',  #22248 ) ;
#23290=PLANE ( 'NONE',  #22491 ) ;
#23292=VERTEX_POINT ( 'NONE', #27601 ) ;
#23293=ORIENTED_EDGE ( 'NONE', *, *, #29993, .F. ) ;
#23297=VECTOR ( 'NONE', #8737, 1000.000000000000000 ) ;
#23299=VECTOR ( 'NONE', #20024, 1000.000000000000000 ) ;
#23300=ORIENTED_EDGE ( 'NONE', *, *, #14691, .T. ) ;
#23301=FACE_OUTER_BOUND ( 'NONE', #4930, .T. ) ;
#23302=ORIENTED_EDGE ( 'NONE', *, *, #5600, .T. ) ;
#23303=EDGE_CURVE ( 'NONE', #15830, #27224, #9222, .T. ) ;
#23305=VERTEX_POINT ( 'NONE', #8782 ) ;
#23306=DIRECTION ( 'NONE',  ( -0.5877852522924731371, 0.000000000000000000, 0.8090169943749474513 ) ) ;
#23307=DIRECTION ( 'NONE',  ( -0.9510565162951536422, -2.566386769018988816E-16, -0.3090169943749472292 ) ) ;
#23310=ORIENTED_EDGE ( 'NONE', *, *, #6057, .F. ) ;
#23313=PLANE ( 'NONE',  #8451 ) ;
#23316=CARTESIAN_POINT ( 'NONE',  ( 137.0152310637605524, -1.999999999999980016, -0.06116980274991495881 ) ) ;
#23317=ORIENTED_EDGE ( 'NONE', *, *, #25324, .T. ) ;
#23321=EDGE_LOOP ( 'NONE', ( #22484, #320, #19398, #26906 ) ) ;
#23322=CARTESIAN_POINT ( 'NONE',  ( 147.0152310637605808, -10.00000000000000178, -15.61832212156129707 ) ) ;
#23323=VERTEX_POINT ( 'NONE', #27311 ) ;
#23329=DIRECTION ( 'NONE',  ( -2.698458740408365879E-16, 1.000000000000000000, 0.000000000000000000 ) ) ;
#23331=CARTESIAN_POINT ( 'NONE',  ( 6.227276357848867683, -5.000000000000015987, 19.16558592799212235 ) ) ;
#23333=CARTESIAN_POINT ( 'NONE',  ( 148.6922820468853956, -10.00000000000000178, -6.413161187712876909 ) ) ;
#23336=EDGE_CURVE ( 'NONE', #29174, #16977, #27907, .T. ) ;
#23337=AXIS2_PLACEMENT_3D ( 'NONE', #22184, #17452, #3293 ) ;
#23338=FACE_OUTER_BOUND ( 'NONE', #9180, .T. ) ;
#23339=EDGE_CURVE ( 'NONE', #24460, #21674, #4369, .T. ) ;
#23340=FACE_OUTER_BOUND ( 'NONE', #14461, .T. ) ;
#23341=DIRECTION ( 'NONE',  ( -2.698458740408365879E-16, 1.000000000000000000, 0.000000000000000000 ) ) ;
#23342=VECTOR ( 'NONE', #2903, 999.9999999999998863 ) ;
#23344=LINE ( 'NONE', #27517, #14050 ) ;
#23347=VERTEX_POINT ( 'NONE', #4659 ) ;
#23353=DIRECTION ( 'NONE',  ( 0.000000000000000000, -0.7071067811865456854, -0.7071067811865493491 ) ) ;
#23354=EDGE_LOOP ( 'NONE', ( #1653, #214, #10838, #29163 ) ) ;
#23355=VERTEX_POINT ( 'NONE', #11374 ) ;
#23359=DIRECTION ( 'NONE',  ( -0.9510565162951536422, -2.566386769018988816E-16, -0.3090169943749472292 ) ) ;
#23360=DIRECTION ( 'NONE',  ( -2.698458740408365879E-16, 1.000000000000000000, 0.000000000000000000 ) ) ;
#23361=ORIENTED_EDGE ( 'NONE', *, *, #29248, .T. ) ;
#23362=LINE ( 'NONE', #4892, #21774 ) ;
#23363=EDGE_LOOP ( 'NONE', ( #26939, #7800, #25508, #3656, #22407 ) ) ;
#23366=AXIS2_PLACEMENT_3D ( 'NONE', #19546, #15566, #18159 ) ;
#23370=VECTOR ( 'NONE', #8653, 1000.000000000000000 ) ;
#23375=ORIENTED_EDGE ( 'NONE', *, *, #5295, .T. ) ;
#23376=FACE_BOUND ( 'NONE', #10504, .T. ) ;
#23377=EDGE_CURVE ( 'NONE', #23552, #19492, #18401, .T. ) ;
#23378=EDGE_CURVE ( 'NONE', #30087, #17576, #25428, .T. ) ;
#23379=EDGE_CURVE ( 'NONE', #6014, #3793, #19007, .T. ) ;
#23380=EDGE_CURVE ( 'NONE', #26115, #21455, #25888, .T. ) ;
#23381=EDGE_LOOP ( 'NONE', ( #6611, #7074, #15726, #10474, #20719 ) ) ;
#23382=VECTOR ( 'NONE', #20446, 1000.000000000000000 ) ;
#23383=CARTESIAN_POINT ( 'NONE',  ( 141.1922820468854525, -1.999999999999978684, -13.59645775552055902 ) ) ;
#23384=VECTOR ( 'NONE', #25347, 1000.000000000000000 ) ;
#23385=DIRECTION ( 'NONE',  ( -2.698458740408365879E-16, 1.000000000000000000, 0.000000000000000000 ) ) ;
#23386=DIRECTION ( 'NONE',  ( -0.9510565162951536422, -2.566386769018988323E-16, 0.3090169943749475623 ) ) ;
#23387=VECTOR ( 'NONE', #22790, 1000.000000000000000 ) ;
#23390=DIRECTION ( 'NONE',  ( -0.8090169943749474513, -2.183098979609982436E-16, 0.5877852522924731371 ) ) ;
#23391=ORIENTED_EDGE ( 'NONE', *, *, #27287, .T. ) ;
#23392=DIRECTION ( 'NONE',  ( -0.5877852522924731371, -1.586114251531760728E-16, -0.8090169943749474513 ) ) ;
#23393=ORIENTED_EDGE ( 'NONE', *, *, #2274, .F. ) ;
#23397=CARTESIAN_POINT ( 'NONE',  ( 169.5152310637604955, -4.999999999999971578, -30.37205893520531319 ) ) ;
#23398=LINE ( 'NONE', #16818, #842 ) ;
#23400=ORIENTED_EDGE ( 'NONE', *, *, #6151, .F. ) ;
#23403=ORIENTED_EDGE ( 'NONE', *, *, #18099, .F. ) ;
#23406=DIRECTION ( 'NONE',  ( -0.9510565162951536422, 0.000000000000000000, -0.3090169943749472292 ) ) ;
#23409=CARTESIAN_POINT ( 'NONE',  ( 130.7287565553229456, -4.999999999999983125, 0.5000000000000052180 ) ) ;
#23411=VECTOR ( 'NONE', #8927, 1000.000000000000000 ) ;
#23414=VECTOR ( 'NONE', #27734, 1000.000000000000000 ) ;
#23416=LINE ( 'NONE', #7246, #5376 ) ;
#23417=EDGE_CURVE ( 'NONE', #6582, #29656, #21599, .T. ) ;
#23418=ADVANCED_FACE ( 'NONE', ( #28364 ), #9984, .T. ) ;
#23419=EDGE_CURVE ( 'NONE', #3706, #2025, #23440, .T. ) ;
#23420=CARTESIAN_POINT ( 'NONE',  ( 157.2287565553230024, -1.999999999999973133, -29.49038105676660493 ) ) ;
#23422=EDGE_CURVE ( 'NONE', #26303, #9856, #16862, .T. ) ;
#23424=CARTESIAN_POINT ( 'NONE',  ( 172.2287565553229172, -9.999999999999996447, -20.83012701892220520 ) ) ;
#23425=CARTESIAN_POINT ( 'NONE',  ( 139.5152310637605808, -4.999999999999980460, -1.548930218128858680E-14 ) ) ;
#23427=DIRECTION ( 'NONE',  ( 0.9510565162951535312, 2.566386769018988816E-16, -0.3090169943749475623 ) ) ;
#23432=ORIENTED_EDGE ( 'NONE', *, *, #15030, .T. ) ;
#23433=AXIS2_PLACEMENT_3D ( 'NONE', #10344, #12326, #8204 ) ;
#23436=FACE_OUTER_BOUND ( 'NONE', #20945, .T. ) ;
#23437=CARTESIAN_POINT ( 'NONE',  ( 173.6922820468852535, -4.999999999999971578, -0.6060766987539614181 ) ) ;
#23440=LINE ( 'NONE', #14256, #11982 ) ;
#23443=DIRECTION ( 'NONE',  ( 0.5877852522924731371, 0.000000000000000000, 0.8090169943749474513 ) ) ;
#23444=CARTESIAN_POINT ( 'NONE',  ( 178.7287565553229172, -1.999999999999968914, 0.5000000000000029976 ) ) ;
#23448=ORIENTED_EDGE ( 'NONE', *, *, #10002, .F. ) ;
#23452=VECTOR ( 'NONE', #26762, 1000.000000000000000 ) ;
#23456=EDGE_CURVE ( 'NONE', #2040, #1623, #5273, .T. ) ;
#23457=VERTEX_POINT ( 'NONE', #19299 ) ;
#23459=PLANE ( 'NONE',  #27489 ) ;
#23460=ADVANCED_FACE ( 'NONE', ( #9682 ), #11823, .T. ) ;
#23461=CARTESIAN_POINT ( 'NONE',  ( 137.0152310637606092, -10.00000000000000533, -24.27857615940569147 ) ) ;
#23462=DIRECTION ( 'NONE',  ( -0.9510565162951536422, 0.000000000000000000, -0.3090169943749472292 ) ) ;
#23463=DIRECTION ( 'NONE',  ( 0.000000000000000000, 0.000000000000000000, -1.000000000000000000 ) ) ;
#23467=VERTEX_POINT ( 'NONE', #25731 ) ;
#23469=DIRECTION ( 'NONE',  ( 1.110223024625156540E-16, 2.995891024602366092E-32, 1.000000000000000000 ) ) ;
#23472=ORIENTED_EDGE ( 'NONE', *, *, #27005, .T. ) ;
#23473=CARTESIAN_POINT ( 'NONE',  ( 122.6304986437925209, -4.999999999999984901, -89.09627249521899728 ) ) ;
#23474=ORIENTED_EDGE ( 'NONE', *, *, #24908, .T. ) ;
#23475=LINE ( 'NONE', #4413, #17811 ) ;
#23476=PLANE ( 'NONE',  #16597 ) ;
#23477=ORIENTED_EDGE ( 'NONE', *, *, #28318, .T. ) ;
#23478=CARTESIAN_POINT ( 'NONE',  ( 18.54986643893153442, -5.000000000000012434, -57.09061855589936840 ) ) ;
#23479=EDGE_LOOP ( 'NONE', ( #23317, #23400, #8522, #3143 ) ) ;
#23481=EDGE_CURVE ( 'NONE', #24269, #24460, #23748, .T. ) ;
#23482=ORIENTED_EDGE ( 'NONE', *, *, #6856, .F. ) ;
#23485=CARTESIAN_POINT ( 'NONE',  ( 149.5152310637605240, -10.00000000000000178, -13.05155085951651195 ) ) ;
#23486=LINE ( 'NONE', #16156, #10154 ) ;
#23487=CARTESIAN_POINT ( 'NONE',  ( 134.7287565553230024, -4.999999999999981348, -7.839745962155600267 ) ) ;
#23489=DIRECTION ( 'NONE',  ( 0.000000000000000000, 0.000000000000000000, -1.000000000000000000 ) ) ;
#23490=LINE ( 'NONE', #2600, #21408 ) ;
#23492=DIRECTION ( 'NONE',  ( 0.3090169943749472292, 8.338696094057992503E-17, -0.9510565162951536422 ) ) ;
#23493=FACE_OUTER_BOUND ( 'NONE', #236, .T. ) ;
#23500=PLANE ( 'NONE',  #22707 ) ;
#23501=VECTOR ( 'NONE', #4459, 1000.000000000000000 ) ;
#23504=FACE_BOUND ( 'NONE', #12698, .T. ) ;
#23506=ORIENTED_EDGE ( 'NONE', *, *, #9021, .T. ) ;
#23508=FACE_OUTER_BOUND ( 'NONE', #25841, .T. ) ;
#23511=CARTESIAN_POINT ( 'NONE',  ( 169.5152310637604387, -9.999999999999996447, -2.627941064794695691 ) ) ;
#23514=VERTEX_POINT ( 'NONE', #250 ) ;
#23516=EDGE_CURVE ( 'NONE', #25495, #18619, #26194, .T. ) ;
#23517=ORIENTED_EDGE ( 'NONE', *, *, #9202, .T. ) ;
#23522=EDGE_CURVE ( 'NONE', #19955, #23305, #3003, .T. ) ;
#23531=VECTOR ( 'NONE', #9959, 1000.000000000000000 ) ;
#23532=VERTEX_POINT ( 'NONE', #17020 ) ;
#23533=CARTESIAN_POINT ( 'NONE',  ( 153.6922820468853672, -10.00000000000000178, -6.413161187712876909 ) ) ;
#23535=CARTESIAN_POINT ( 'NONE',  ( 161.1922820468853956, -1.999999999999972689, -30.91696583120936026 ) ) ;
#23537=VECTOR ( 'NONE', #19649, 1000.000000000000000 ) ;
#23538=CARTESIAN_POINT ( 'NONE',  ( 162.2287565553229172, -9.999999999999998224, -12.16987298107780369 ) ) ;
#23541=PLANE ( 'NONE',  #5857 ) ;
#23542=CARTESIAN_POINT ( 'NONE',  ( 134.7287565553230024, -1.999999999999980460, 0.8205080756887930260 ) ) ;
#23543=VERTEX_POINT ( 'NONE', #18849 ) ;
#23545=VERTEX_POINT ( 'NONE', #28210 ) ;
#23547=VECTOR ( 'NONE', #16767, 1000.000000000000000 ) ;
#23552=VERTEX_POINT ( 'NONE', #26344 ) ;
#23553=CARTESIAN_POINT ( 'NONE',  ( 171.1922820468853104, -1.999999999999970468, -10.74328820663507678 ) ) ;
#23555=ORIENTED_EDGE ( 'NONE', *, *, #18303, .F. ) ;
#23556=EDGE_CURVE ( 'NONE', #7790, #3713, #19154, .T. ) ;
#23558=PLANE ( 'NONE',  #4922 ) ;
#23559=EDGE_LOOP ( 'NONE', ( #25145, #23021, #11776, #28982, #19372, #14378 ) ) ;
#23560=ADVANCED_FACE ( 'NONE', ( #557 ), #9841, .T. ) ;
#23561=LINE ( 'NONE', #12098, #18393 ) ;
#23562=EDGE_CURVE ( 'NONE', #23077, #10756, #9379, .T. ) ;
#23565=CARTESIAN_POINT ( 'NONE',  ( 89.72970066344139184, -4.999999999999992895, 65.19244355718100792 ) ) ;
#23573=ORIENTED_EDGE ( 'NONE', *, *, #19383, .T. ) ;
#23574=CARTESIAN_POINT ( 'NONE',  ( 169.5152310637605240, -1.999999999999970024, -28.60870317832789667 ) ) ;
#23575=CARTESIAN_POINT ( 'NONE',  ( 147.0152310637605240, -10.00000000000000178, -8.721423840594312082 ) ) ;
#23583=CARTESIAN_POINT ( 'NONE',  ( 138.6922820468854525, -10.00000000000000533, -17.92658477444275533 ) ) ;
#23584=DIRECTION ( 'NONE',  ( 0.9510565162951535312, 2.566386769018988816E-16, -0.3090169943749475623 ) ) ;
#23585=DIRECTION ( 'NONE',  ( 1.110223024625156540E-16, 2.995891024602366092E-32, 1.000000000000000000 ) ) ;
#23587=ORIENTED_EDGE ( 'NONE', *, *, #1847, .F. ) ;
#23588=CARTESIAN_POINT ( 'NONE',  ( 172.0152310637604671, -9.999999999999994671, -26.04193191628311155 ) ) ;
#23590=ORIENTED_EDGE ( 'NONE', *, *, #17441, .F. ) ;
#23591=CARTESIAN_POINT ( 'NONE',  ( 138.6922820468854241, -4.999999999999980460, -0.6060766987539614181 ) ) ;
#23592=CARTESIAN_POINT ( 'NONE',  ( 8.531849494005609102, -5.000000000000015099, 26.25833272935806662 ) ) ;
#23593=EDGE_CURVE ( 'NONE', #11963, #3548, #10434, .T. ) ;
#23595=VECTOR ( 'NONE', #14915, 1000.000000000000000 ) ;
#23599=ORIENTED_EDGE ( 'NONE', *, *, #3281, .T. ) ;
#23604=VERTEX_POINT ( 'NONE', #5729 ) ;
#23607=ORIENTED_EDGE ( 'NONE', *, *, #26927, .F. ) ;
#23608=LINE ( 'NONE', #10153, #6977 ) ;
#23609=LINE ( 'NONE', #25585, #27318 ) ;
#23610=ORIENTED_EDGE ( 'NONE', *, *, #25412, .F. ) ;
#23612=AXIS2_PLACEMENT_3D ( 'NONE', #26369, #574, #12152 ) ;
#23616=ORIENTED_EDGE ( 'NONE', *, *, #14093, .T. ) ;
#23618=LINE ( 'NONE', #19034, #5655 ) ;
#23621=ORIENTED_EDGE ( 'NONE', *, *, #22317, .T. ) ;
#23623=ORIENTED_EDGE ( 'NONE', *, *, #20544, .F. ) ;
#23624=ORIENTED_EDGE ( 'NONE', *, *, #178, .T. ) ;
#23625=DIRECTION ( 'NONE',  ( -0.5877852522924731371, -1.586114251531760235E-16, 0.8090169943749474513 ) ) ;
#23626=EDGE_CURVE ( 'NONE', #7033, #6062, #29430, .T. ) ;
#23627=CARTESIAN_POINT ( 'NONE',  ( 167.0152310637605240, -1.999999999999970912, -24.27857615940569502 ) ) ;
#23628=ORIENTED_EDGE ( 'NONE', *, *, #15235, .F. ) ;
#23631=EDGE_LOOP ( 'NONE', ( #28974, #28543, #2923, #18137 ) ) ;
#23632=EDGE_CURVE ( 'NONE', #19861, #10906, #6026, .T. ) ;
#23637=CARTESIAN_POINT ( 'NONE',  ( 169.7287565553228603, -9.999999999999998224, 0.8205080756887930260 ) ) ;
#23638=LINE ( 'NONE', #7010, #5289 ) ;
#23639=VECTOR ( 'NONE', #6916, 1000.000000000000000 ) ;
#23640=DIRECTION ( 'NONE',  ( -0.9510565162951536422, -2.566386769018988323E-16, 0.3090169943749475623 ) ) ;
#23642=VERTEX_POINT ( 'NONE', #17609 ) ;
#23643=FILL_AREA_STYLE_COLOUR ( '', #24212 ) ;
#23644=CARTESIAN_POINT ( 'NONE',  ( 131.1922820468854241, -10.00000000000000888, -19.40354224447947473 ) ) ;
#23645=CARTESIAN_POINT ( 'NONE',  ( 169.5152310637604955, -9.999999999999994671, -30.37205893520531319 ) ) ;
#23646=CARTESIAN_POINT ( 'NONE',  ( 156.1922820468853672, -1.999999999999974909, -13.59645775552055902 ) ) ;
#23647=LINE ( 'NONE', #9591, #199 ) ;
#23649=DIRECTION ( 'NONE',  ( -2.698458740408365879E-16, 1.000000000000000000, 0.000000000000000000 ) ) ;
#23651=ORIENTED_EDGE ( 'NONE', *, *, #4059, .F. ) ;
#23653=ORIENTED_EDGE ( 'NONE', *, *, #11481, .T. ) ;
#23654=CARTESIAN_POINT ( 'NONE',  ( 137.0152310637606092, -1.999999999999979572, -6.958068083716895558 ) ) ;
#23655=VECTOR ( 'NONE', #16319, 1000.000000000000000 ) ;
#23659=ORIENTED_EDGE ( 'NONE', *, *, #12338, .F. ) ;
#23660=VERTEX_POINT ( 'NONE', #20056 ) ;
#23662=DIRECTION ( 'NONE',  ( -2.698458740408365879E-16, 1.000000000000000000, 0.000000000000000000 ) ) ;
#23665=EDGE_LOOP ( 'NONE', ( #29259, #14639, #15058, #21786 ) ) ;
#23667=EDGE_LOOP ( 'NONE', ( #25758, #4546, #20577, #263 ) ) ;
#23668=EDGE_CURVE ( 'NONE', #3067, #15263, #12576, .T. ) ;
#23670=VECTOR ( 'NONE', #15799, 1000.000000000000000 ) ;
#23671=ORIENTED_EDGE ( 'NONE', *, *, #5398, .F. ) ;
#23675=EDGE_LOOP ( 'NONE', ( #3253, #5968, #21206, #15841 ) ) ;
#23680=AXIS2_PLACEMENT_3D ( 'NONE', #9563, #881, #21321 ) ;
#23682=VECTOR ( 'NONE', #24985, 1000.000000000000000 ) ;
#23683=ORIENTED_EDGE ( 'NONE', *, *, #7605, .F. ) ;
#23684=ORIENTED_EDGE ( 'NONE', *, *, #22460, .F. ) ;
#23685=PLANE ( 'NONE',  #13760 ) ;
#23687=LINE ( 'NONE', #642, #7721 ) ;
#23688=DIRECTION ( 'NONE',  ( 0.5877852522924731371, 1.586114251531760728E-16, -0.8090169943749474513 ) ) ;
#23689=CARTESIAN_POINT ( 'NONE',  ( 130.7287565553229172, -4.999999999999983125, -36.50000000000000711 ) ) ;
#23690=LINE ( 'NONE', #23538, #1732 ) ;
#23691=VECTOR ( 'NONE', #29473, 1000.000000000000000 ) ;
#23693=DIRECTION ( 'NONE',  ( 0.9510565162951535312, 2.566386769018988816E-16, -0.3090169943749475623 ) ) ;
#23694=PLANE ( 'NONE',  #9081 ) ;
#23695=VERTEX_POINT ( 'NONE', #1155 ) ;
#23696=VECTOR ( 'NONE', #5115, 1000.000000000000000 ) ;
#23700=AXIS2_PLACEMENT_3D ( 'NONE', #27512, #1548, #20439 ) ;
#23702=CARTESIAN_POINT ( 'NONE',  ( 133.6922820468854241, -1.999999999999981348, -35.24709285013155835 ) ) ;
#23703=CARTESIAN_POINT ( 'NONE',  ( 83.60744220746381927, -4.999999999999994671, 60.74436242147287146 ) ) ;
#23705=ORIENTED_EDGE ( 'NONE', *, *, #13073, .T. ) ;
#23706=VERTEX_POINT ( 'NONE', #22192 ) ;
#23707=CARTESIAN_POINT ( 'NONE',  ( 118.0894766101636719, -4.999999999999985789, -85.79702686717824633 ) ) ;
#23712=CARTESIAN_POINT ( 'NONE',  ( 153.6922820468854525, -10.00000000000000000, -35.24709285013155835 ) ) ;
#23715=VERTEX_POINT ( 'NONE', #8152 ) ;
#23716=DIRECTION ( 'NONE',  ( 2.908569913943825554E-16, -1.000000000000000000, 0.000000000000000000 ) ) ;
#23721=ORIENTED_EDGE ( 'NONE', *, *, #20037, .T. ) ;
#23722=DIRECTION ( 'NONE',  ( -2.698458740408365879E-16, 1.000000000000000000, 0.000000000000000000 ) ) ;
#23724=ORIENTED_EDGE ( 'NONE', *, *, #446, .F. ) ;
#23725=FACE_OUTER_BOUND ( 'NONE', #23665, .T. ) ;
#23726=VECTOR ( 'NONE', #6327, 1000.000000000000000 ) ;
#23727=VECTOR ( 'NONE', #11182, 1000.000000000000000 ) ;
#23728=CARTESIAN_POINT ( 'NONE',  ( 167.0152310637604103, -1.999999999999972244, -0.06116980274991495881 ) ) ;
#23729=EDGE_CURVE ( 'NONE', #29571, #25565, #1010, .T. ) ;
#23730=EDGE_CURVE ( 'NONE', #17680, #7231, #3301, .T. ) ;
#23733=EDGE_CURVE ( 'NONE', #25583, #10712, #19743, .T. ) ;
#23734=LINE ( 'NONE', #23894, #19241 ) ;
#23735=ADVANCED_FACE ( 'NONE', ( #13035 ), #5880, .T. ) ;
#23740=ORIENTED_EDGE ( 'NONE', *, *, #18897, .T. ) ;
#23741=DIRECTION ( 'NONE',  ( 0.5877852522924731371, 1.586114251531760728E-16, 0.8090169943749474513 ) ) ;
#23742=CARTESIAN_POINT ( 'NONE',  ( 132.2287565553230024, -1.999999999999981348, -12.16987298107780013 ) ) ;
#23743=AXIS2_PLACEMENT_3D ( 'NONE', #27725, #29895, #9046 ) ;
#23744=LINE ( 'NONE', #2841, #13653 ) ;
#23747=ORIENTED_EDGE ( 'NONE', *, *, #17787, .T. ) ;
#23748=LINE ( 'NONE', #16720, #18806 ) ;
#23750=DIRECTION ( 'NONE',  ( -2.698458740408365879E-16, 1.000000000000000000, 0.000000000000000000 ) ) ;
#23751=CARTESIAN_POINT ( 'NONE',  ( 158.6922820468853388, -10.00000000000000000, -9.266330736598359152 ) ) ;
#23752=VECTOR ( 'NONE', #8487, 1000.000000000000000 ) ;
#23755=VERTEX_POINT ( 'NONE', #24497 ) ;
#23759=VERTEX_POINT ( 'NONE', #10748 ) ;
#23762=ORIENTED_EDGE ( 'NONE', *, *, #13651, .F. ) ;
#23763=VERTEX_POINT ( 'NONE', #1302 ) ;
#23764=FACE_OUTER_BOUND ( 'NONE', #10953, .T. ) ;
#23768=VECTOR ( 'NONE', #5888, 1000.000000000000000 ) ;
#23769=EDGE_CURVE ( 'NONE', #3794, #10636, #8302, .T. ) ;
#23770=ADVANCED_FACE ( 'NONE', ( #10137 ), #12427, .T. ) ;
#23771=CARTESIAN_POINT ( 'NONE',  ( 158.6922820468853104, -10.00000000000000000, 2.247092850131519715 ) ) ;
#23772=EDGE_CURVE ( 'NONE', #17665, #29503, #18360, .T. ) ;
#23773=DIRECTION ( 'NONE',  ( -2.698458740408365879E-16, 1.000000000000000000, 0.000000000000000000 ) ) ;
#23778=CARTESIAN_POINT ( 'NONE',  ( 136.1922820468854241, -10.00000000000000533, -30.91696583120935671 ) ) ;
#23779=LINE ( 'NONE', #21472, #2245 ) ;
#23782=DIRECTION ( 'NONE',  ( -1.110223024625156540E-16, 0.000000000000000000, -1.000000000000000000 ) ) ;
#23783=EDGE_LOOP ( 'NONE', ( #28956, #18506, #27495, #24150 ) ) ;
#23784=FACE_OUTER_BOUND ( 'NONE', #21677, .T. ) ;
#23785=VECTOR ( 'NONE', #22215, 1000.000000000000000 ) ;
#23786=DIRECTION ( 'NONE',  ( 0.5877852522924731371, 1.586114251531760728E-16, 0.8090169943749474513 ) ) ;
#23787=ORIENTED_EDGE ( 'NONE', *, *, #7058, .T. ) ;
#23788=CARTESIAN_POINT ( 'NONE',  ( 153.6922820468853388, -10.00000000000000178, -0.6060766987539614181 ) ) ;
#23791=AXIS2_PLACEMENT_3D ( 'NONE', #28588, #7641, #7350 ) ;
#23794=DIRECTION ( 'NONE',  ( -2.698458740408365879E-16, 1.000000000000000000, 0.000000000000000000 ) ) ;
#23795=LINE ( 'NONE', #3195, #24797 ) ;
#23796=DIRECTION ( 'NONE',  ( -2.698458740408366372E-16, 1.000000000000000000, 0.000000000000000000 ) ) ;
#23797=VECTOR ( 'NONE', #20629, 999.9999999999998863 ) ;
#23799=DIRECTION ( 'NONE',  ( -0.9510565162951536422, -2.566386769018988816E-16, -0.3090169943749472292 ) ) ;
#23801=FACE_OUTER_BOUND ( 'NONE', #22067, .T. ) ;
#23802=EDGE_CURVE ( 'NONE', #6477, #17665, #16068, .T. ) ;
#23803=ADVANCED_FACE ( 'NONE', ( #22655 ), #24799, .T. ) ;
#23804=VECTOR ( 'NONE', #1780, 1000.000000000000000 ) ;
#23806=LINE ( 'NONE', #2905, #14307 ) ;
#23807=EDGE_CURVE ( 'NONE', #10786, #23763, #4037, .T. ) ;
#23808=EDGE_CURVE ( 'NONE', #11673, #19955, #797, .T. ) ;
#23810=DIRECTION ( 'NONE',  ( 0.5877852522924731371, 0.000000000000000000, 0.8090169943749474513 ) ) ;
#23812=VECTOR ( 'NONE', #18602, 1000.000000000000000 ) ;
#23813=ORIENTED_EDGE ( 'NONE', *, *, #7201, .F. ) ;
#23817=FACE_BOUND ( 'NONE', #22237, .T. ) ;
#23818=VECTOR ( 'NONE', #14902, 1000.000000000000000 ) ;
#23823=CARTESIAN_POINT ( 'NONE',  ( 88.46122111574997859, -4.999999999999992895, 64.27083921987819792 ) ) ;
#23826=CARTESIAN_POINT ( 'NONE',  ( 162.0152310637604671, -1.999999999999972689, -17.38167787843871182 ) ) ;
#23827=ORIENTED_EDGE ( 'NONE', *, *, #8240, .F. ) ;
#23829=ORIENTED_EDGE ( 'NONE', *, *, #24109, .T. ) ;
#23834=CARTESIAN_POINT ( 'NONE',  ( 133.6922820468854241, -1.999999999999981348, -35.24709285013155835 ) ) ;
#23837=EDGE_CURVE ( 'NONE', #21323, #12653, #23104, .T. ) ;
#23843=FACE_BOUND ( 'NONE', #7126, .T. ) ;
#23844=AXIS2_PLACEMENT_3D ( 'NONE', #1326, #457, #19063 ) ;
#23845=EDGE_CURVE ( 'NONE', #14013, #16928, #1913, .T. ) ;
#23846=EDGE_CURVE ( 'NONE', #2926, #13701, #13476, .T. ) ;
#23847=EDGE_CURVE ( 'NONE', #29946, #9369, #6478, .T. ) ;
#23848=CARTESIAN_POINT ( 'NONE',  ( 131.1922820468854241, -1.999999999999981792, -10.74328820663507322 ) ) ;
#23850=LINE ( 'NONE', #14209, #25814 ) ;
#23851=CARTESIAN_POINT ( 'NONE',  ( 133.6922820468854241, -4.999999999999982236, -17.92658477444275533 ) ) ;
#23852=PRODUCT_DEFINITION_CONTEXT ( 'detailed design', #17667, 'design' ) ;
#23854=CARTESIAN_POINT ( 'NONE',  ( 147.0152310637605808, -10.00000000000000178, -26.04193191628311155 ) ) ;
#23855=ORIENTED_EDGE ( 'NONE', *, *, #20817, .F. ) ;
#23856=VECTOR ( 'NONE', #22140, 1000.000000000000000 ) ;
#23857=DIRECTION ( 'NONE',  ( 0.9510565162951535312, 2.566386769018988816E-16, -0.3090169943749475623 ) ) ;
#23858=VERTEX_POINT ( 'NONE', #15768 ) ;
#23860=EDGE_LOOP ( 'NONE', ( #15894, #5071, #27413, #4733 ) ) ;
#23863=LINE ( 'NONE', #21557, #19342 ) ;
#23864=DIRECTION ( 'NONE',  ( 0.5877852522924731371, 0.000000000000000000, 0.8090169943749474513 ) ) ;
#23865=VECTOR ( 'NONE', #9396, 1000.000000000000000 ) ;
#23866=CARTESIAN_POINT ( 'NONE',  ( 164.7287565553229456, -1.999999999999971356, -25.16025403784440329 ) ) ;
#23868=ORIENTED_EDGE ( 'NONE', *, *, #10733, .T. ) ;
#23872=PLANE ( 'NONE',  #5731 ) ;
#23875=ORIENTED_EDGE ( 'NONE', *, *, #28282, .T. ) ;
#23877=EDGE_CURVE ( 'NONE', #1409, #5536, #2060, .T. ) ;
#23879=EDGE_CURVE ( 'NONE', #600, #2712, #18515, .T. ) ;
#23884=EDGE_LOOP ( 'NONE', ( #20870, #19875, #2799, #24745 ) ) ;
#23885=ORIENTED_EDGE ( 'NONE', *, *, #8582, .T. ) ;
#23887=VECTOR ( 'NONE', #6402, 1000.000000000000000 ) ;
#23890=DIRECTION ( 'NONE',  ( -0.8090169943749474513, -2.183098979609982436E-16, 0.5877852522924731371 ) ) ;
#23891=VECTOR ( 'NONE', #24821, 1000.000000000000000 ) ;
#23892=PLANE ( 'NONE',  #21736 ) ;
#23893=DIRECTION ( 'NONE',  ( 1.000000000000000000, 2.698458740408365879E-16, -1.110223024625156540E-16 ) ) ;
#23894=CARTESIAN_POINT ( 'NONE',  ( 169.5152310637604387, -4.999999999999971578, -1.881997125516404065E-14 ) ) ;
#23899=ORIENTED_EDGE ( 'NONE', *, *, #6300, .T. ) ;
#23900=LINE ( 'NONE', #26488, #7095 ) ;
#23901=DIRECTION ( 'NONE',  ( 0.5877852522924731371, 1.586114251531760728E-16, 0.8090169943749474513 ) ) ;
#23903=DIRECTION ( 'NONE',  ( -2.698458740408365879E-16, 1.000000000000000000, 0.000000000000000000 ) ) ;
#23906=PRODUCT_DEFINITION_FORMATION_WITH_SPECIFIED_SOURCE ( 'ANY', '', #1074, .NOT_KNOWN. ) ;
#23907=ORIENTED_EDGE ( 'NONE', *, *, #18939, .T. ) ;
#23908=DIRECTION ( 'NONE',  ( -2.698458740408365879E-16, 1.000000000000000000, 0.000000000000000000 ) ) ;
#23910=VECTOR ( 'NONE', #10167, 1000.000000000000000 ) ;
#23911=CARTESIAN_POINT ( 'NONE',  ( 175.7287565553229456, -9.999999999999994671, -2.233642730705309720 ) ) ;
#23912=LINE ( 'NONE', #14715, #2536 ) ;
#23916=ORIENTED_EDGE ( 'NONE', *, *, #24026, .T. ) ;
#23918=EDGE_CURVE ( 'NONE', #2712, #14597, #3889, .T. ) ;
#23920=ADVANCED_FACE ( 'NONE', ( #1611 ), #27567, .T. ) ;
#23924=VECTOR ( 'NONE', #26802, 1000.000000000000000 ) ;
#23926=ORIENTED_EDGE ( 'NONE', *, *, #19314, .F. ) ;
#23927=DIRECTION ( 'NONE',  ( 0.5877852522924731371, 1.586114251531760728E-16, -0.8090169943749474513 ) ) ;
#23929=DIRECTION ( 'NONE',  ( 0.5877852522924731371, 1.586114251531760728E-16, -0.8090169943749474513 ) ) ;
#23931=LINE ( 'NONE', #19027, #20673 ) ;
#23932=PLANE ( 'NONE',  #14611 ) ;
#23937=DIRECTION ( 'NONE',  ( -2.698458740408365879E-16, 1.000000000000000000, 0.000000000000000000 ) ) ;
#23940=PLANE ( 'NONE',  #26611 ) ;
#23942=EDGE_LOOP ( 'NONE', ( #12938, #17527, #17542, #27014 ) ) ;
#23945=CARTESIAN_POINT ( 'NONE',  ( 137.0152310637606092, -4.999999999999980460, -24.27857615940569147 ) ) ;
#23946=CARTESIAN_POINT ( 'NONE',  ( 10.91913706431875930, -5.000000000000015099, 33.60564838301395696 ) ) ;
#23949=ORIENTED_EDGE ( 'NONE', *, *, #10478, .F. ) ;
#23951=ORIENTED_EDGE ( 'NONE', *, *, #5331, .T. ) ;
#23952=EDGE_CURVE ( 'NONE', #17919, #1754, #11045, .T. ) ;
#23954=EDGE_CURVE ( 'NONE', #17680, #4823, #20198, .T. ) ;
#23956=FACE_OUTER_BOUND ( 'NONE', #29757, .T. ) ;
#23957=LINE ( 'NONE', #3491, #2386 ) ;
#23958=EDGE_CURVE ( 'NONE', #27211, #13095, #4332, .T. ) ;
#23959=LINE ( 'NONE', #16765, #19096 ) ;
#23960=VERTEX_POINT ( 'NONE', #15623 ) ;
#23962=DIRECTION ( 'NONE',  ( -0.5877852522924731371, -1.586114251531760728E-16, -0.8090169943749474513 ) ) ;
#23964=VECTOR ( 'NONE', #7423, 1000.000000000000000 ) ;
#23966=CARTESIAN_POINT ( 'NONE',  ( 172.2287565553229172, -4.999999999999971578, -12.16987298107781434 ) ) ;
#23968=DIRECTION ( 'NONE',  ( -0.5877852522924731371, -1.586114251531760728E-16, -0.8090169943749474513 ) ) ;
#23972=DIRECTION ( 'NONE',  ( -2.698458740408365879E-16, 1.000000000000000000, 0.000000000000000000 ) ) ;
#23976=EDGE_LOOP ( 'NONE', ( #3514, #17588, #29102, #24893, #17123 ) ) ;
#23977=ORIENTED_EDGE ( 'NONE', *, *, #17817, .T. ) ;
#23981=LINE ( 'NONE', #28733, #7207 ) ;
#23982=ORIENTED_EDGE ( 'NONE', *, *, #897, .F. ) ;
#23984=ORIENTED_EDGE ( 'NONE', *, *, #25110, .T. ) ;
#23986=VERTEX_POINT ( 'NONE', #24956 ) ;
#23991=EDGE_CURVE ( 'NONE', #18805, #11448, #364, .T. ) ;
#23993=EDGE_CURVE ( 'NONE', #26875, #2818, #60, .T. ) ;
#23994=ADVANCED_FACE ( 'NONE', ( #9344 ), #2655, .T. ) ;
#23995=ADVANCED_FACE ( 'NONE', ( #12243 ), #18671, .T. ) ;
#24000=DIRECTION ( 'NONE',  ( 0.9510565162951535312, 2.566386769018988816E-16, -0.3090169943749475623 ) ) ;
#24001=FACE_BOUND ( 'NONE', #22423, .T. ) ;
#24002=VECTOR ( 'NONE', #22625, 999.9999999999998863 ) ;
#24003=DIRECTION ( 'NONE',  ( 0.5877852522924731371, 1.586114251531760728E-16, 0.8090169943749474513 ) ) ;
#24004=CARTESIAN_POINT ( 'NONE',  ( 171.1922820468853104, -1.999999999999970912, -13.59645775552055902 ) ) ;
#24006=PLANE ( 'NONE',  #24636 ) ;
#24009=CARTESIAN_POINT ( 'NONE',  ( 151.1922820468854525, -1.999999999999975353, -30.91696583120936026 ) ) ;
#24012=EDGE_LOOP ( 'NONE', ( #19651, #23599, #6587, #5440, #12463, #23096 ) ) ;
#24013=AXIS2_PLACEMENT_3D ( 'NONE', #9888, #4716, #23489 ) ;
#24015=FACE_OUTER_BOUND ( 'NONE', #7279, .T. ) ;
#24016=DIRECTION ( 'NONE',  ( -1.000000000000000000, -2.891205793294689173E-16, 0.000000000000000000 ) ) ;
#24017=CARTESIAN_POINT ( 'NONE',  ( 161.1922820468853104, -1.999999999999973577, -2.083034168790677043 ) ) ;
#24023=DIRECTION ( 'NONE',  ( 1.000000000000000000, 0.000000000000000000, 0.000000000000000000 ) ) ;
#24024=VECTOR ( 'NONE', #16840, 1000.000000000000000 ) ;
#24026=EDGE_CURVE ( 'NONE', #20158, #12496, #16223, .T. ) ;
#24028=ADVANCED_FACE ( 'NONE', ( #212 ), #14369, .T. ) ;
#24033=ORIENTED_EDGE ( 'NONE', *, *, #13930, .F. ) ;
#24034=FACE_OUTER_BOUND ( 'NONE', #27275, .T. ) ;
#24035=DIRECTION ( 'NONE',  ( 0.9510565162951536422, 0.000000000000000000, -0.3090169943749475623 ) ) ;
#24036=LINE ( 'NONE', #10120, #28640 ) ;
#24037=LINE ( 'NONE', #3137, #431 ) ;
#24039=AXIS2_PLACEMENT_3D ( 'NONE', #29939, #30083, #266 ) ;
#24045=VERTEX_POINT ( 'NONE', #9490 ) ;
#24047=CARTESIAN_POINT ( 'NONE',  ( 164.5152310637604387, -1.999999999999972689, -4.391296821672111328 ) ) ;
#24048=FACE_OUTER_BOUND ( 'NONE', #2996, .T. ) ;
#24050=DIRECTION ( 'NONE',  ( -0.8090169943749474513, -2.183098979609982436E-16, -0.5877852522924731371 ) ) ;
#24051=LINE ( 'NONE', #9837, #766 ) ;
#24053=ORIENTED_EDGE ( 'NONE', *, *, #23668, .F. ) ;
#24054=DIRECTION ( 'NONE',  ( 0.3090169943749475623, 8.338696094058001131E-17, 0.9510565162951536422 ) ) ;
#24056=PLANE ( 'NONE',  #8095 ) ;
#24057=FACE_OUTER_BOUND ( 'NONE', #16058, .T. ) ;
#24060=VERTEX_POINT ( 'NONE', #5230 ) ;
#24065=VECTOR ( 'NONE', #2986, 1000.000000000000000 ) ;
#24066=ORIENTED_EDGE ( 'NONE', *, *, #27482, .T. ) ;
#24067=CARTESIAN_POINT ( 'NONE',  ( 176.1922820468853104, -1.999999999999968914, -19.40354224447947828 ) ) ;
#24068=ORIENTED_EDGE ( 'NONE', *, *, #2644, .F. ) ;
#24069=PLANE ( 'NONE',  #963 ) ;
#24070=FACE_OUTER_BOUND ( 'NONE', #2409, .T. ) ;
#24071=CARTESIAN_POINT ( 'NONE',  ( 146.1922820468853956, -1.999999999999978018, -2.083034168790677043 ) ) ;
#24072=CARTESIAN_POINT ( 'NONE',  ( 173.6922820468852819, -9.999999999999996447, -9.266330736598359152 ) ) ;
#24073=ADVANCED_FACE ( 'NONE', ( #28172 ), #2965, .T. ) ;
#24076=EDGE_CURVE ( 'NONE', #18221, #506, #21253, .T. ) ;
#24077=VECTOR ( 'NONE', #25910, 1000.000000000000000 ) ;
#24078=FACE_OUTER_BOUND ( 'NONE', #1795, .T. ) ;
#24079=LINE ( 'NONE', #7586, #14868 ) ;
#24081=CARTESIAN_POINT ( 'NONE',  ( 137.0152310637606092, -4.999999999999980460, -15.61832212156129351 ) ) ;
#24082=DIRECTION ( 'NONE',  ( -0.9510565162951536422, -2.566386769018988816E-16, -0.3090169943749472292 ) ) ;
#24083=VERTEX_POINT ( 'NONE', #13921 ) ;
#24085=FACE_OUTER_BOUND ( 'NONE', #6546, .T. ) ;
#24086=ORIENTED_EDGE ( 'NONE', *, *, #28151, .F. ) ;
#24088=ORIENTED_EDGE ( 'NONE', *, *, #19270, .F. ) ;
#24089=ORIENTED_EDGE ( 'NONE', *, *, #17484, .F. ) ;
#24093=CARTESIAN_POINT ( 'NONE',  ( 149.7287565553230309, -1.999999999999975353, -25.16025403784440329 ) ) ;
#24095=DIRECTION ( 'NONE',  ( -0.8090169943749474513, -2.183098979609982436E-16, 0.5877852522924731371 ) ) ;
#24096=VECTOR ( 'NONE', #20080, 1000.000000000000000 ) ;
#24097=DIRECTION ( 'NONE',  ( 0.5877852522924731371, 0.000000000000000000, 0.8090169943749474513 ) ) ;
#24098=CARTESIAN_POINT ( 'NONE',  ( 142.0152310637606092, -1.999999999999978018, -24.27857615940569147 ) ) ;
#24099=CARTESIAN_POINT ( 'NONE',  ( 130.7287565553229456, -4.999999999999983125, 3.500000000000003109 ) ) ;
#24100=CARTESIAN_POINT ( 'NONE',  ( 134.5152310637605808, -10.00000000000000533, -2.627941064794695691 ) ) ;
#24101=CARTESIAN_POINT ( 'NONE',  ( 177.2287565553229172, -9.999999999999994671, -29.49038105676660493 ) ) ;
#24102=VECTOR ( 'NONE', #23693, 1000.000000000000000 ) ;
#24104=EDGE_CURVE ( 'NONE', #29971, #20355, #513, .T. ) ;
#24105=EDGE_CURVE ( 'NONE', #18619, #16899, #9650, .T. ) ;
#24107=ORIENTED_EDGE ( 'NONE', *, *, #28212, .T. ) ;
#24109=EDGE_CURVE ( 'NONE', #19416, #14794, #9945, .T. ) ;
#24113=FACE_BOUND ( 'NONE', #19970, .T. ) ;
#24114=ORIENTED_EDGE ( 'NONE', *, *, #18036, .F. ) ;
#24117=DIRECTION ( 'NONE',  ( 1.000000000000000000, 2.698458740408365879E-16, -1.110223024625156540E-16 ) ) ;
#24118=VECTOR ( 'NONE', #28499, 1000.000000000000000 ) ;
#24120=LINE ( 'NONE', #24419, #27216 ) ;
#24122=LINE ( 'NONE', #763, #30138 ) ;
#24123=ORIENTED_EDGE ( 'NONE', *, *, #12216, .T. ) ;
#24125=ORIENTED_EDGE ( 'NONE', *, *, #13892, .T. ) ;
#24129=CARTESIAN_POINT ( 'NONE',  ( 132.0152310637605524, -10.00000000000000711, -34.70218595412750773 ) ) ;
#24130=VERTEX_POINT ( 'NONE', #4781 ) ;
#24131=VERTEX_POINT ( 'NONE', #14072 ) ;
#24136=LINE ( 'NONE', #28758, #21247 ) ;
#24137=FACE_BOUND ( 'NONE', #26815, .T. ) ;
#24139=DIRECTION ( 'NONE',  ( 0.5877852522924731371, 0.000000000000000000, 0.8090169943749474513 ) ) ;
#24140=DIRECTION ( 'NONE',  ( -2.698458740408365879E-16, 1.000000000000000000, 0.000000000000000000 ) ) ;
#24143=LINE ( 'NONE', #9932, #26585 ) ;
#24146=DIRECTION ( 'NONE',  ( -0.9510565162951536422, 0.000000000000000000, -0.3090169943749472292 ) ) ;
#24149=DIRECTION ( 'NONE',  ( -0.9510565162951536422, 0.000000000000000000, -0.3090169943749472292 ) ) ;
#24150=ORIENTED_EDGE ( 'NONE', *, *, #13557, .F. ) ;
#24154=DIRECTION ( 'NONE',  ( 1.000000000000000000, 2.698458740408365879E-16, -1.110223024625156540E-16 ) ) ;
#24155=DIRECTION ( 'NONE',  ( -0.8090169943749474513, -2.183098979609982436E-16, 0.5877852522924731371 ) ) ;
#24156=ORIENTED_EDGE ( 'NONE', *, *, #5259, .T. ) ;
#24157=DIRECTION ( 'NONE',  ( 2.908569913943825061E-16, -1.000000000000000000, -6.826925868028081731E-18 ) ) ;
#24158=VERTEX_POINT ( 'NONE', #10095 ) ;
#24162=ORIENTED_EDGE ( 'NONE', *, *, #25412, .T. ) ;
#24163=EDGE_LOOP ( 'NONE', ( #8963, #7088, #7067, #5961, #13475 ) ) ;
#24164=VERTEX_POINT ( 'NONE', #12997 ) ;
#24166=DIRECTION ( 'NONE',  ( -0.8090169943749474513, -2.183098979609982436E-16, 0.5877852522924731371 ) ) ;
#24168=ORIENTED_EDGE ( 'NONE', *, *, #5777, .F. ) ;
#24169=CARTESIAN_POINT ( 'NONE',  ( 164.5152310637604671, -9.999999999999998224, -21.71180489736091346 ) ) ;
#24172=ORIENTED_EDGE ( 'NONE', *, *, #27170, .F. ) ;
#24174=DIRECTION ( 'NONE',  ( -0.5877852522924731371, 0.000000000000000000, 0.8090169943749474513 ) ) ;
#24175=VECTOR ( 'NONE', #11710, 1000.000000000000000 ) ;
#24176=DIRECTION ( 'NONE',  ( 0.3090169943749475623, 8.338696094058001131E-17, 0.9510565162951536422 ) ) ;
#24178=CARTESIAN_POINT ( 'NONE',  ( 161.1922820468853956, -4.999999999999974243, -30.91696583120936026 ) ) ;
#24179=AXIS2_PLACEMENT_3D ( 'NONE', #6622, #20796, #18209 ) ;
#24181=EDGE_CURVE ( 'NONE', #2025, #7643, #805, .T. ) ;
#24182=LINE ( 'NONE', #21878, #24118 ) ;
#24184=EDGE_CURVE ( 'NONE', #21114, #29571, #8260, .T. ) ;
#24186=EDGE_CURVE ( 'NONE', #28478, #10393, #19409, .T. ) ;
#24191=PLANE ( 'NONE',  #20762 ) ;
#24192=CARTESIAN_POINT ( 'NONE',  ( 147.2287565553230309, -10.00000000000000178, -29.49038105676660138 ) ) ;
#24193=CARTESIAN_POINT ( 'NONE',  ( 95.00630608762466522, -4.999999999999991118, 69.02612180135393771 ) ) ;
#24202=CARTESIAN_POINT ( 'NONE',  ( 164.5152310637604671, -9.999999999999998224, -21.71180489736091346 ) ) ;
#24206=ORIENTED_EDGE ( 'NONE', *, *, #4361, .F. ) ;
#24212=COLOUR_RGB ( '', 0.40784314, 0.44705882, 0.49803922) ;
#24213=ORIENTED_EDGE ( 'NONE', *, *, #8281, .F. ) ;
#24216=ORIENTED_EDGE ( 'NONE', *, *, #5333, .F. ) ;
#24219=DIRECTION ( 'NONE',  ( 0.000000000000000000, -1.000000000000000000, 0.000000000000000000 ) ) ;
#24220=DIRECTION ( 'NONE',  ( 8.163404592832029035E-16, 2.202861047501738386E-31, 1.000000000000000000 ) ) ;
#24221=FACE_OUTER_BOUND ( 'NONE', #1082, .T. ) ;
#24222=AXIS2_PLACEMENT_3D ( 'NONE', #975, #29400, #19715 ) ;
#24223=EDGE_CURVE ( 'NONE', #12383, #590, #17569, .T. ) ;
#24226=VECTOR ( 'NONE', #25810, 1000.000000000000000 ) ;
#24228=LINE ( 'NONE', #1036, #27887 ) ;
#24229=FACE_OUTER_BOUND ( 'NONE', #27173, .T. ) ;
#24232=CARTESIAN_POINT ( 'NONE',  ( 129.5152310637605524, -1.999999999999982236, -30.37205893520530964 ) ) ;
#24233=ORIENTED_EDGE ( 'NONE', *, *, #21229, .T. ) ;
#24235=DIRECTION ( 'NONE',  ( -2.698458740408365879E-16, 1.000000000000000000, 0.000000000000000000 ) ) ;
#24237=ORIENTED_EDGE ( 'NONE', *, *, #8693, .F. ) ;
#24238=EDGE_LOOP ( 'NONE', ( #5431, #24634, #25030, #22888 ) ) ;
#24243=FACE_OUTER_BOUND ( 'NONE', #3229, .T. ) ;
#24245=CARTESIAN_POINT ( 'NONE',  ( 159.7287565553229456, -4.999999999999974243, -16.50000000000000000 ) ) ;
#24246=EDGE_CURVE ( 'NONE', #2635, #26570, #22309, .T. ) ;
#24247=VECTOR ( 'NONE', #29436, 1000.000000000000000 ) ;
#24249=ORIENTED_EDGE ( 'NONE', *, *, #16387, .F. ) ;
#24250=LINE ( 'NONE', #19199, #9875 ) ;
#24251=DIRECTION ( 'NONE',  ( -2.698458740408365879E-16, 1.000000000000000000, 0.000000000000000000 ) ) ;
#24252=CARTESIAN_POINT ( 'NONE',  ( 137.0152310637606092, -10.00000000000000533, -32.93883019725009120 ) ) ;
#24253=VERTEX_POINT ( 'NONE', #1263 ) ;
#24254=LINE ( 'NONE', #21954, #20502 ) ;
#24255=CARTESIAN_POINT ( 'NONE',  ( 141.1922820468854525, -10.00000000000000533, -30.91696583120935671 ) ) ;
#24260=AXIS2_PLACEMENT_3D ( 'NONE', #23511, #9454, #12202 ) ;
#24263=FACE_BOUND ( 'NONE', #26100, .T. ) ;
#24266=DIRECTION ( 'NONE',  ( -0.8090169943749474513, -2.183098979609982436E-16, -0.5877852522924731371 ) ) ;
#24268=CARTESIAN_POINT ( 'NONE',  ( 132.0152310637605524, -4.999999999999982236, -17.38167787843870826 ) ) ;
#24269=VERTEX_POINT ( 'NONE', #5690 ) ;
#24273=EDGE_LOOP ( 'NONE', ( #477, #15278, #17872, #12433 ) ) ;
#24276=CARTESIAN_POINT ( 'NONE',  ( 169.5152310637604955, -1.999999999999970024, -30.37205893520531319 ) ) ;
#24277=ORIENTED_EDGE ( 'NONE', *, *, #3570, .F. ) ;
#24278=PLANE ( 'NONE',  #16175 ) ;
#24280=EDGE_CURVE ( 'NONE', #28906, #18615, #26923, .T. ) ;
#24281=ORIENTED_EDGE ( 'NONE', *, *, #25110, .F. ) ;
#24286=CARTESIAN_POINT ( 'NONE',  ( 130.7287565553229456, -4.999999999999983125, -10.89389676854976408 ) ) ;
#24287=AXIS2_PLACEMENT_3D ( 'NONE', #23637, #16155, #4565 ) ;
#24288=DIRECTION ( 'NONE',  ( 0.5877852522924731371, 0.000000000000000000, 0.8090169943749474513 ) ) ;
#24289=LINE ( 'NONE', #5671, #5291 ) ;
#24290=LINE ( 'NONE', #15108, #6794 ) ;
#24294=DIRECTION ( 'NONE',  ( -2.698458740408365879E-16, 1.000000000000000000, 0.000000000000000000 ) ) ;
#24295=ORIENTED_EDGE ( 'NONE', *, *, #19958, .F. ) ;
#24297=VERTEX_POINT ( 'NONE', #12692 ) ;
#24302=CARTESIAN_POINT ( 'NONE',  ( 169.5152310637604671, -4.999999999999971578, -21.71180489736091346 ) ) ;
#24303=EDGE_LOOP ( 'NONE', ( #6, #5986, #23300, #13397, #24496 ) ) ;
#24304=DIRECTION ( 'NONE',  ( 0.5877852522924731371, 1.586114251531760728E-16, -0.8090169943749474513 ) ) ;
#24305=VERTEX_POINT ( 'NONE', #24017 ) ;
#24307=VECTOR ( 'NONE', #233, 1000.000000000000000 ) ;
#24311=ORIENTED_EDGE ( 'NONE', *, *, #4124, .F. ) ;
#24312=CARTESIAN_POINT ( 'NONE',  ( 174.5152310637604955, -4.999999999999969802, -28.60870317832789667 ) ) ;
#24315=AXIS2_PLACEMENT_3D ( 'NONE', #10938, #15521, #27018 ) ;
#24316=DIRECTION ( 'NONE',  ( 1.000000000000000000, 2.698458740408365879E-16, -1.110223024625156540E-16 ) ) ;
#24318=EDGE_CURVE ( 'NONE', #28540, #29884, #10399, .T. ) ;
#24320=ADVANCED_FACE ( 'NONE', ( #26304 ), #19706, .T. ) ;
#24323=ADVANCED_FACE ( 'NONE', ( #12389 ), #3261, .T. ) ;
#24324=ORIENTED_EDGE ( 'NONE', *, *, #5368, .T. ) ;
#24325=CARTESIAN_POINT ( 'NONE',  ( 138.6922820468854525, -10.00000000000000533, -23.73366926340167282 ) ) ;
#24326=CARTESIAN_POINT ( 'NONE',  ( 178.7287565553229172, -1.999999999999968914, -33.50000000000000000 ) ) ;
#24328=VECTOR ( 'NONE', #6606, 1000.000000000000000 ) ;
#24329=CARTESIAN_POINT ( 'NONE',  ( 148.6922820468853956, -10.00000000000000178, -9.266330736598359152 ) ) ;
#24330=LINE ( 'NONE', #3423, #14348 ) ;
#24335=LINE ( 'NONE', #7993, #800 ) ;
#24336=LINE ( 'NONE', #26336, #6764 ) ;
#24338=LINE ( 'NONE', #26491, #21460 ) ;
#24341=ORIENTED_EDGE ( 'NONE', *, *, #27136, .F. ) ;
#24345=DIRECTION ( 'NONE',  ( 1.000000000000000000, 2.908569913943825554E-16, -6.938893903907227392E-16 ) ) ;
#24346=VECTOR ( 'NONE', #27564, 999.9999999999998863 ) ;
#24351=CARTESIAN_POINT ( 'NONE',  ( 132.0152310637605808, -1.999999999999981348, -15.61832212156129351 ) ) ;
#24356=ADVANCED_FACE ( 'NONE', ( #26456 ), #24454, .T. ) ;
#24357=EDGE_CURVE ( 'NONE', #4081, #28996, #14821, .T. ) ;
#24360=EDGE_CURVE ( 'NONE', #30087, #11783, #23072, .T. ) ;
#24361=ORIENTED_EDGE ( 'NONE', *, *, #11864, .F. ) ;
#24363=FACE_OUTER_BOUND ( 'NONE', #22967, .T. ) ;
#24365=CARTESIAN_POINT ( 'NONE',  ( 127.7287565553229740, -1.999999999999982681, 0.5000000000000397460 ) ) ;
#24366=CARTESIAN_POINT ( 'NONE',  ( 176.1922820468853388, -9.999999999999994671, -28.06379628232387802 ) ) ;
#24367=DIRECTION ( 'NONE',  ( -0.8090169943749474513, -2.183098979609982436E-16, -0.5877852522924731371 ) ) ;
#24370=CONICAL_SURFACE ( 'NONE', #28822, 5.999999999999983125, 0.7853981633974496113 ) ;
#24372=VECTOR ( 'NONE', #29722, 1000.000000000000000 ) ;
#24377=ORIENTED_EDGE ( 'NONE', *, *, #16690, .T. ) ;
#24378=CARTESIAN_POINT ( 'NONE',  ( 17.51600279482502742, -5.000000000000013323, -53.90871343874875521 ) ) ;
#24380=CARTESIAN_POINT ( 'NONE',  ( 133.6922820468853956, -1.999999999999980904, -23.73366926340167282 ) ) ;
#24381=LINE ( 'NONE', #1191, #3457 ) ;
#24382=CARTESIAN_POINT ( 'NONE',  ( 147.0152310637605808, -4.999999999999977796, -34.70218595412750773 ) ) ;
#24383=ORIENTED_EDGE ( 'NONE', *, *, #27824, .T. ) ;
#24384=ORIENTED_EDGE ( 'NONE', *, *, #25877, .F. ) ;
#24388=AXIS2_PLACEMENT_3D ( 'NONE', #3884, #29731, #8739 ) ;
#24389=EDGE_CURVE ( 'NONE', #28330, #2176, #2026, .T. ) ;
#24392=FACE_OUTER_BOUND ( 'NONE', #29851, .T. ) ;
#24393=DIRECTION ( 'NONE',  ( -1.110223024625156540E-16, 0.000000000000000000, -1.000000000000000000 ) ) ;
#24394=LINE ( 'NONE', #733, #133 ) ;
#24396=VECTOR ( 'NONE', #4998, 1000.000000000000000 ) ;
#24397=ORIENTED_EDGE ( 'NONE', *, *, #12763, .F. ) ;
#24398=CARTESIAN_POINT ( 'NONE',  ( 142.0152310637606092, -4.999999999999978684, -15.61832212156129707 ) ) ;
#24401=VERTEX_POINT ( 'NONE', #8558 ) ;
#24403=DIRECTION ( 'NONE',  ( -2.698458740408365879E-16, 1.000000000000000000, 0.000000000000000000 ) ) ;
#24405=VECTOR ( 'NONE', #6217, 1000.000000000000000 ) ;
#24408=VERTEX_POINT ( 'NONE', #8858 ) ;
#24409=VECTOR ( 'NONE', #13139, 1000.000000000000000 ) ;
#24413=FACE_BOUND ( 'NONE', #29790, .T. ) ;
#24414=EDGE_CURVE ( 'NONE', #17911, #10566, #25208, .T. ) ;
#24416=ORIENTED_EDGE ( 'NONE', *, *, #24527, .T. ) ;
#24419=CARTESIAN_POINT ( 'NONE',  ( 177.2287565553228319, -9.999999999999994671, -3.509618943233403510 ) ) ;
#24420=ORIENTED_EDGE ( 'NONE', *, *, #819, .T. ) ;
#24421=FACE_OUTER_BOUND ( 'NONE', #18650, .T. ) ;
#24422=VERTEX_POINT ( 'NONE', #11306 ) ;
#24424=ORIENTED_EDGE ( 'NONE', *, *, #23877, .F. ) ;
#24427=CARTESIAN_POINT ( 'NONE',  ( 132.0152310637605808, -1.999999999999981348, 1.702185954127501066 ) ) ;
#24432=EDGE_LOOP ( 'NONE', ( #19849, #20234, #16536, #26767 ) ) ;
#24433=VECTOR ( 'NONE', #4078, 1000.000000000000000 ) ;
#24435=PLANE ( 'NONE',  #3723 ) ;
#24436=FACE_BOUND ( 'NONE', #18670, .T. ) ;
#24437=CARTESIAN_POINT ( 'NONE',  ( 171.1922820468853104, -9.999999999999996447, -13.59645775552055902 ) ) ;
#24439=DIRECTION ( 'NONE',  ( 1.000000000000000000, 0.000000000000000000, -0.000000000000000000 ) ) ;
#24441=DIRECTION ( 'NONE',  ( -2.698458740408365879E-16, 1.000000000000000000, 0.000000000000000000 ) ) ;
#24443=DIRECTION ( 'NONE',  ( 0.3090169943749472292, 8.338696094057992503E-17, -0.9510565162951536422 ) ) ;
#24445=PLANE ( 'NONE',  #22766 ) ;
#24446=ORIENTED_EDGE ( 'NONE', *, *, #28068, .F. ) ;
#24447=AXIS2_PLACEMENT_3D ( 'NONE', #10283, #1003, #5724 ) ;
#24449=EDGE_LOOP ( 'NONE', ( #6291, #5932, #28819, #10553 ) ) ;
#24452=LINE ( 'NONE', #29220, #2313 ) ;
#24453=ORIENTED_EDGE ( 'NONE', *, *, #5894, .F. ) ;
#24454=PLANE ( 'NONE',  #26662 ) ;
#24459=EDGE_LOOP ( 'NONE', ( #20947, #23194, #1153, #30158 ) ) ;
#24460=VERTEX_POINT ( 'NONE', #22471 ) ;
#24461=CARTESIAN_POINT ( 'NONE',  ( 139.7287565553230309, -1.999999999999978684, -16.50000000000000000 ) ) ;
#24463=VERTEX_POINT ( 'NONE', #4299 ) ;
#24464=LINE ( 'NONE', #26938, #26169 ) ;
#24466=EDGE_CURVE ( 'NONE', #1114, #9138, #10848, .T. ) ;
#24469=ORIENTED_EDGE ( 'NONE', *, *, #15853, .T. ) ;
#24470=ORIENTED_EDGE ( 'NONE', *, *, #4408, .F. ) ;
#24471=VECTOR ( 'NONE', #4481, 1000.000000000000000 ) ;
#24473=DIRECTION ( 'NONE',  ( 0.5877852522924731371, 1.586114251531760728E-16, 0.8090169943749474513 ) ) ;
#24475=LINE ( 'NONE', #3572, #7648 ) ;
#24478=ORIENTED_EDGE ( 'NONE', *, *, #16137, .F. ) ;
#24482=ADVANCED_FACE ( 'NONE', ( #20157 ), #20609, .T. ) ;
#24483=ADVANCED_FACE ( 'NONE', ( #22616 ), #6588, .T. ) ;
#24484=VERTEX_POINT ( 'NONE', #29996 ) ;
#24485=PLANE ( 'NONE',  #20285 ) ;
#24486=DIRECTION ( 'NONE',  ( 0.5877852522924731371, 1.586114251531760728E-16, -0.8090169943749474513 ) ) ;
#24488=LINE ( 'NONE', #19444, #12261 ) ;
#24490=VECTOR ( 'NONE', #9319, 1000.000000000000000 ) ;
#24491=CARTESIAN_POINT ( 'NONE',  ( 157.0152310637604671, -1.999999999999974909, 1.702185954127501066 ) ) ;
#24492=LINE ( 'NONE', #8447, #9314 ) ;
#24493=EDGE_CURVE ( 'NONE', #21438, #436, #13440, .T. ) ;
#24495=ORIENTED_EDGE ( 'NONE', *, *, #9998, .T. ) ;
#24496=ORIENTED_EDGE ( 'NONE', *, *, #14435, .T. ) ;
#24497=CARTESIAN_POINT ( 'NONE',  ( 141.1922820468854525, -4.999999999999980460, -13.59645775552055902 ) ) ;
#24500=PLANE ( 'NONE',  #17357 ) ;
#24501=FACE_OUTER_BOUND ( 'NONE', #4483, .T. ) ;
#24504=CARTESIAN_POINT ( 'NONE',  ( 171.1922820468852819, -4.999999999999971578, -4.936203717676158398 ) ) ;
#24506=ORIENTED_EDGE ( 'NONE', *, *, #20963, .T. ) ;
#24511=CARTESIAN_POINT ( 'NONE',  ( 139.5152310637606092, -1.999999999999978684, -11.28819510263909542 ) ) ;
#24512=VECTOR ( 'NONE', #4088, 1000.000000000000000 ) ;
#24513=CARTESIAN_POINT ( 'NONE',  ( 132.2287565553230024, -10.00000000000000888, -12.16987298107780013 ) ) ;
#24514=ORIENTED_EDGE ( 'NONE', *, *, #3135, .F. ) ;
#24517=DIRECTION ( 'NONE',  ( -0.8090169943749474513, -2.183098979609982436E-16, -0.5877852522924731371 ) ) ;
#24524=EDGE_CURVE ( 'NONE', #5689, #7473, #25357, .T. ) ;
#24525=CARTESIAN_POINT ( 'NONE',  ( 146.1922820468854241, -1.999999999999978018, -19.40354224447947828 ) ) ;
#24526=LINE ( 'NONE', #29302, #30065 ) ;
#24527=EDGE_CURVE ( 'NONE', #16899, #1878, #11001, .T. ) ;
#24528=EDGE_CURVE ( 'NONE', #3207, #17958, #8708, .T. ) ;
#24530=LINE ( 'NONE', #3621, #23910 ) ;
#24531=EDGE_CURVE ( 'NONE', #23037, #15699, #13744, .T. ) ;
#24532=DIRECTION ( 'NONE',  ( -2.698458740408365879E-16, 1.000000000000000000, 0.000000000000000000 ) ) ;
#24534=DIRECTION ( 'NONE',  ( -1.110223024625156540E-16, 0.000000000000000000, -1.000000000000000000 ) ) ;
#24540=ORIENTED_EDGE ( 'NONE', *, *, #6407, .F. ) ;
#24545=DIRECTION ( 'NONE',  ( 1.110223024625156540E-16, 2.995891024602366092E-32, 1.000000000000000000 ) ) ;
#24546=CARTESIAN_POINT ( 'NONE',  ( 173.6922820468853104, -4.999999999999969802, -17.92658477444275889 ) ) ;
#24547=DIRECTION ( 'NONE',  ( -0.8090169943749474513, -2.183098979609982436E-16, 0.5877852522924731371 ) ) ;
#24548=VERTEX_POINT ( 'NONE', #11447 ) ;
#24549=CARTESIAN_POINT ( 'NONE',  ( 6.783682487892742863, -5.000000000000015987, 20.87802791441155037 ) ) ;
#24550=FACE_OUTER_BOUND ( 'NONE', #4540, .T. ) ;
#24552=DIRECTION ( 'NONE',  ( -0.9510565162951536422, 0.000000000000000000, -0.3090169943749472292 ) ) ;
#24553=FACE_OUTER_BOUND ( 'NONE', #11618, .T. ) ;
#24557=EDGE_LOOP ( 'NONE', ( #25260, #19169, #8463, #27127 ) ) ;
#24559=ORIENTED_EDGE ( 'NONE', *, *, #17484, .T. ) ;
#24560=EDGE_CURVE ( 'NONE', #22451, #21981, #29386, .T. ) ;
#24561=EDGE_CURVE ( 'NONE', #4559, #19382, #29695, .T. ) ;
#24565=FACE_BOUND ( 'NONE', #12794, .T. ) ;
#24566=ADVANCED_FACE ( 'NONE', ( #27835 ), #7342, .T. ) ;
#24567=VERTEX_POINT ( 'NONE', #16641 ) ;
#24568=EDGE_LOOP ( 'NONE', ( #6599, #24384, #11889, #9137 ) ) ;
#24569=EDGE_LOOP ( 'NONE', ( #15527, #26410, #2469, #1722, #10094 ) ) ;
#24570=DIRECTION ( 'NONE',  ( 1.000000000000000000, 2.891205793294675861E-16, 0.000000000000000000 ) ) ;
#24572=DIRECTION ( 'NONE',  ( -2.698458740408365879E-16, 1.000000000000000000, 0.000000000000000000 ) ) ;
#24573=ORIENTED_EDGE ( 'NONE', *, *, #13725, .T. ) ;
#24574=LINE ( 'NONE', #28896, #23264 ) ;
#24575=ORIENTED_EDGE ( 'NONE', *, *, #9051, .T. ) ;
#24577=ORIENTED_EDGE ( 'NONE', *, *, #18422, .T. ) ;
#24581=VECTOR ( 'NONE', #27813, 1000.000000000000000 ) ;
#24585=CARTESIAN_POINT ( 'NONE',  ( 1.244173783436457737E-15, -5.000000000000017764, 0.000000000000000000 ) ) ;
#24586=ORIENTED_EDGE ( 'NONE', *, *, #27585, .T. ) ;
#24587=LINE ( 'NONE', #3679, #22924 ) ;
#24590=ORIENTED_EDGE ( 'NONE', *, *, #20622, .T. ) ;
#24591=CARTESIAN_POINT ( 'NONE',  ( 164.5152310637604955, -9.999999999999996447, -30.37205893520531319 ) ) ;
#24596=DIRECTION ( 'NONE',  ( -0.9510565162951536422, 0.000000000000000000, -0.3090169943749472292 ) ) ;
#24597=ORIENTED_EDGE ( 'NONE', *, *, #24104, .F. ) ;
#24598=FACE_OUTER_BOUND ( 'NONE', #13873, .T. ) ;
#24599=VERTEX_POINT ( 'NONE', #6898 ) ;
#24601=DIRECTION ( 'NONE',  ( -2.698458740408365879E-16, 1.000000000000000000, 0.000000000000000000 ) ) ;
#24602=LINE ( 'NONE', #12689, #17871 ) ;
#24603=ORIENTED_EDGE ( 'NONE', *, *, #22760, .T. ) ;
#24605=ORIENTED_EDGE ( 'NONE', *, *, #19745, .F. ) ;
#24609=VERTEX_POINT ( 'NONE', #11752 ) ;
#24610=ORIENTED_EDGE ( 'NONE', *, *, #25974, .F. ) ;
#24611=DIRECTION ( 'NONE',  ( 1.110223024625156540E-16, 2.995891024602366092E-32, 1.000000000000000000 ) ) ;
#24617=VECTOR ( 'NONE', #28352, 1000.000000000000000 ) ;
#24618=ORIENTED_EDGE ( 'NONE', *, *, #9842, .T. ) ;
#24620=ADVANCED_FACE ( 'NONE', ( #16486 ), #21070, .T. ) ;
#24621=PLANE ( 'NONE',  #21553 ) ;
#24622=LINE ( 'NONE', #8432, #12146 ) ;
#24623=PLANE ( 'NONE',  #12328 ) ;
#24624=VECTOR ( 'NONE', #23937, 1000.000000000000000 ) ;
#24625=DIRECTION ( 'NONE',  ( 0.3090169943749472292, 8.338696094057992503E-17, -0.9510565162951536422 ) ) ;
#24626=DIRECTION ( 'NONE',  ( -0.5877852522924731371, 0.000000000000000000, 0.8090169943749474513 ) ) ;
#24627=CARTESIAN_POINT ( 'NONE',  ( 137.2287565553230309, -10.00000000000000533, -20.83012701892220164 ) ) ;
#24631=ORIENTED_EDGE ( 'NONE', *, *, #1723, .T. ) ;
#24632=CARTESIAN_POINT ( 'NONE',  ( 162.0152310637605240, -4.999999999999974243, -34.70218595412750773 ) ) ;
#24633=PLANE ( 'NONE',  #10170 ) ;
#24634=ORIENTED_EDGE ( 'NONE', *, *, #14855, .F. ) ;
#24636=AXIS2_PLACEMENT_3D ( 'NONE', #12523, #947, #28600 ) ;
#24637=PLANE ( 'NONE',  #24388 ) ;
#24638=LINE ( 'NONE', #7855, #29317 ) ;
#24640=VERTEX_POINT ( 'NONE', #2771 ) ;
#24641=ORIENTED_EDGE ( 'NONE', *, *, #12336, .F. ) ;
#24645=CARTESIAN_POINT ( 'NONE',  ( 133.6922820468854241, -10.00000000000000711, -0.6060766987539614181 ) ) ;
#24646=ORIENTED_EDGE ( 'NONE', *, *, #6440, .F. ) ;
#24650=VERTEX_POINT ( 'NONE', #16789 ) ;
#24652=VECTOR ( 'NONE', #2842, 1000.000000000000000 ) ;
#24656=VECTOR ( 'NONE', #18279, 1000.000000000000000 ) ;
#24657=VERTEX_POINT ( 'NONE', #28433 ) ;
#24660=ADVANCED_FACE ( 'NONE', ( #23212 ), #9764, .T. ) ;
#24661=CARTESIAN_POINT ( 'NONE',  ( 163.6922820468853956, -9.999999999999998224, -32.39392330124607611 ) ) ;
#24662=VECTOR ( 'NONE', #2281, 1000.000000000000000 ) ;
#24666=CARTESIAN_POINT ( 'NONE',  ( 138.6922820468854525, -10.00000000000000533, -26.58683881228715506 ) ) ;
#24668=DIRECTION ( 'NONE',  ( -0.9510565162951536422, -2.566386769018988323E-16, 0.3090169943749475623 ) ) ;
#24671=CARTESIAN_POINT ( 'NONE',  ( 167.0152310637604103, -1.999999999999972244, -0.06116980274991495881 ) ) ;
#24676=DIRECTION ( 'NONE',  ( -0.5877852522924731371, -1.586114251531760235E-16, 0.8090169943749474513 ) ) ;
#24678=VECTOR ( 'NONE', #21602, 1000.000000000000000 ) ;
#24679=CARTESIAN_POINT ( 'NONE',  ( 134.5152310637605524, -10.00000000000000533, -4.391296821672111328 ) ) ;
#24680=DIRECTION ( 'NONE',  ( 0.5877852522924731371, 1.586114251531760728E-16, -0.8090169943749474513 ) ) ;
#24682=CARTESIAN_POINT ( 'NONE',  ( 168.6922820468853388, -4.999999999999971578, -15.07341522555727664 ) ) ;
#24683=CARTESIAN_POINT ( 'NONE',  ( 137.0152310637605808, -1.999999999999979572, -26.04193191628310800 ) ) ;
#24685=ORIENTED_EDGE ( 'NONE', *, *, #19958, .T. ) ;
#24687=CARTESIAN_POINT ( 'NONE',  ( 147.0152310637605808, -10.00000000000000178, -34.70218595412750773 ) ) ;
#24688=CARTESIAN_POINT ( 'NONE',  ( 173.6922820468852535, -1.999999999999970912, -0.6060766987539614181 ) ) ;
#24689=ORIENTED_EDGE ( 'NONE', *, *, #19814, .F. ) ;
#24690=VECTOR ( 'NONE', #17107, 1000.000000000000000 ) ;
#24691=CARTESIAN_POINT ( 'NONE',  ( 163.6922820468853104, -9.999999999999998224, -6.413161187712876909 ) ) ;
#24697=DIRECTION ( 'NONE',  ( -0.5877852522924731371, -1.586114251531760728E-16, -0.8090169943749474513 ) ) ;
#24698=DIRECTION ( 'NONE',  ( -0.5877852522924731371, -1.586114251531760728E-16, -0.8090169943749474513 ) ) ;
#24701=EDGE_CURVE ( 'NONE', #2206, #11734, #26116, .T. ) ;
#24702=EDGE_CURVE ( 'NONE', #16032, #4875, #7042, .T. ) ;
#24704=EDGE_LOOP ( 'NONE', ( #6066, #23621, #30061, #16273, #573 ) ) ;
#24705=EDGE_CURVE ( 'NONE', #29509, #9780, #23362, .T. ) ;
#24706=LINE ( 'NONE', #6233, #17204 ) ;
#24708=AXIS2_PLACEMENT_3D ( 'NONE', #2809, #14222, #25852 ) ;
#24709=DIRECTION ( 'NONE',  ( -0.5877852522924731371, 0.000000000000000000, 0.8090169943749474513 ) ) ;
#24710=VECTOR ( 'NONE', #16513, 1000.000000000000000 ) ;
#24714=ORIENTED_EDGE ( 'NONE', *, *, #14740, .F. ) ;
#24717=ORIENTED_EDGE ( 'NONE', *, *, #9581, .T. ) ;
#24720=FACE_BOUND ( 'NONE', #27843, .T. ) ;
#24721=EDGE_LOOP ( 'NONE', ( #26193, #7537, #7836, #10570, #11543 ) ) ;
#24722=VERTEX_POINT ( 'NONE', #21214 ) ;
#24723=CARTESIAN_POINT ( 'NONE',  ( 158.6922820468854241, -9.999999999999998224, -32.39392330124607611 ) ) ;
#24726=PLANE ( 'NONE',  #26717 ) ;
#24727=CARTESIAN_POINT ( 'NONE',  ( 156.1922820468854241, -10.00000000000000000, -30.91696583120936026 ) ) ;
#24728=ORIENTED_EDGE ( 'NONE', *, *, #3856, .F. ) ;
#24730=EDGE_LOOP ( 'NONE', ( #11849, #15113, #17278, #15567 ) ) ;
#24733=DIRECTION ( 'NONE',  ( -0.8090169943749474513, -2.183098979609982436E-16, -0.5877852522924731371 ) ) ;
#24734=ORIENTED_EDGE ( 'NONE', *, *, #308, .T. ) ;
#24738=EDGE_CURVE ( 'NONE', #9138, #2080, #28287, .T. ) ;
#24739=ADVANCED_FACE ( 'NONE', ( #5652 ), #14636, .T. ) ;
#24740=EDGE_CURVE ( 'NONE', #19636, #3882, #12654, .T. ) ;
#24741=DIRECTION ( 'NONE',  ( 1.110223024625156540E-16, 2.995891024602366092E-32, 1.000000000000000000 ) ) ;
#24743=FACE_OUTER_BOUND ( 'NONE', #28022, .T. ) ;
#24744=AXIS2_PLACEMENT_3D ( 'NONE', #7483, #18929, #28284 ) ;
#24745=ORIENTED_EDGE ( 'NONE', *, *, #11789, .F. ) ;
#24746=CARTESIAN_POINT ( 'NONE',  ( 168.6922820468853104, -9.999999999999998224, -9.266330736598359152 ) ) ;
#24748=CARTESIAN_POINT ( 'NONE',  ( 141.1922820468854525, -1.999999999999978462, -10.74328820663507678 ) ) ;
#24749=VECTOR ( 'NONE', #5159, 1000.000000000000000 ) ;
#24751=PLANE ( 'NONE',  #8047 ) ;
#24755=DIRECTION ( 'NONE',  ( 0.3090169943749472292, 8.338696094057992503E-17, -0.9510565162951536422 ) ) ;
#24757=CARTESIAN_POINT ( 'NONE',  ( 142.0152310637606092, -10.00000000000000355, -24.27857615940569147 ) ) ;
#24758=ORIENTED_EDGE ( 'NONE', *, *, #15787, .F. ) ;
#24760=LINE ( 'NONE', #3846, #24409 ) ;
#24761=CARTESIAN_POINT ( 'NONE',  ( 142.2287565553230309, -10.00000000000000533, -29.49038105676660138 ) ) ;
#24767=VERTEX_POINT ( 'NONE', #28577 ) ;
#24768=AXIS2_PLACEMENT_3D ( 'NONE', #2618, #8592, #24949 ) ;
#24769=CARTESIAN_POINT ( 'NONE',  ( 139.5152310637606092, -4.999999999999980460, -11.28819510263909542 ) ) ;
#24770=PLANE ( 'NONE',  #6296 ) ;
#24771=CARTESIAN_POINT ( 'NONE',  ( 134.7287565553230024, -1.999999999999980460, -7.839745962155602044 ) ) ;
#24775=EDGE_CURVE ( 'NONE', #4875, #14798, #21973, .T. ) ;
#24777=ORIENTED_EDGE ( 'NONE', *, *, #21004, .F. ) ;
#24779=DIRECTION ( 'NONE',  ( 0.5877852522924731371, 1.586114251531760728E-16, -0.8090169943749474513 ) ) ;
#24780=LINE ( 'NONE', #13166, #6039 ) ;
#24781=CARTESIAN_POINT ( 'NONE',  ( 161.1922820468853104, -10.00000000000000000, -4.936203717676158398 ) ) ;
#24782=PLANE ( 'NONE',  #13092 ) ;
#24784=VECTOR ( 'NONE', #12200, 1000.000000000000000 ) ;
#24787=CARTESIAN_POINT ( 'NONE',  ( 148.6922820468854241, -1.999999999999977129, -15.07341522555727664 ) ) ;
#24789=LINE ( 'NONE', #3880, #6641 ) ;
#24795=CARTESIAN_POINT ( 'NONE',  ( 174.5152310637604103, -9.999999999999994671, -13.05155085951651195 ) ) ;
#24797=VECTOR ( 'NONE', #19344, 999.9999999999998863 ) ;
#24798=ORIENTED_EDGE ( 'NONE', *, *, #2447, .T. ) ;
#24799=PLANE ( 'NONE',  #24179 ) ;
#24801=EDGE_CURVE ( 'NONE', #7028, #11745, #24122, .T. ) ;
#24802=VECTOR ( 'NONE', #20665, 1000.000000000000000 ) ;
#24803=LINE ( 'NONE', #5732, #13934 ) ;
#24804=DIRECTION ( 'NONE',  ( 0.9510565162951536422, 0.000000000000000000, -0.3090169943749475623 ) ) ;
#24805=ORIENTED_EDGE ( 'NONE', *, *, #12756, .F. ) ;
#24808=CARTESIAN_POINT ( 'NONE',  ( 153.6922820468853672, -4.999999999999976019, -9.266330736598359152 ) ) ;
#24810=ORIENTED_EDGE ( 'NONE', *, *, #16305, .F. ) ;
#24811=DIRECTION ( 'NONE',  ( -0.5877852522924731371, -1.586114251531760235E-16, 0.8090169943749474513 ) ) ;
#24814=EDGE_CURVE ( 'NONE', #6532, #25128, #26889, .T. ) ;
#24815=ORIENTED_EDGE ( 'NONE', *, *, #8799, .F. ) ;
#24817=AXIS2_PLACEMENT_3D ( 'NONE', #28949, #10728, #22177 ) ;
#24819=AXIS2_PLACEMENT_3D ( 'NONE', #10282, #26490, #5723 ) ;
#24821=DIRECTION ( 'NONE',  ( -2.698458740408365879E-16, 1.000000000000000000, 0.000000000000000000 ) ) ;
#24822=DIRECTION ( 'NONE',  ( 0.5877852522924731371, 1.586114251531760728E-16, 0.8090169943749474513 ) ) ;
#24823=CARTESIAN_POINT ( 'NONE',  ( 87.72563772519548309, -4.999999999999993783, 63.73640660374597644 ) ) ;
#24830=LINE ( 'NONE', #8924, #8809 ) ;
#24831=DIRECTION ( 'NONE',  ( -0.8090169943749474513, -2.183098979609982436E-16, -0.5877852522924731371 ) ) ;
#24834=LINE ( 'NONE', #3925, #778 ) ;
#24836=EDGE_CURVE ( 'NONE', #968, #12496, #29187, .T. ) ;
#24837=ORIENTED_EDGE ( 'NONE', *, *, #2938, .T. ) ;
#24838=CONICAL_SURFACE ( 'NONE', #11650, 5.999999999999977796, 0.7853981633974509435 ) ;
#24840=LINE ( 'NONE', #23000, #14147 ) ;
#24841=EDGE_CURVE ( 'NONE', #21691, #24463, #14459, .T. ) ;
#24842=PLANE ( 'NONE',  #29834 ) ;
#24845=EDGE_LOOP ( 'NONE', ( #5781, #1568, #24237, #4847 ) ) ;
#24848=ORIENTED_EDGE ( 'NONE', *, *, #15853, .F. ) ;
#24851=PLANE ( 'NONE',  #17968 ) ;
#24852=CARTESIAN_POINT ( 'NONE',  ( 163.6922820468853956, -9.999999999999998224, -35.24709285013155835 ) ) ;
#24855=ORIENTED_EDGE ( 'NONE', *, *, #8952, .F. ) ;
#24856=LINE ( 'NONE', #1817, #4054 ) ;
#24858=VECTOR ( 'NONE', #25053, 1000.000000000000000 ) ;
#24859=ORIENTED_EDGE ( 'NONE', *, *, #28381, .F. ) ;
#24861=CARTESIAN_POINT ( 'NONE',  ( 141.1922820468854525, -4.999999999999980460, -22.25671179336495697 ) ) ;
#24862=CARTESIAN_POINT ( 'NONE',  ( 152.0152310637604955, -10.00000000000000178, -15.61832212156129351 ) ) ;
#24863=VECTOR ( 'NONE', #28076, 1000.000000000000000 ) ;
#24864=AXIS2_PLACEMENT_3D ( 'NONE', #28838, #12899, #7727 ) ;
#24867=EDGE_LOOP ( 'NONE', ( #29346, #29547, #1145, #27608, #22119 ) ) ;
#24869=ORIENTED_EDGE ( 'NONE', *, *, #17332, .F. ) ;
#24872=CARTESIAN_POINT ( 'NONE',  ( 127.7287565553229598, -1.999999999999982681, -33.50000000000000000 ) ) ;
#24873=ADVANCED_FACE ( 'NONE', ( #24421 ), #12497, .T. ) ;
#24874=ORIENTED_EDGE ( 'NONE', *, *, #10380, .F. ) ;
#24875=DIRECTION ( 'NONE',  ( -0.8090169943749474513, -2.183098979609982436E-16, 0.5877852522924731371 ) ) ;
#24876=VERTEX_POINT ( 'NONE', #7631 ) ;
#24877=ADVANCED_FACE ( 'NONE', ( #19525 ), #5954, .T. ) ;
#24880=EDGE_CURVE ( 'NONE', #13256, #9641, #26268, .T. ) ;
#24881=DIRECTION ( 'NONE',  ( 0.3090169943749475623, 8.338696094058001131E-17, 0.9510565162951536422 ) ) ;
#24882=EDGE_LOOP ( 'NONE', ( #14593, #23228, #14132, #12242 ) ) ;
#24885=AXIS2_PLACEMENT_3D ( 'NONE', #16771, #9432, #7019 ) ;
#24888=ORIENTED_EDGE ( 'NONE', *, *, #27246, .T. ) ;
#24889=VECTOR ( 'NONE', #11947, 1000.000000000000000 ) ;
#24891=CARTESIAN_POINT ( 'NONE',  ( 156.1922820468853388, -1.999999999999975353, -4.936203717676158398 ) ) ;
#24893=ORIENTED_EDGE ( 'NONE', *, *, #23049, .T. ) ;
#24894=CARTESIAN_POINT ( 'NONE',  ( 153.6922820468853388, -1.999999999999976241, -17.92658477444275533 ) ) ;
#24895=AXIS2_PLACEMENT_3D ( 'NONE', #18252, #15808, #1954 ) ;
#24896=FACE_OUTER_BOUND ( 'NONE', #22316, .T. ) ;
#24897=VECTOR ( 'NONE', #16218, 1000.000000000000000 ) ;
#24898=CARTESIAN_POINT ( 'NONE',  ( 136.1922820468854241, -10.00000000000000533, -10.74328820663507322 ) ) ;
#24900=CARTESIAN_POINT ( 'NONE',  ( 173.6922820468852535, -4.999999999999969802, 2.247092850131519715 ) ) ;
#24901=ORIENTED_EDGE ( 'NONE', *, *, #16238, .T. ) ;
#24902=ORIENTED_EDGE ( 'NONE', *, *, #4737, .T. ) ;
#24903=CARTESIAN_POINT ( 'NONE',  ( 162.2287565553229172, -1.999999999999972689, -12.16987298107780369 ) ) ;
#24906=ORIENTED_EDGE ( 'NONE', *, *, #13482, .F. ) ;
#24907=DIRECTION ( 'NONE',  ( -2.698458740408365879E-16, 1.000000000000000000, 0.000000000000000000 ) ) ;
#24908=EDGE_CURVE ( 'NONE', #26572, #24722, #24574, .T. ) ;
#24910=CARTESIAN_POINT ( 'NONE',  ( 163.6922820468853388, -9.999999999999998224, -15.07341522555727664 ) ) ;
#24911=DIRECTION ( 'NONE',  ( -2.698458740408365879E-16, 1.000000000000000000, 0.000000000000000000 ) ) ;
#24912=EDGE_CURVE ( 'NONE', #4960, #3275, #21662, .T. ) ;
#24913=EDGE_CURVE ( 'NONE', #22429, #722, #28736, .T. ) ;
#24914=ORIENTED_EDGE ( 'NONE', *, *, #20809, .T. ) ;
#24915=CARTESIAN_POINT ( 'NONE',  ( 134.5152310637605808, -1.999999999999980460, -28.60870317832789311 ) ) ;
#24916=ADVANCED_FACE ( 'NONE', ( #16937 ), #26417, .T. ) ;
#24917=ORIENTED_EDGE ( 'NONE', *, *, #9965, .F. ) ;
#24919=VECTOR ( 'NONE', #2393, 1000.000000000000000 ) ;
#24921=VECTOR ( 'NONE', #11894, 1000.000000000000000 ) ;
#24923=LINE ( 'NONE', #6593, #19390 ) ;
#24924=LINE ( 'NONE', #6869, #20872 ) ;
#24925=CARTESIAN_POINT ( 'NONE',  ( 144.7287565553230309, -4.999999999999978684, -33.82050807568879947 ) ) ;
#24933=FACE_OUTER_BOUND ( 'NONE', #402, .T. ) ;
#24934=VECTOR ( 'NONE', #23584, 1000.000000000000000 ) ;
#24935=ADVANCED_FACE ( 'NONE', ( #17382 ), #4114, .T. ) ;
#24936=PLANE ( 'NONE',  #27682 ) ;
#24937=CARTESIAN_POINT ( 'NONE',  ( 159.5152310637605240, -9.999999999999998224, -30.37205893520531319 ) ) ;
#24938=VECTOR ( 'NONE', #15626, 1000.000000000000000 ) ;
#24942=LINE ( 'NONE', #29419, #6340 ) ;
#24943=ORIENTED_EDGE ( 'NONE', *, *, #19776, .T. ) ;
#24944=CARTESIAN_POINT ( 'NONE',  ( 12.82896712056928124, -5.000000000000014211, 39.48350090593866923 ) ) ;
#24946=EDGE_LOOP ( 'NONE', ( #11119, #10215, #2852, #7864, #11583 ) ) ;
#24949=DIRECTION ( 'NONE',  ( -2.698458740408365879E-16, 1.000000000000000000, 0.000000000000000000 ) ) ;
#24950=CARTESIAN_POINT ( 'NONE',  ( 171.1922820468853672, -9.999999999999994671, -30.91696583120936026 ) ) ;
#24951=PLANE ( 'NONE',  #23016 ) ;
#24952=EDGE_CURVE ( 'NONE', #6495, #26976, #27501, .T. ) ;
#24954=ORIENTED_EDGE ( 'NONE', *, *, #16896, .F. ) ;
#24956=CARTESIAN_POINT ( 'NONE',  ( 176.1922820468853388, -1.999999999999969580, -28.06379628232387802 ) ) ;
#24957=EDGE_CURVE ( 'NONE', #28570, #2318, #6099, .T. ) ;
#24960=DIRECTION ( 'NONE',  ( 0.9510565162951536422, 0.000000000000000000, -0.3090169943749475623 ) ) ;
#24964=ORIENTED_EDGE ( 'NONE', *, *, #3406, .T. ) ;
#24966=ORIENTED_EDGE ( 'NONE', *, *, #15085, .T. ) ;
#24967=ORIENTED_EDGE ( 'NONE', *, *, #23419, .F. ) ;
#24971=ORIENTED_EDGE ( 'NONE', *, *, #9024, .F. ) ;
#24975=CARTESIAN_POINT ( 'NONE',  ( 168.6922820468853672, -1.999999999999970912, -26.58683881228715862 ) ) ;
#24976=CARTESIAN_POINT ( 'NONE',  ( 137.0152310637605808, -4.999999999999980460, -17.38167787843870826 ) ) ;
#24977=DIRECTION ( 'NONE',  ( -0.9510565162951536422, 0.000000000000000000, -0.3090169943749472292 ) ) ;
#24979=AXIS2_PLACEMENT_3D ( 'NONE', #11870, #14604, #5167 ) ;
#24980=FACE_OUTER_BOUND ( 'NONE', #27475, .T. ) ;
#24984=ORIENTED_EDGE ( 'NONE', *, *, #2349, .F. ) ;
#24985=DIRECTION ( 'NONE',  ( -0.5877852522924731371, -1.586114251531760235E-16, 0.8090169943749474513 ) ) ;
#24987=DIRECTION ( 'NONE',  ( -2.698458740408365879E-16, 1.000000000000000000, 0.000000000000000000 ) ) ;
#24988=CARTESIAN_POINT ( 'NONE',  ( 102.1495906963740623, -4.999999999999989342, -74.21602185925650019 ) ) ;
#24990=DIRECTION ( 'NONE',  ( -2.698458740408365879E-16, 1.000000000000000000, 0.000000000000000000 ) ) ;
#24995=DIRECTION ( 'NONE',  ( 0.9510565162951536422, 2.566386769018988816E-16, 0.3090169943749472292 ) ) ;
#24996=CARTESIAN_POINT ( 'NONE',  ( 129.5152310637605524, -1.999999999999982236, -21.71180489736090991 ) ) ;
#24997=LINE ( 'NONE', #1650, #24405 ) ;
#24998=ORIENTED_EDGE ( 'NONE', *, *, #29487, .T. ) ;
#24999=ORIENTED_EDGE ( 'NONE', *, *, #22323, .T. ) ;
#25006=CARTESIAN_POINT ( 'NONE',  ( 136.1922820468854241, -4.999999999999980460, -28.06379628232387446 ) ) ;
#25008=ORIENTED_EDGE ( 'NONE', *, *, #3278, .T. ) ;
#25010=ADVANCED_FACE ( 'NONE', ( #10965 ), #29661, .T. ) ;
#25011=FACE_OUTER_BOUND ( 'NONE', #8100, .T. ) ;
#25012=CARTESIAN_POINT ( 'NONE',  ( 156.1922820468853956, -10.00000000000000000, -19.40354224447947828 ) ) ;
#25013=CARTESIAN_POINT ( 'NONE',  ( 174.5152310637604103, -1.999999999999970024, -2.627941064794695691 ) ) ;
#25015=VERTEX_POINT ( 'NONE', #1992 ) ;
#25018=VECTOR ( 'NONE', #13827, 1000.000000000000000 ) ;
#25020=CARTESIAN_POINT ( 'NONE',  ( 143.6922820468854525, -4.999999999999978684, -23.73366926340167282 ) ) ;
#25022=CARTESIAN_POINT ( 'NONE',  ( 172.7287565553229456, -4.999999999999971578, 0.5000000000000029976 ) ) ;
#25023=VERTEX_POINT ( 'NONE', #15843 ) ;
#25024=ORIENTED_EDGE ( 'NONE', *, *, #5815, .T. ) ;
#25025=CARTESIAN_POINT ( 'NONE',  ( 159.5152310637604955, -4.999999999999974243, -1.770974823053889042E-14 ) ) ;
#25027=CARTESIAN_POINT ( 'NONE',  ( 157.0152310637604955, -4.999999999999975131, -17.38167787843871182 ) ) ;
#25028=ORIENTED_EDGE ( 'NONE', *, *, #19173, .F. ) ;
#25029=CARTESIAN_POINT ( 'NONE',  ( 167.2287565553229456, -4.999999999999972466, -12.16987298107780013 ) ) ;
#25030=ORIENTED_EDGE ( 'NONE', *, *, #23379, .F. ) ;
#25034=ORIENTED_EDGE ( 'NONE', *, *, #25610, .T. ) ;
#25038=VECTOR ( 'NONE', #20661, 1000.000000000000000 ) ;
#25039=DIRECTION ( 'NONE',  ( -0.8090169943749474513, -2.183098979609982436E-16, -0.5877852522924731371 ) ) ;
#25040=EDGE_CURVE ( 'NONE', #357, #18885, #15996, .T. ) ;
#25042=ADVANCED_FACE ( 'NONE', ( #15548 ), #10673, .T. ) ;
#25044=EDGE_CURVE ( 'NONE', #22963, #25794, #22433, .T. ) ;
#25045=ORIENTED_EDGE ( 'NONE', *, *, #20809, .F. ) ;
#25048=CARTESIAN_POINT ( 'NONE',  ( 154.5152310637604955, -1.999999999999974909, -13.05155085951651195 ) ) ;
#25049=VERTEX_POINT ( 'NONE', #1536 ) ;
#25050=DIRECTION ( 'NONE',  ( 0.5877852522924731371, 1.586114251531760728E-16, 0.8090169943749474513 ) ) ;
#25053=DIRECTION ( 'NONE',  ( 1.110223024625156540E-16, 2.995891024602366092E-32, 1.000000000000000000 ) ) ;
#25054=ORIENTED_EDGE ( 'NONE', *, *, #11481, .F. ) ;
#25055=LINE ( 'NONE', #22466, #8838 ) ;
#25058=FACE_OUTER_BOUND ( 'NONE', #23884, .T. ) ;
#25060=ORIENTED_EDGE ( 'NONE', *, *, #28880, .T. ) ;
#25065=LINE ( 'NONE', #23080, #28911 ) ;
#25070=ORIENTED_EDGE ( 'NONE', *, *, #892, .T. ) ;
#25071=LINE ( 'NONE', #6456, #16194 ) ;
#25072=EDGE_CURVE ( 'NONE', #11670, #29672, #20427, .T. ) ;
#25075=DIRECTION ( 'NONE',  ( 0.5877852522924731371, 1.586114251531760728E-16, -0.8090169943749474513 ) ) ;
#25078=VECTOR ( 'NONE', #18503, 1000.000000000000000 ) ;
#25081=VERTEX_POINT ( 'NONE', #8968 ) ;
#25082=LINE ( 'NONE', #4170, #18346 ) ;
#25083=ORIENTED_EDGE ( 'NONE', *, *, #8829, .F. ) ;
#25085=CARTESIAN_POINT ( 'NONE',  ( 142.0152310637605524, -4.999999999999979572, -1.576685793744487278E-14 ) ) ;
#25087=FACE_OUTER_BOUND ( 'NONE', #18141, .T. ) ;
#25088=CARTESIAN_POINT ( 'NONE',  ( 129.5152310637605524, -1.999999999999982236, -13.05155085951650840 ) ) ;
#25090=VERTEX_POINT ( 'NONE', #25029 ) ;
#25091=ORIENTED_EDGE ( 'NONE', *, *, #10771, .T. ) ;
#25094=EDGE_LOOP ( 'NONE', ( #16929, #23262, #25739, #13428, #13805 ) ) ;
#25096=PLANE ( 'NONE',  #3976 ) ;
#25098=AXIS2_PLACEMENT_3D ( 'NONE', #28642, #14546, #5257 ) ;
#25102=CARTESIAN_POINT ( 'NONE',  ( 166.1922820468853672, -1.999999999999970912, -28.06379628232387802 ) ) ;
#25105=EDGE_LOOP ( 'NONE', ( #3962, #13778, #28605, #15959 ) ) ;
#25107=CARTESIAN_POINT ( 'NONE',  ( 157.2287565553229456, -1.999999999999974021, -12.16987298107780369 ) ) ;
#25108=ADVANCED_FACE ( 'NONE', ( #8826 ), #18284, .T. ) ;
#25109=ADVANCED_FACE ( 'NONE', ( #12957 ), #22272, .T. ) ;
#25110=EDGE_CURVE ( 'NONE', #19118, #8559, #2587, .T. ) ;
#25111=PLANE ( 'NONE',  #29972 ) ;
#25112=EDGE_CURVE ( 'NONE', #13066, #19416, #11413, .T. ) ;
#25113=VERTEX_POINT ( 'NONE', #11862 ) ;
#25115=CARTESIAN_POINT ( 'NONE',  ( 169.7287565553229172, -1.999999999999970468, -16.50000000000000355 ) ) ;
#25117=AXIS2_PLACEMENT_3D ( 'NONE', #1560, #22606, #7951 ) ;
#25122=CARTESIAN_POINT ( 'NONE',  ( 148.6922820468854241, -1.999999999999976241, -15.07341522555727664 ) ) ;
#25124=CARTESIAN_POINT ( 'NONE',  ( 132.0152310637605808, -1.999999999999981348, -32.93883019725009120 ) ) ;
#25127=CARTESIAN_POINT ( 'NONE',  ( 147.0152310637604955, -4.999999999999977796, -1.632196944975744474E-14 ) ) ;
#25128=VERTEX_POINT ( 'NONE', #25603 ) ;
#25129=ORIENTED_EDGE ( 'NONE', *, *, #4198, .F. ) ;
#25133=CARTESIAN_POINT ( 'NONE',  ( 167.0152310637604955, -1.999999999999971356, -15.61832212156129707 ) ) ;
#25134=CARTESIAN_POINT ( 'NONE',  ( 4.794903815660978452, -5.000000000000016875, 14.75719653579859347 ) ) ;
#25135=FACE_OUTER_BOUND ( 'NONE', #30253, .T. ) ;
#25136=VERTEX_POINT ( 'NONE', #9569 ) ;
#25140=VECTOR ( 'NONE', #27068, 1000.000000000000000 ) ;
#25143=DIRECTION ( 'NONE',  ( -2.698458740408365879E-16, 1.000000000000000000, 0.000000000000000000 ) ) ;
#25145=ORIENTED_EDGE ( 'NONE', *, *, #28365, .F. ) ;
#25146=EDGE_CURVE ( 'NONE', #12292, #19109, #9113, .T. ) ;
#25147=LINE ( 'NONE', #10802, #5517 ) ;
#25149=VECTOR ( 'NONE', #18240, 1000.000000000000000 ) ;
#25152=DIRECTION ( 'NONE',  ( -2.698458740408365879E-16, 1.000000000000000000, 0.000000000000000000 ) ) ;
#25154=VECTOR ( 'NONE', #18887, 1000.000000000000000 ) ;
#25158=VECTOR ( 'NONE', #17459, 1000.000000000000000 ) ;
#25160=ORIENTED_EDGE ( 'NONE', *, *, #27732, .F. ) ;
#25162=CARTESIAN_POINT ( 'NONE',  ( 138.6922820468854525, -10.00000000000000533, -32.39392330124607611 ) ) ;
#25163=PLANE ( 'NONE',  #13333 ) ;
#25165=DIRECTION ( 'NONE',  ( 0.9510565162951536422, 0.000000000000000000, -0.3090169943749475623 ) ) ;
#25166=VERTEX_POINT ( 'NONE', #25771 ) ;
#25168=VERTEX_POINT ( 'NONE', #9266 ) ;
#25169=LINE ( 'NONE', #6702, #23183 ) ;
#25170=DIRECTION ( 'NONE',  ( -2.698458740408365879E-16, 1.000000000000000000, 0.000000000000000000 ) ) ;
#25172=ORIENTED_EDGE ( 'NONE', *, *, #14950, .F. ) ;
#25173=DIRECTION ( 'NONE',  ( 0.3090169943749472292, 8.338696094057992503E-17, -0.9510565162951536422 ) ) ;
#25176=EDGE_CURVE ( 'NONE', #22060, #20312, #28088, .T. ) ;
#25180=VECTOR ( 'NONE', #15311, 1000.000000000000000 ) ;
#25182=EDGE_LOOP ( 'NONE', ( #9567, #16187, #27331, #22579 ) ) ;
#25186=ORIENTED_EDGE ( 'NONE', *, *, #7535, .F. ) ;
#25187=PLANE ( 'NONE',  #11025 ) ;
#25188=CARTESIAN_POINT ( 'NONE',  ( 176.1922820468852819, -1.999999999999969580, -13.59645775552055902 ) ) ;
#25190=CARTESIAN_POINT ( 'NONE',  ( 126.3258676456270564, -4.999999999999984013, -91.78111523172451314 ) ) ;
#25191=CARTESIAN_POINT ( 'NONE',  ( 161.1922820468853672, -1.999999999999972689, -19.40354224447947828 ) ) ;
#25192=CARTESIAN_POINT ( 'NONE',  ( 168.6922820468853956, -1.999999999999970468, -35.24709285013155835 ) ) ;
#25193=ORIENTED_EDGE ( 'NONE', *, *, #8692, .F. ) ;
#25194=ORIENTED_EDGE ( 'NONE', *, *, #4909, .T. ) ;
#25195=CARTESIAN_POINT ( 'NONE',  ( 137.2287565553230309, -4.999999999999981348, -3.509618943233400401 ) ) ;
#25196=AXIS2_PLACEMENT_3D ( 'NONE', #7681, #21115, #221 ) ;
#25200=ORIENTED_EDGE ( 'NONE', *, *, #12072, .F. ) ;
#25201=AXIS2_PLACEMENT_3D ( 'NONE', #17532, #15241, #3368 ) ;
#25202=CARTESIAN_POINT ( 'NONE',  ( 153.6922820468853388, -10.00000000000000178, 2.247092850131519715 ) ) ;
#25203=VECTOR ( 'NONE', #279, 1000.000000000000000 ) ;
#25206=CARTESIAN_POINT ( 'NONE',  ( 159.7287565553229172, -4.999999999999975131, -7.839745962155600267 ) ) ;
#25208=LINE ( 'NONE', #18175, #19801 ) ;
#25209=VERTEX_POINT ( 'NONE', #435 ) ;
#25213=VECTOR ( 'NONE', #13167, 1000.000000000000000 ) ;
#25216=ORIENTED_EDGE ( 'NONE', *, *, #17817, .F. ) ;
#25219=DIRECTION ( 'NONE',  ( 0.9510565162951535312, 2.566386769018988816E-16, -0.3090169943749475623 ) ) ;
#25226=CARTESIAN_POINT ( 'NONE',  ( 95.42913260352182192, -4.999999999999991118, 69.33332324712154104 ) ) ;
#25227=AXIS2_PLACEMENT_3D ( 'NONE', #6935, #1918, #23109 ) ;
#25228=LINE ( 'NONE', #15453, #5711 ) ;
#25229=PLANE ( 'NONE',  #12141 ) ;
#25230=DIRECTION ( 'NONE',  ( -0.9510565162951536422, 0.000000000000000000, -0.3090169943749472292 ) ) ;
#25232=CARTESIAN_POINT ( 'NONE',  ( 133.6922820468854241, -1.999999999999981348, -0.6060766987539614181 ) ) ;
#25234=PLANE ( 'NONE',  #28142 ) ;
#25235=EDGE_LOOP ( 'NONE', ( #24577, #20464, #23762, #10288 ) ) ;
#25237=VECTOR ( 'NONE', #5952, 1000.000000000000000 ) ;
#25239=DIRECTION ( 'NONE',  ( -2.698458740408365879E-16, 1.000000000000000000, 0.000000000000000000 ) ) ;
#25242=ORIENTED_EDGE ( 'NONE', *, *, #17621, .T. ) ;
#25243=DIRECTION ( 'NONE',  ( -2.698458740408365879E-16, 1.000000000000000000, 0.000000000000000000 ) ) ;
#25245=ORIENTED_EDGE ( 'NONE', *, *, #23562, .F. ) ;
#25246=EDGE_CURVE ( 'NONE', #13920, #10352, #13711, .T. ) ;
#25249=DIRECTION ( 'NONE',  ( 0.3090169943749475623, 8.338696094058001131E-17, 0.9510565162951536422 ) ) ;
#25250=VERTEX_POINT ( 'NONE', #28400 ) ;
#25251=ADVANCED_FACE ( 'NONE', ( #14151 ), #7454, .T. ) ;
#25254=EDGE_CURVE ( 'NONE', #6140, #16946, #23173, .T. ) ;
#25257=CARTESIAN_POINT ( 'NONE',  ( 22.76426963133880221, -5.000000000000011546, -70.06121788019005692 ) ) ;
#25260=ORIENTED_EDGE ( 'NONE', *, *, #6403, .T. ) ;
#25261=ORIENTED_EDGE ( 'NONE', *, *, #19616, .T. ) ;
#25262=LINE ( 'NONE', #4347, #17540 ) ;
#25263=VECTOR ( 'NONE', #30049, 1000.000000000000000 ) ;
#25266=VECTOR ( 'NONE', #11563, 999.9999999999998863 ) ;
#25267=CARTESIAN_POINT ( 'NONE',  ( 176.1922820468852535, -9.999999999999994671, -2.083034168790677043 ) ) ;
#25269=DIRECTION ( 'NONE',  ( -1.000000000000000000, -2.698458740408365879E-16, 1.779203565104417375E-16 ) ) ;
#25276=DIRECTION ( 'NONE',  ( -0.5877852522924731371, 0.000000000000000000, 0.8090169943749474513 ) ) ;
#25278=PLANE ( 'NONE',  #10722 ) ;
#25280=DIRECTION ( 'NONE',  ( 0.5877852522924731371, 1.586114251531760728E-16, -0.8090169943749474513 ) ) ;
#25282=ORIENTED_EDGE ( 'NONE', *, *, #17246, .F. ) ;
#25284=CARTESIAN_POINT ( 'NONE',  ( 152.2287565553230024, -1.999999999999974909, -20.83012701892220520 ) ) ;
#25285=ORIENTED_EDGE ( 'NONE', *, *, #7200, .F. ) ;
#25286=ADVANCED_FACE ( 'NONE', ( #11555 ), #25926, .F. ) ;
#25287=EDGE_CURVE ( 'NONE', #16652, #29408, #20871, .T. ) ;
#25288=ADVANCED_FACE ( 'NONE', ( #4701 ), #13993, .T. ) ;
#25289=ORIENTED_EDGE ( 'NONE', *, *, #23417, .T. ) ;
#25290=EDGE_CURVE ( 'NONE', #2121, #15637, #136, .T. ) ;
#25296=AXIS2_PLACEMENT_3D ( 'NONE', #16908, #21796, #26392 ) ;
#25297=LINE ( 'NONE', #20397, #24512 ) ;
#25300=EDGE_LOOP ( 'NONE', ( #18479, #6184, #15526, #2752, #10136 ) ) ;
#25302=DIRECTION ( 'NONE',  ( 1.110223024625156540E-16, 2.995891024602366092E-32, 1.000000000000000000 ) ) ;
#25303=ORIENTED_EDGE ( 'NONE', *, *, #10601, .F. ) ;
#25305=FACE_OUTER_BOUND ( 'NONE', #6705, .T. ) ;
#25306=DIRECTION ( 'NONE',  ( -0.8090169943749474513, -2.183098979609982436E-16, 0.5877852522924731371 ) ) ;
#25309=VECTOR ( 'NONE', #7214, 1000.000000000000000 ) ;
#25311=ORIENTED_EDGE ( 'NONE', *, *, #23772, .F. ) ;
#25313=DIRECTION ( 'NONE',  ( 1.110223024625156540E-16, 2.995891024602366092E-32, 1.000000000000000000 ) ) ;
#25315=DIRECTION ( 'NONE',  ( 0.5877852522924731371, 1.586114251531760728E-16, -0.8090169943749474513 ) ) ;
#25317=DIRECTION ( 'NONE',  ( 1.110223024625156540E-16, 2.995891024602366092E-32, 1.000000000000000000 ) ) ;
#25318=EDGE_LOOP ( 'NONE', ( #20065, #327, #16527, #23393 ) ) ;
#25319=CARTESIAN_POINT ( 'NONE',  ( 157.0152310637604671, -1.999999999999974909, 1.702185954127501066 ) ) ;
#25320=EDGE_CURVE ( 'NONE', #25907, #4151, #1160, .T. ) ;
#25322=ORIENTED_EDGE ( 'NONE', *, *, #27483, .T. ) ;
#25324=EDGE_CURVE ( 'NONE', #22451, #25397, #10294, .T. ) ;
#25327=EDGE_CURVE ( 'NONE', #7152, #5129, #29586, .T. ) ;
#25334=VECTOR ( 'NONE', #30128, 1000.000000000000000 ) ;
#25336=VECTOR ( 'NONE', #19650, 1000.000000000000000 ) ;
#25337=CARTESIAN_POINT ( 'NONE',  ( 162.0152310637604103, -1.999999999999973577, -0.06116980274991495881 ) ) ;
#25338=DIRECTION ( 'NONE',  ( -0.9510565162951536422, 0.000000000000000000, -0.3090169943749472292 ) ) ;
#25339=EDGE_CURVE ( 'NONE', #6838, #7265, #17763, .T. ) ;
#25343=ORIENTED_EDGE ( 'NONE', *, *, #8456, .T. ) ;
#25344=DIRECTION ( 'NONE',  ( -0.9510565162951536422, -2.566386769018988323E-16, 0.3090169943749475623 ) ) ;
#25347=DIRECTION ( 'NONE',  ( -2.698458740408365879E-16, 1.000000000000000000, 0.000000000000000000 ) ) ;
#25348=ORIENTED_EDGE ( 'NONE', *, *, #22671, .F. ) ;
#25349=VECTOR ( 'NONE', #15658, 1000.000000000000000 ) ;
#25350=VERTEX_POINT ( 'NONE', #17315 ) ;
#25354=CARTESIAN_POINT ( 'NONE',  ( 147.0152310637605524, -1.999999999999976685, -17.38167787843871182 ) ) ;
#25355=VECTOR ( 'NONE', #11395, 1000.000000000000000 ) ;
#25356=ORIENTED_EDGE ( 'NONE', *, *, #11405, .F. ) ;
#25357=LINE ( 'NONE', #20463, #25674 ) ;
#25358=ORIENTED_EDGE ( 'NONE', *, *, #20200, .F. ) ;
#25363=CARTESIAN_POINT ( 'NONE',  ( 162.0152310637604387, -1.999999999999973133, -8.721423840594312082 ) ) ;
#25367=VECTOR ( 'NONE', #23585, 1000.000000000000000 ) ;
#25370=EDGE_LOOP ( 'NONE', ( #26577, #512, #5077, #22762 ) ) ;
#25371=DIRECTION ( 'NONE',  ( 0.5877852522924731371, 1.586114251531760728E-16, -0.8090169943749474513 ) ) ;
#25372=AXIS2_PLACEMENT_3D ( 'NONE', #27959, #21190, #9590 ) ;
#25375=CARTESIAN_POINT ( 'NONE',  ( 144.5152310637605524, -1.999999999999977573, -13.05155085951651195 ) ) ;
#25377=DIRECTION ( 'NONE',  ( -0.9510565162951536422, -2.566386769018988816E-16, -0.3090169943749472292 ) ) ;
#25381=VECTOR ( 'NONE', #8188, 1000.000000000000000 ) ;
#25383=ORIENTED_EDGE ( 'NONE', *, *, #12930, .F. ) ;
#25384=CARTESIAN_POINT ( 'NONE',  ( 159.5152310637604387, -4.999999999999974243, -4.391296821672111328 ) ) ;
#25385=ORIENTED_EDGE ( 'NONE', *, *, #7121, .F. ) ;
#25389=CARTESIAN_POINT ( 'NONE',  ( 152.2287565553229456, -10.00000000000000178, -3.509618943233403510 ) ) ;
#25390=CARTESIAN_POINT ( 'NONE',  ( 169.5152310637604387, -9.999999999999996447, -13.05155085951651195 ) ) ;
#25392=ORIENTED_EDGE ( 'NONE', *, *, #17179, .F. ) ;
#25393=ORIENTED_EDGE ( 'NONE', *, *, #23556, .T. ) ;
#25394=CARTESIAN_POINT ( 'NONE',  ( 23.71918465946406229, -5.000000000000011546, -73.00014414165241305 ) ) ;
#25396=EDGE_CURVE ( 'NONE', #22051, #20539, #1017, .T. ) ;
#25397=VERTEX_POINT ( 'NONE', #19749 ) ;
#25399=LINE ( 'NONE', #14226, #15662 ) ;
#25400=DIRECTION ( 'NONE',  ( -0.5877852522924731371, 0.000000000000000000, 0.8090169943749474513 ) ) ;
#25402=ORIENTED_EDGE ( 'NONE', *, *, #8952, .T. ) ;
#25403=PLANE ( 'NONE',  #6679 ) ;
#25406=VERTEX_POINT ( 'NONE', #24808 ) ;
#25407=AXIS2_PLACEMENT_3D ( 'NONE', #6361, #13363, #22687 ) ;
#25408=DIRECTION ( 'NONE',  ( -2.698458740408365879E-16, 1.000000000000000000, 0.000000000000000000 ) ) ;
#25409=VECTOR ( 'NONE', #21748, 1000.000000000000000 ) ;
#25411=EDGE_CURVE ( 'NONE', #22699, #966, #12167, .T. ) ;
#25412=EDGE_CURVE ( 'NONE', #3067, #2371, #29118, .T. ) ;
#25413=CARTESIAN_POINT ( 'NONE',  ( 144.5152310637605524, -4.999999999999978684, -1.604441369360116192E-14 ) ) ;
#25414=CARTESIAN_POINT ( 'NONE',  ( 167.0152310637604103, -4.999999999999972466, -0.06116980274991495881 ) ) ;
#25415=EDGE_CURVE ( 'NONE', #4159, #11708, #10894, .T. ) ;
#25417=EDGE_CURVE ( 'NONE', #19263, #14150, #6180, .T. ) ;
#25418=DIRECTION ( 'NONE',  ( -2.698458740408365879E-16, 1.000000000000000000, 0.000000000000000000 ) ) ;
#25422=LINE ( 'NONE', #16097, #8061 ) ;
#25424=PLANE ( 'NONE',  #12232 ) ;
#25425=LINE ( 'NONE', #24988, #9528 ) ;
#25426=FACE_OUTER_BOUND ( 'NONE', #1456, .T. ) ;
#25427=ORIENTED_EDGE ( 'NONE', *, *, #8065, .F. ) ;
#25428=LINE ( 'NONE', #697, #14889 ) ;
#25431=VECTOR ( 'NONE', #17304, 1000.000000000000000 ) ;
#25432=LINE ( 'NONE', #13809, #28601 ) ;
#25433=DIRECTION ( 'NONE',  ( -2.698458740408365879E-16, 1.000000000000000000, 0.000000000000000000 ) ) ;
#25442=VECTOR ( 'NONE', #14645, 1000.000000000000000 ) ;
#25443=ORIENTED_EDGE ( 'NONE', *, *, #2942, .F. ) ;
#25444=FACE_OUTER_BOUND ( 'NONE', #26004, .T. ) ;
#25445=ORIENTED_EDGE ( 'NONE', *, *, #7697, .F. ) ;
#25446=CARTESIAN_POINT ( 'NONE',  ( 142.2287565553230309, -1.999999999999978018, -20.83012701892220164 ) ) ;
#25447=ORIENTED_EDGE ( 'NONE', *, *, #3278, .F. ) ;
#25448=VERTEX_POINT ( 'NONE', #24504 ) ;
#25450=PLANE ( 'NONE',  #4121 ) ;
#25451=EDGE_CURVE ( 'NONE', #26769, #10452, #26656, .T. ) ;
#25452=ADVANCED_FACE ( 'NONE', ( #12884 ), #14450, .T. ) ;
#25453=DIRECTION ( 'NONE',  ( -2.698458740408366372E-16, 1.000000000000000000, 0.000000000000000000 ) ) ;
#25456=ORIENTED_EDGE ( 'NONE', *, *, #24246, .F. ) ;
#25457=PLANE ( 'NONE',  #28373 ) ;
#25458=CARTESIAN_POINT ( 'NONE',  ( 158.6922820468854241, -9.999999999999998224, -32.39392330124607611 ) ) ;
#25460=FACE_BOUND ( 'NONE', #26201, .T. ) ;
#25461=FACE_OUTER_BOUND ( 'NONE', #2721, .T. ) ;
#25462=EDGE_LOOP ( 'NONE', ( #1697, #10415, #12379, #17962, #17649 ) ) ;
#25463=CARTESIAN_POINT ( 'NONE',  ( 144.7287565553230309, -1.999999999999977129, -33.82050807568879947 ) ) ;
#25465=VERTEX_POINT ( 'NONE', #2883 ) ;
#25466=ORIENTED_EDGE ( 'NONE', *, *, #23846, .T. ) ;
#25468=EDGE_LOOP ( 'NONE', ( #21663, #18931, #9260, #12163 ) ) ;
#25472=ORIENTED_EDGE ( 'NONE', *, *, #6301, .T. ) ;
#25474=CARTESIAN_POINT ( 'NONE',  ( 168.6922820468853388, -1.999999999999971356, -17.92658477444275889 ) ) ;
#25476=ORIENTED_EDGE ( 'NONE', *, *, #14268, .F. ) ;
#25479=VECTOR ( 'NONE', #21188, 1000.000000000000000 ) ;
#25480=ORIENTED_EDGE ( 'NONE', *, *, #15028, .T. ) ;
#25481=LINE ( 'NONE', #7168, #21776 ) ;
#25482=DIRECTION ( 'NONE',  ( -0.5877852522924731371, 0.000000000000000000, 0.8090169943749474513 ) ) ;
#25483=DIRECTION ( 'NONE',  ( -0.5877852522924731371, -1.586114251531760235E-16, 0.8090169943749474513 ) ) ;
#25485=EDGE_CURVE ( 'NONE', #12041, #5801, #3447, .T. ) ;
#25486=DIRECTION ( 'NONE',  ( 1.110223024625156540E-16, 2.995891024602366092E-32, 1.000000000000000000 ) ) ;
#25488=VECTOR ( 'NONE', #26242, 1000.000000000000000 ) ;
#25489=EDGE_CURVE ( 'NONE', #28726, #15010, #26973, .T. ) ;
#25493=CARTESIAN_POINT ( 'NONE',  ( 159.5152310637605240, -9.999999999999998224, -19.94844914048349693 ) ) ;
#25495=VERTEX_POINT ( 'NONE', #11051 ) ;
#25496=DIRECTION ( 'NONE',  ( -0.5877852522924731371, -1.586114251531760235E-16, 0.8090169943749474513 ) ) ;
#25504=CARTESIAN_POINT ( 'NONE',  ( 133.6922820468854241, -10.00000000000000711, -15.07341522555727309 ) ) ;
#25505=LINE ( 'NONE', #5347, #8166 ) ;
#25506=ORIENTED_EDGE ( 'NONE', *, *, #18942, .F. ) ;
#25508=ORIENTED_EDGE ( 'NONE', *, *, #21137, .T. ) ;
#25512=EDGE_LOOP ( 'NONE', ( #18248, #20165, #4222, #10438, #25466 ) ) ;
#25514=CARTESIAN_POINT ( 'NONE',  ( 139.5152310637605808, -4.999999999999980460, -13.05155085951651195 ) ) ;
#25520=DIRECTION ( 'NONE',  ( 0.9510565162951536422, 2.566386769018988816E-16, 0.3090169943749472292 ) ) ;
#25521=EDGE_CURVE ( 'NONE', #6680, #12148, #2215, .T. ) ;
#25522=CARTESIAN_POINT ( 'NONE',  ( 139.5152310637605808, -10.00000000000000533, -13.05155085951651195 ) ) ;
#25523=LINE ( 'NONE', #18343, #24328 ) ;
#25525=AXIS2_PLACEMENT_3D ( 'NONE', #11103, #6391, #27025 ) ;
#25527=DIRECTION ( 'NONE',  ( -0.9510565162951536422, 0.000000000000000000, -0.3090169943749472292 ) ) ;
#25528=DIRECTION ( 'NONE',  ( -2.698458740408365879E-16, 1.000000000000000000, 0.000000000000000000 ) ) ;
#25529=ORIENTED_EDGE ( 'NONE', *, *, #7725, .F. ) ;
#25533=LINE ( 'NONE', #13772, #24346 ) ;
#25535=ORIENTED_EDGE ( 'NONE', *, *, #24702, .T. ) ;
#25536=ORIENTED_EDGE ( 'NONE', *, *, #25875, .F. ) ;
#25537=CARTESIAN_POINT ( 'NONE',  ( 138.6922820468854525, -10.00000000000000533, -9.266330736598359152 ) ) ;
#25539=EDGE_LOOP ( 'NONE', ( #17206, #5006, #28780, #17403, #18772, #21577, #1341, #10089 ) ) ;
#25542=DIRECTION ( 'NONE',  ( 0.5877852522924731371, 0.000000000000000000, 0.8090169943749474513 ) ) ;
#25544=EDGE_LOOP ( 'NONE', ( #20498, #18465, #29682, #27715 ) ) ;
#25545=LINE ( 'NONE', #25102, #10569 ) ;
#25549=AXIS2_PLACEMENT_3D ( 'NONE', #22831, #4648, #4955 ) ;
#25550=ORIENTED_EDGE ( 'NONE', *, *, #3640, .F. ) ;
#25551=DIRECTION ( 'NONE',  ( 0.9510565162951536422, 0.000000000000000000, -0.3090169943749475623 ) ) ;
#25552=FACE_OUTER_BOUND ( 'NONE', #3166, .T. ) ;
#25553=DIRECTION ( 'NONE',  ( -2.698458740408365879E-16, 1.000000000000000000, -0.000000000000000000 ) ) ;
#25554=CARTESIAN_POINT ( 'NONE',  ( 175.7287565553229456, -4.999999999999969802, -28.21440484423852979 ) ) ;
#25559=ORIENTED_EDGE ( 'NONE', *, *, #13930, .T. ) ;
#25561=AXIS2_PLACEMENT_3D ( 'NONE', #19138, #7844, #26329 ) ;
#25562=DIRECTION ( 'NONE',  ( 0.9510565162951535312, 2.566386769018988816E-16, -0.3090169943749475623 ) ) ;
#25563=FACE_OUTER_BOUND ( 'NONE', #17383, .T. ) ;
#25565=VERTEX_POINT ( 'NONE', #2066 ) ;
#25566=DIRECTION ( 'NONE',  ( -0.5877852522924731371, -1.586114251531760728E-16, -0.8090169943749474513 ) ) ;
#25568=ORIENTED_EDGE ( 'NONE', *, *, #5718, .T. ) ;
#25570=CARTESIAN_POINT ( 'NONE',  ( 157.0152310637605240, -1.999999999999974021, -15.61832212156129707 ) ) ;
#25572=ORIENTED_EDGE ( 'NONE', *, *, #18884, .F. ) ;
#25574=ORIENTED_EDGE ( 'NONE', *, *, #27935, .T. ) ;
#25578=ADVANCED_FACE ( 'NONE', ( #11196 ), #27879, .T. ) ;
#25580=EDGE_CURVE ( 'NONE', #15051, #9036, #20353, .T. ) ;
#25582=VECTOR ( 'NONE', #12560, 999.9999999999998863 ) ;
#25583=VERTEX_POINT ( 'NONE', #20649 ) ;
#25585=CARTESIAN_POINT ( 'NONE',  ( 156.1922820468853956, -10.00000000000000000, -22.25671179336496053 ) ) ;
#25586=ORIENTED_EDGE ( 'NONE', *, *, #20743, .T. ) ;
#25588=PLANE ( 'NONE',  #28531 ) ;
#25589=CARTESIAN_POINT ( 'NONE',  ( 134.5152310637605524, -10.00000000000000533, -21.71180489736090991 ) ) ;
#25592=ORIENTED_EDGE ( 'NONE', *, *, #18559, .F. ) ;
#25593=DIRECTION ( 'NONE',  ( -0.8090169943749474513, -2.183098979609982436E-16, -0.5877852522924731371 ) ) ;
#25594=CARTESIAN_POINT ( 'NONE',  ( 142.0152310637605808, -4.999999999999979572, -1.576685793744487594E-14 ) ) ;
#25597=CARTESIAN_POINT ( 'NONE',  ( 132.0152310637605524, -4.999999999999982236, -1.465663491281971624E-14 ) ) ;
#25598=EDGE_LOOP ( 'NONE', ( #16360, #17368, #8902, #27974 ) ) ;
#25599=LINE ( 'NONE', #25767, #297 ) ;
#25601=FACE_OUTER_BOUND ( 'NONE', #14380, .T. ) ;
#25603=CARTESIAN_POINT ( 'NONE',  ( 144.5152310637605240, -1.999999999999978018, -4.391296821672111328 ) ) ;
#25604=ORIENTED_EDGE ( 'NONE', *, *, #26602, .F. ) ;
#25607=ADVANCED_FACE ( 'NONE', ( #4338 ), #30036, .T. ) ;
#25610=EDGE_CURVE ( 'NONE', #18285, #6891, #18217, .T. ) ;
#25612=ADVANCED_FACE ( 'NONE', ( #22814 ), #16229, .T. ) ;
#25614=CARTESIAN_POINT ( 'NONE',  ( 162.2287565553229740, -1.999999999999971800, -29.49038105676660493 ) ) ;
#25616=EDGE_CURVE ( 'NONE', #6165, #25166, #8749, .T. ) ;
#25618=DIRECTION ( 'NONE',  ( -2.698458740408365879E-16, 1.000000000000000000, 0.000000000000000000 ) ) ;
#25621=AXIS2_PLACEMENT_3D ( 'NONE', #2725, #28856, #25923 ) ;
#25622=ORIENTED_EDGE ( 'NONE', *, *, #11914, .T. ) ;
#25623=PLANE ( 'NONE',  #10544 ) ;
#25624=LINE ( 'NONE', #11875, #13275 ) ;
#25625=CARTESIAN_POINT ( 'NONE',  ( 167.0152310637604671, -4.999999999999971578, -6.958068083716895558 ) ) ;
#25631=DIRECTION ( 'NONE',  ( -0.8090169943749474513, -2.183098979609982436E-16, 0.5877852522924731371 ) ) ;
#25633=VECTOR ( 'NONE', #6949, 1000.000000000000000 ) ;
#25634=EDGE_LOOP ( 'NONE', ( #24610, #11305, #29338, #24603 ) ) ;
#25637=DIRECTION ( 'NONE',  ( 6.938893903907227392E-16, -0.000000000000000000, 1.000000000000000000 ) ) ;
#25640=LINE ( 'NONE', #26106, #9705 ) ;
#25641=ORIENTED_EDGE ( 'NONE', *, *, #22874, .T. ) ;
#25642=ORIENTED_EDGE ( 'NONE', *, *, #10268, .F. ) ;
#25644=DIRECTION ( 'NONE',  ( -2.698458740408365879E-16, 1.000000000000000000, 0.000000000000000000 ) ) ;
#25645=VECTOR ( 'NONE', #24534, 1000.000000000000000 ) ;
#25647=DIRECTION ( 'NONE',  ( -0.5877852522924731371, 0.000000000000000000, 0.8090169943749474513 ) ) ;
#25648=CARTESIAN_POINT ( 'NONE',  ( 149.7287565553229740, -1.999999999999976241, -7.839745962155603820 ) ) ;
#25651=ORIENTED_EDGE ( 'NONE', *, *, #2557, .T. ) ;
#25653=ORIENTED_EDGE ( 'NONE', *, *, #20077, .F. ) ;
#25654=VECTOR ( 'NONE', #17418, 1000.000000000000000 ) ;
#25657=ORIENTED_EDGE ( 'NONE', *, *, #16829, .F. ) ;
#25659=VECTOR ( 'NONE', #1446, 1000.000000000000000 ) ;
#25661=ADVANCED_FACE ( 'NONE', ( #16072 ), #22661, .T. ) ;
#25662=EDGE_CURVE ( 'NONE', #18003, #23706, #18068, .T. ) ;
#25663=ADVANCED_FACE ( 'NONE', ( #30186 ), #9196, .T. ) ;
#25664=CARTESIAN_POINT ( 'NONE',  ( 167.0152310637605524, -9.999999999999996447, -32.93883019725009120 ) ) ;
#25668=ORIENTED_EDGE ( 'NONE', *, *, #29210, .T. ) ;
#25669=CARTESIAN_POINT ( 'NONE',  ( 148.6922820468853956, -1.999999999999976685, -6.413161187712876909 ) ) ;
#25671=EDGE_LOOP ( 'NONE', ( #22595, #14924, #25245, #4944, #27923, #10322 ) ) ;
#25672=DIRECTION ( 'NONE',  ( -1.110223024625156540E-16, 0.000000000000000000, -1.000000000000000000 ) ) ;
#25673=CARTESIAN_POINT ( 'NONE',  ( 151.1922820468853672, -10.00000000000000178, -2.083034168790677043 ) ) ;
#25674=VECTOR ( 'NONE', #4450, 1000.000000000000000 ) ;
#25675=LINE ( 'NONE', #23090, #1221 ) ;
#25679=CARTESIAN_POINT ( 'NONE',  ( 152.0152310637604955, -4.999999999999976907, -15.61832212156129351 ) ) ;
#25680=ORIENTED_EDGE ( 'NONE', *, *, #4274, .T. ) ;
#25682=LINE ( 'NONE', #2800, #6188 ) ;
#25683=ORIENTED_EDGE ( 'NONE', *, *, #9126, .F. ) ;
#25688=DIRECTION ( 'NONE',  ( -2.698458740408365879E-16, 1.000000000000000000, 0.000000000000000000 ) ) ;
#25694=CARTESIAN_POINT ( 'NONE',  ( 162.0152310637604387, -1.999999999999973577, 1.702185954127501066 ) ) ;
#25695=ORIENTED_EDGE ( 'NONE', *, *, #9505, .T. ) ;
#25696=ORIENTED_EDGE ( 'NONE', *, *, #17850, .F. ) ;
#25697=EDGE_CURVE ( 'NONE', #7245, #17600, #23561, .T. ) ;
#25698=DIRECTION ( 'NONE',  ( 0.5877852522924731371, 0.000000000000000000, 0.8090169943749474513 ) ) ;
#25700=ADVANCED_FACE ( 'NONE', ( #7389 ), #14681, .T. ) ;
#25701=ORIENTED_EDGE ( 'NONE', *, *, #14473, .T. ) ;
#25702=EDGE_CURVE ( 'NONE', #10712, #18131, #376, .T. ) ;
#25703=DIRECTION ( 'NONE',  ( 0.9510565162951536422, 2.566386769018988816E-16, 0.3090169943749472292 ) ) ;
#25707=VECTOR ( 'NONE', #15316, 1000.000000000000000 ) ;
#25710=EDGE_LOOP ( 'NONE', ( #20448, #18765, #13730, #17376 ) ) ;
#25712=CARTESIAN_POINT ( 'NONE',  ( 133.6922820468854241, -1.999999999999980904, -32.39392330124607611 ) ) ;
#25713=ORIENTED_EDGE ( 'NONE', *, *, #16918, .T. ) ;
#25714=CARTESIAN_POINT ( 'NONE',  ( 144.7287565553230024, -10.00000000000000355, -7.839745962155603820 ) ) ;
#25715=LINE ( 'NONE', #23425, #12703 ) ;
#25716=ORIENTED_EDGE ( 'NONE', *, *, #28491, .F. ) ;
#25717=LINE ( 'NONE', #4800, #26063 ) ;
#25722=ADVANCED_FACE ( 'NONE', ( #26161 ), #2972, .T. ) ;
#25724=ORIENTED_EDGE ( 'NONE', *, *, #7439, .F. ) ;
#25727=CARTESIAN_POINT ( 'NONE',  ( 174.7287565553229456, -9.999999999999994671, -33.82050807568879947 ) ) ;
#25730=VERTEX_POINT ( 'NONE', #2815 ) ;
#25731=CARTESIAN_POINT ( 'NONE',  ( 133.7287565553229456, -9.999999999999982236, 3.500000000000003109 ) ) ;
#25733=ORIENTED_EDGE ( 'NONE', *, *, #16900, .F. ) ;
#25734=CARTESIAN_POINT ( 'NONE',  ( 167.0152310637604387, -1.999999999999972244, 1.702185954127501066 ) ) ;
#25735=PLANE ( 'NONE',  #7868 ) ;
#25738=ADVANCED_FACE ( 'NONE', ( #12395 ), #23872, .T. ) ;
#25739=ORIENTED_EDGE ( 'NONE', *, *, #16517, .T. ) ;
#25747=ORIENTED_EDGE ( 'NONE', *, *, #8829, .T. ) ;
#25750=DIRECTION ( 'NONE',  ( 1.000000000000000000, 2.698458740408365879E-16, -1.110223024625156540E-16 ) ) ;
#25751=VERTEX_POINT ( 'NONE', #16376 ) ;
#25752=CARTESIAN_POINT ( 'NONE',  ( 158.6922820468853672, -10.00000000000000000, -15.07341522555727664 ) ) ;
#25754=EDGE_CURVE ( 'NONE', #3594, #18808, #2660, .T. ) ;
#25757=EDGE_CURVE ( 'NONE', #10926, #26594, #21112, .T. ) ;
#25758=ORIENTED_EDGE ( 'NONE', *, *, #16701, .T. ) ;
#25760=DIRECTION ( 'NONE',  ( -0.9510565162951536422, 0.000000000000000000, -0.3090169943749472292 ) ) ;
#25761=FACE_OUTER_BOUND ( 'NONE', #799, .T. ) ;
#25763=CARTESIAN_POINT ( 'NONE',  ( 133.6922820468854241, -4.999999999999981348, 2.247092850131519715 ) ) ;
#25764=CARTESIAN_POINT ( 'NONE',  ( 143.6922820468854525, -4.999999999999978684, -26.58683881228715506 ) ) ;
#25765=ORIENTED_EDGE ( 'NONE', *, *, #14205, .T. ) ;
#25767=CARTESIAN_POINT ( 'NONE',  ( 123.4761516755868627, -4.999999999999984901, -89.71067538675424657 ) ) ;
#25771=CARTESIAN_POINT ( 'NONE',  ( 176.1922820468852535, -1.999999999999969358, -2.083034168790677931 ) ) ;
#25772=EDGE_LOOP ( 'NONE', ( #25356, #12947, #15906, #15224 ) ) ;
#25774=VERTEX_POINT ( 'NONE', #5087 ) ;
#25775=AXIS2_PLACEMENT_3D ( 'NONE', #11578, #25631, #4721 ) ;
#25778=CARTESIAN_POINT ( 'NONE',  ( 174.5152310637604103, -1.999999999999969580, -13.05155085951651195 ) ) ;
#25779=CARTESIAN_POINT ( 'NONE',  ( 4.396394917579590889, -5.000000000000016875, 13.53071226075565470 ) ) ;
#25780=DIRECTION ( 'NONE',  ( -1.110223024625156540E-16, 0.000000000000000000, -1.000000000000000000 ) ) ;
#25782=ORIENTED_EDGE ( 'NONE', *, *, #18382, .T. ) ;
#25783=CARTESIAN_POINT ( 'NONE',  ( 147.0152310637604955, -10.00000000000000355, -0.06116980274991495881 ) ) ;
#25784=DIRECTION ( 'NONE',  ( -2.698458740408365879E-16, 1.000000000000000000, 0.000000000000000000 ) ) ;
#25785=VECTOR ( 'NONE', #10427, 1000.000000000000000 ) ;
#25787=DIRECTION ( 'NONE',  ( 1.110223024625156540E-16, 2.995891024602366092E-32, 1.000000000000000000 ) ) ;
#25788=DIRECTION ( 'NONE',  ( -2.698458740408365879E-16, 1.000000000000000000, 0.000000000000000000 ) ) ;
#25791=ADVANCED_FACE ( 'NONE', ( #9497 ), #4936, .T. ) ;
#25792=DIRECTION ( 'NONE',  ( -0.5877852522924731371, -1.586114251531760235E-16, 0.8090169943749474513 ) ) ;
#25794=VERTEX_POINT ( 'NONE', #14529 ) ;
#25796=ADVANCED_FACE ( 'NONE', ( #28023 ), #9656, .T. ) ;
#25797=FACE_OUTER_BOUND ( 'NONE', #14576, .T. ) ;
#25798=ADVANCED_FACE ( 'NONE', ( #19265 ), #9349, .T. ) ;
#25801=FACE_OUTER_BOUND ( 'NONE', #29429, .T. ) ;
#25803=ORIENTED_EDGE ( 'NONE', *, *, #25489, .F. ) ;
#25805=CARTESIAN_POINT ( 'NONE',  ( 153.6922820468853388, -10.00000000000000178, 2.247092850131519715 ) ) ;
#25807=DIRECTION ( 'NONE',  ( -1.110223024625156540E-16, 0.000000000000000000, -1.000000000000000000 ) ) ;
#25810=DIRECTION ( 'NONE',  ( -2.698458740408365879E-16, 1.000000000000000000, 0.000000000000000000 ) ) ;
#25811=VERTEX_POINT ( 'NONE', #14227 ) ;
#25813=EDGE_LOOP ( 'NONE', ( #7630, #1256, #7814, #22149 ) ) ;
#25814=VECTOR ( 'NONE', #23385, 1000.000000000000000 ) ;
#25819=EDGE_LOOP ( 'NONE', ( #16986, #29676, #27157, #3728 ) ) ;
#25821=DIRECTION ( 'NONE',  ( 0.5877852522924731371, 0.000000000000000000, 0.8090169943749474513 ) ) ;
#25826=DIRECTION ( 'NONE',  ( -0.8090169943749474513, -2.183098979609982436E-16, 0.5877852522924731371 ) ) ;
#25827=DIRECTION ( 'NONE',  ( -2.698458740408365879E-16, 1.000000000000000000, 0.000000000000000000 ) ) ;
#25829=CARTESIAN_POINT ( 'NONE',  ( 131.1922820468854241, -10.00000000000000888, -22.25671179336495697 ) ) ;
#25830=VECTOR ( 'NONE', #19073, 999.9999999999998863 ) ;
#25831=DIRECTION ( 'NONE',  ( -2.698458740408365879E-16, 1.000000000000000000, 0.000000000000000000 ) ) ;
#25832=EDGE_CURVE ( 'NONE', #30106, #5942, #25858, .T. ) ;
#25833=DIRECTION ( 'NONE',  ( -2.698458740408365879E-16, 1.000000000000000000, 0.000000000000000000 ) ) ;
#25834=EDGE_CURVE ( 'NONE', #3555, #14905, #18977, .T. ) ;
#25835=EDGE_CURVE ( 'NONE', #6518, #24599, #14375, .T. ) ;
#25836=VECTOR ( 'NONE', #20258, 1000.000000000000000 ) ;
#25838=VECTOR ( 'NONE', #23929, 1000.000000000000000 ) ;
#25839=EDGE_CURVE ( 'NONE', #9877, #7345, #9809, .T. ) ;
#25840=LINE ( 'NONE', #26141, #29019 ) ;
#25841=EDGE_LOOP ( 'NONE', ( #4677, #15994, #22574, #4200 ) ) ;
#25843=ORIENTED_EDGE ( 'NONE', *, *, #25834, .T. ) ;
#25848=DIRECTION ( 'NONE',  ( -0.5877852522924731371, -1.586114251531760235E-16, 0.8090169943749474513 ) ) ;
#25849=DIRECTION ( 'NONE',  ( -2.698458740408365879E-16, 1.000000000000000000, 0.000000000000000000 ) ) ;
#25851=EDGE_LOOP ( 'NONE', ( #24506, #9418, #2958, #7747 ) ) ;
#25852=DIRECTION ( 'NONE',  ( -0.5877852522924731371, 0.000000000000000000, 0.8090169943749474513 ) ) ;
#25856=VECTOR ( 'NONE', #13181, 1000.000000000000000 ) ;
#25857=FACE_OUTER_BOUND ( 'NONE', #20610, .T. ) ;
#25858=LINE ( 'NONE', #7081, #5243 ) ;
#25860=VERTEX_POINT ( 'NONE', #5991 ) ;
#25865=ORIENTED_EDGE ( 'NONE', *, *, #13208, .T. ) ;
#25866=VERTEX_POINT ( 'NONE', #24461 ) ;
#25867=LINE ( 'NONE', #7838, #17152 ) ;
#25868=DIRECTION ( 'NONE',  ( -2.698458740408365879E-16, 1.000000000000000000, 0.000000000000000000 ) ) ;
#25869=VECTOR ( 'NONE', #5309, 1000.000000000000000 ) ;
#25871=DIRECTION ( 'NONE',  ( -2.698458740408365879E-16, 1.000000000000000000, -0.000000000000000000 ) ) ;
#25872=VECTOR ( 'NONE', #14031, 1000.000000000000000 ) ;
#25873=ADVANCED_FACE ( 'NONE', ( #28785 ), #10713, .T. ) ;
#25875=EDGE_CURVE ( 'NONE', #888, #10558, #29081, .T. ) ;
#25877=EDGE_CURVE ( 'NONE', #29393, #24131, #5547, .T. ) ;
#25881=EDGE_LOOP ( 'NONE', ( #8372, #12956, #1543, #161 ) ) ;
#25883=CARTESIAN_POINT ( 'NONE',  ( 144.5152310637605808, -4.999999999999978684, -30.37205893520530964 ) ) ;
#25885=CARTESIAN_POINT ( 'NONE',  ( 156.1922820468853388, -10.00000000000000178, -2.083034168790677043 ) ) ;
#25886=LINE ( 'NONE', #14254, #25367 ) ;
#25888=LINE ( 'NONE', #18705, #21727 ) ;
#25892=DIRECTION ( 'NONE',  ( -2.698458740408366372E-16, 1.000000000000000000, 0.000000000000000000 ) ) ;
#25893=DIRECTION ( 'NONE',  ( -2.698458740408365879E-16, 1.000000000000000000, 0.000000000000000000 ) ) ;
#25901=AXIS2_PLACEMENT_3D ( 'NONE', #4489, #26006, #7078 ) ;
#25905=ORIENTED_EDGE ( 'NONE', *, *, #27551, .F. ) ;
#25906=LINE ( 'NONE', #14276, #9893 ) ;
#25907=VERTEX_POINT ( 'NONE', #6143 ) ;
#25908=FACE_OUTER_BOUND ( 'NONE', #1193, .T. ) ;
#25909=ORIENTED_EDGE ( 'NONE', *, *, #20077, .T. ) ;
#25910=DIRECTION ( 'NONE',  ( 0.9510565162951536422, 2.566386769018988816E-16, 0.3090169943749472292 ) ) ;
#25911=ADVANCED_FACE ( 'NONE', ( #14828 ), #26464, .T. ) ;
#25914=VECTOR ( 'NONE', #13844, 1000.000000000000000 ) ;
#25916=EDGE_LOOP ( 'NONE', ( #3809, #14037, #9302, #12585 ) ) ;
#25918=LINE ( 'NONE', #7735, #24624 ) ;
#25923=DIRECTION ( 'NONE',  ( 0.5877852522924731371, 0.000000000000000000, 0.8090169943749474513 ) ) ;
#25924=LINE ( 'NONE', #9416, #26872 ) ;
#25925=ORIENTED_EDGE ( 'NONE', *, *, #16100, .F. ) ;
#25926=PLANE ( 'NONE',  #20323 ) ;
#25927=ORIENTED_EDGE ( 'NONE', *, *, #25112, .F. ) ;
#25931=DIRECTION ( 'NONE',  ( -2.698458740408365879E-16, 1.000000000000000000, 0.000000000000000000 ) ) ;
#25933=PLANE ( 'NONE',  #24979 ) ;
#25937=LINE ( 'NONE', #21497, #7911 ) ;
#25938=FACE_OUTER_BOUND ( 'NONE', #2545, .T. ) ;
#25939=CARTESIAN_POINT ( 'NONE',  ( 176.1922820468852819, -9.999999999999994671, -10.74328820663507678 ) ) ;
#25942=CARTESIAN_POINT ( 'NONE',  ( 163.6922820468853104, -9.999999999999998224, -9.266330736598359152 ) ) ;
#25944=VERTEX_POINT ( 'NONE', #24312 ) ;
#25946=ORIENTED_EDGE ( 'NONE', *, *, #14740, .T. ) ;
#25948=VECTOR ( 'NONE', #490, 1000.000000000000000 ) ;
#25952=ORIENTED_EDGE ( 'NONE', *, *, #131, .T. ) ;
#25953=EDGE_LOOP ( 'NONE', ( #29515, #754, #30174, #1380 ) ) ;
#25954=ORIENTED_EDGE ( 'NONE', *, *, #23626, .F. ) ;
#25956=DIRECTION ( 'NONE',  ( -8.163404592832029035E-16, -2.202861047501738386E-31, -1.000000000000000000 ) ) ;
#25958=CARTESIAN_POINT ( 'NONE',  ( 144.5152310637605524, -10.00000000000000355, -13.05155085951651195 ) ) ;
#25960=CARTESIAN_POINT ( 'NONE',  ( 172.0152310637603819, -9.999999999999996447, -0.06116980274991495881 ) ) ;
#25967=VECTOR ( 'NONE', #17255, 1000.000000000000000 ) ;
#25968=ORIENTED_EDGE ( 'NONE', *, *, #16137, .T. ) ;
#25973=EDGE_CURVE ( 'NONE', #486, #25166, #3556, .T. ) ;
#25974=EDGE_CURVE ( 'NONE', #1366, #29409, #12544, .T. ) ;
#25976=EDGE_CURVE ( 'NONE', #17665, #28008, #972, .T. ) ;
#25979=EDGE_CURVE ( 'NONE', #10099, #15678, #15439, .T. ) ;
#25980=ORIENTED_EDGE ( 'NONE', *, *, #7157, .T. ) ;
#25981=CARTESIAN_POINT ( 'NONE',  ( 133.7287565553229456, -84.33034373659253902, -41.50000000000000000 ) ) ;
#25984=PLANE ( 'NONE',  #26216 ) ;
#25989=FACE_OUTER_BOUND ( 'NONE', #882, .T. ) ;
#25990=EDGE_LOOP ( 'NONE', ( #18253, #20389, #727, #8561, #12619 ) ) ;
#25991=LINE ( 'NONE', #16968, #7591 ) ;
#25992=EDGE_LOOP ( 'NONE', ( #7455, #14861, #19838, #13108 ) ) ;
#25994=ORIENTED_EDGE ( 'NONE', *, *, #19781, .F. ) ;
#25996=VECTOR ( 'NONE', #28984, 1000.000000000000000 ) ;
#26001=VERTEX_POINT ( 'NONE', #24769 ) ;
#26004=EDGE_LOOP ( 'NONE', ( #1051, #20334, #15977, #29216 ) ) ;
#26006=DIRECTION ( 'NONE',  ( 0.3090169943749475623, 8.338696094058001131E-17, 0.9510565162951536422 ) ) ;
#26007=ORIENTED_EDGE ( 'NONE', *, *, #21722, .F. ) ;
#26008=DIRECTION ( 'NONE',  ( 2.908569913943825061E-16, -1.000000000000000000, -6.826925868028081731E-18 ) ) ;
#26011=VERTEX_POINT ( 'NONE', #1126 ) ;
#26013=ORIENTED_EDGE ( 'NONE', *, *, #27323, .T. ) ;
#26015=EDGE_CURVE ( 'NONE', #8715, #16514, #19568, .T. ) ;
#26018=EDGE_CURVE ( 'NONE', #25015, #28921, #26616, .T. ) ;
#26019=DIRECTION ( 'NONE',  ( -2.698458740408365879E-16, 1.000000000000000000, 0.000000000000000000 ) ) ;
#26020=EDGE_CURVE ( 'NONE', #2818, #25866, #10106, .T. ) ;
#26022=ORIENTED_EDGE ( 'NONE', *, *, #3982, .T. ) ;
#26024=AXIS2_PLACEMENT_3D ( 'NONE', #21122, #20811, #16240 ) ;
#26025=LINE ( 'NONE', #9668, #9919 ) ;
#26027=LINE ( 'NONE', #9510, #10656 ) ;
#26028=VERTEX_POINT ( 'NONE', #17426 ) ;
#26029=DIRECTION ( 'NONE',  ( -2.698458740408365879E-16, 1.000000000000000000, 0.000000000000000000 ) ) ;
#26034=ORIENTED_EDGE ( 'NONE', *, *, #23556, .F. ) ;
#26035=LINE ( 'NONE', #12567, #15384 ) ;
#26037=DIRECTION ( 'NONE',  ( -2.698458740408365879E-16, 1.000000000000000000, 0.000000000000000000 ) ) ;
#26038=CARTESIAN_POINT ( 'NONE',  ( 157.0152310637604955, -1.999999999999974465, -6.958068083716895558 ) ) ;
#26039=LINE ( 'NONE', #28050, #1487 ) ;
#26040=DIRECTION ( 'NONE',  ( 0.3090169943749475623, 8.338696094058001131E-17, 0.9510565162951536422 ) ) ;
#26042=DIRECTION ( 'NONE',  ( 0.9510565162951535312, 2.566386769018988816E-16, -0.3090169943749475623 ) ) ;
#26043=LINE ( 'NONE', #18710, #11758 ) ;
#26047=ORIENTED_EDGE ( 'NONE', *, *, #27967, .T. ) ;
#26052=EDGE_CURVE ( 'NONE', #29696, #7452, #17280, .T. ) ;
#26053=EDGE_CURVE ( 'NONE', #8387, #14514, #1271, .T. ) ;
#26057=ORIENTED_EDGE ( 'NONE', *, *, #30122, .F. ) ;
#26058=ORIENTED_EDGE ( 'NONE', *, *, #29044, .F. ) ;
#26060=CARTESIAN_POINT ( 'NONE',  ( 100.8811111486825780, -4.999999999999990230, -73.29441752195363335 ) ) ;
#26061=ORIENTED_EDGE ( 'NONE', *, *, #22669, .F. ) ;
#26062=CARTESIAN_POINT ( 'NONE',  ( 169.5152310637604387, -4.999999999999971578, -13.05155085951651195 ) ) ;
#26063=VECTOR ( 'NONE', #27586, 1000.000000000000000 ) ;
#26064=ORIENTED_EDGE ( 'NONE', *, *, #5812, .T. ) ;
#26065=CARTESIAN_POINT ( 'NONE',  ( 168.6922820468853672, -9.999999999999996447, -23.73366926340167637 ) ) ;
#26070=FACE_OUTER_BOUND ( 'NONE', #3802, .T. ) ;
#26071=DIRECTION ( 'NONE',  ( 0.9510565162951535312, 2.566386769018988816E-16, -0.3090169943749475623 ) ) ;
#26077=LINE ( 'NONE', #21483, #5869 ) ;
#26078=EDGE_LOOP ( 'NONE', ( #17568, #27190, #7048, #8511 ) ) ;
#26079=CARTESIAN_POINT ( 'NONE',  ( 97.12043866711040607, -4.999999999999991118, 70.56212903019198279 ) ) ;
#26080=EDGE_LOOP ( 'NONE', ( #4695, #23573, #28632, #21096, #1465 ) ) ;
#26083=EDGE_CURVE ( 'NONE', #220, #6891, #22478, .T. ) ;
#26086=CARTESIAN_POINT ( 'NONE',  ( 168.6922820468853672, -4.999999999999971578, -23.73366926340167637 ) ) ;
#26087=VECTOR ( 'NONE', #18994, 1000.000000000000000 ) ;
#26088=LINE ( 'NONE', #9424, #18135 ) ;
#26090=EDGE_LOOP ( 'NONE', ( #2437, #6434, #13593, #25045 ) ) ;
#26092=VECTOR ( 'NONE', #28849, 1000.000000000000000 ) ;
#26093=CARTESIAN_POINT ( 'NONE',  ( 153.6922820468853388, -1.999999999999975797, -15.07341522555727309 ) ) ;
#26094=CARTESIAN_POINT ( 'NONE',  ( 152.0152310637604955, -10.00000000000000178, 1.702185954127501066 ) ) ;
#26095=LINE ( 'NONE', #16462, #18064 ) ;
#26098=CARTESIAN_POINT ( 'NONE',  ( 115.2397606401234924, -4.999999999999985789, -83.72658702220800819 ) ) ;
#26100=EDGE_LOOP ( 'NONE', ( #24717, #5646, #4392, #23829, #18215 ) ) ;
#26102=CARTESIAN_POINT ( 'NONE',  ( 137.0152310637606092, -4.999999999999980460, -32.93883019725009120 ) ) ;
#26106=CARTESIAN_POINT ( 'NONE',  ( 137.0152310637605808, -1.999999999999979572, -26.04193191628310800 ) ) ;
#26107=EDGE_LOOP ( 'NONE', ( #10688, #6812, #15409, #28839, #27217 ) ) ;
#26109=ORIENTED_EDGE ( 'NONE', *, *, #16897, .F. ) ;
#26110=ORIENTED_EDGE ( 'NONE', *, *, #24389, .F. ) ;
#26112=DIRECTION ( 'NONE',  ( 0.9510565162951535312, 2.566386769018988816E-16, -0.3090169943749475623 ) ) ;
#26114=CARTESIAN_POINT ( 'NONE',  ( 142.0152310637605808, -1.999999999999978018, -17.38167787843871182 ) ) ;
#26115=VERTEX_POINT ( 'NONE', #1725 ) ;
#26116=LINE ( 'NONE', #23826, #20300 ) ;
#26119=AXIS2_PLACEMENT_3D ( 'NONE', #21924, #8028, #22386 ) ;
#26120=ORIENTED_EDGE ( 'NONE', *, *, #20481, .F. ) ;
#26124=ORIENTED_EDGE ( 'NONE', *, *, #12896, .T. ) ;
#26126=LINE ( 'NONE', #16947, #17899 ) ;
#26127=ADVANCED_FACE ( 'NONE', ( #23078 ), #11452, .T. ) ;
#26134=FACE_BOUND ( 'NONE', #2824, .T. ) ;
#26135=CARTESIAN_POINT ( 'NONE',  ( 174.7287565553229456, -1.999999999999968470, -33.82050807568879947 ) ) ;
#26136=CARTESIAN_POINT ( 'NONE',  ( 176.1922820468853388, -9.999999999999994671, -30.91696583120936026 ) ) ;
#26137=PLANE ( 'NONE',  #8726 ) ;
#26141=CARTESIAN_POINT ( 'NONE',  ( 146.1922820468854241, -10.00000000000000355, -10.74328820663507678 ) ) ;
#26142=EDGE_CURVE ( 'NONE', #25250, #4687, #11311, .T. ) ;
#26143=DIRECTION ( 'NONE',  ( 1.000000000000000000, 2.891205793294675861E-16, 0.000000000000000000 ) ) ;
#26147=EDGE_CURVE ( 'NONE', #18723, #10809, #1884, .T. ) ;
#26148=VERTEX_POINT ( 'NONE', #9157 ) ;
#26151=CARTESIAN_POINT ( 'NONE',  ( 129.5152310637605524, -10.00000000000000888, -30.37205893520530964 ) ) ;
#26152=DIRECTION ( 'NONE',  ( -2.698458740408365879E-16, 1.000000000000000000, 0.000000000000000000 ) ) ;
#26153=CARTESIAN_POINT ( 'NONE',  ( 139.5152310637605524, -4.999999999999980460, -4.391296821672111328 ) ) ;
#26154=EDGE_LOOP ( 'NONE', ( #5990, #11873, #10708, #13847, #8995 ) ) ;
#26155=ORIENTED_EDGE ( 'NONE', *, *, #3478, .T. ) ;
#26158=ORIENTED_EDGE ( 'NONE', *, *, #5049, .F. ) ;
#26161=FACE_OUTER_BOUND ( 'NONE', #8219, .T. ) ;
#26164=ORIENTED_EDGE ( 'NONE', *, *, #230, .T. ) ;
#26165=CARTESIAN_POINT ( 'NONE',  ( 148.6922820468853672, -4.999999999999976907, 2.247092850131519715 ) ) ;
#26169=VECTOR ( 'NONE', #3863, 1000.000000000000000 ) ;
#26171=VERTEX_POINT ( 'NONE', #27243 ) ;
#26172=LINE ( 'NONE', #5405, #22441 ) ;
#26173=AXIS2_PLACEMENT_3D ( 'NONE', #8744, #30181, #13776 ) ;
#26174=( GEOMETRIC_REPRESENTATION_CONTEXT ( 3 ) GLOBAL_UNCERTAINTY_ASSIGNED_CONTEXT ( ( #1897 ) ) GLOBAL_UNIT_ASSIGNED_CONTEXT ( ( #9281, #9585, #30119 ) ) REPRESENTATION_CONTEXT ( 'NONE', 'WORKASPACE' ) );
#26176=DIRECTION ( 'NONE',  ( -0.5877852522924731371, -1.586114251531760235E-16, 0.8090169943749474513 ) ) ;
#26177=DIRECTION ( 'NONE',  ( -0.9510565162951536422, -2.566386769018988816E-16, -0.3090169943749472292 ) ) ;
#26178=CARTESIAN_POINT ( 'NONE',  ( 134.7287565553230024, -4.999999999999981348, -16.50000000000000000 ) ) ;
#26184=ORIENTED_EDGE ( 'NONE', *, *, #29061, .T. ) ;
#26185=CARTESIAN_POINT ( 'NONE',  ( 131.1922820468854241, -10.00000000000000888, -22.25671179336495697 ) ) ;
#26189=DIRECTION ( 'NONE',  ( -2.698458740408365879E-16, 1.000000000000000000, 0.000000000000000000 ) ) ;
#26191=EDGE_CURVE ( 'NONE', #16627, #20965, #24923, .T. ) ;
#26193=ORIENTED_EDGE ( 'NONE', *, *, #29204, .T. ) ;
#26194=LINE ( 'NONE', #14711, #23696 ) ;
#26197=CARTESIAN_POINT ( 'NONE',  ( 141.1922820468854241, -10.00000000000000533, -2.083034168790677043 ) ) ;
#26198=FACE_OUTER_BOUND ( 'NONE', #19734, .T. ) ;
#26201=EDGE_LOOP ( 'NONE', ( #24495, #9652, #12237, #18664, #5462 ) ) ;
#26207=EDGE_LOOP ( 'NONE', ( #4982, #919, #15308, #10684 ) ) ;
#26210=ORIENTED_EDGE ( 'NONE', *, *, #21958, .F. ) ;
#26211=AXIS2_PLACEMENT_3D ( 'NONE', #29743, #11642, #15921 ) ;
#26212=DIRECTION ( 'NONE',  ( -2.698458740408365879E-16, 1.000000000000000000, 0.000000000000000000 ) ) ;
#26214=ADVANCED_FACE ( 'NONE', ( #29858 ), #29702, .T. ) ;
#26216=AXIS2_PLACEMENT_3D ( 'NONE', #5521, #7948, #24140 ) ;
#26218=EDGE_CURVE ( 'NONE', #2461, #19125, #8716, .T. ) ;
#26220=LINE ( 'NONE', #11852, #12915 ) ;
#26224=FACE_OUTER_BOUND ( 'NONE', #26536, .T. ) ;
#26225=EDGE_CURVE ( 'NONE', #22156, #22605, #18329, .T. ) ;
#26226=DIRECTION ( 'NONE',  ( -2.698458740408365879E-16, 1.000000000000000000, 0.000000000000000000 ) ) ;
#26227=VERTEX_POINT ( 'NONE', #25363 ) ;
#26229=VECTOR ( 'NONE', #18476, 1000.000000000000000 ) ;
#26231=EDGE_LOOP ( 'NONE', ( #24469, #5313, #20187, #24758 ) ) ;
#26238=LINE ( 'NONE', #17355, #15997 ) ;
#26240=VECTOR ( 'NONE', #7805, 1000.000000000000000 ) ;
#26241=VERTEX_POINT ( 'NONE', #22932 ) ;
#26242=DIRECTION ( 'NONE',  ( -2.698458740408365879E-16, 1.000000000000000000, 0.000000000000000000 ) ) ;
#26243=ADVANCED_FACE ( 'NONE', ( #2034 ), #27687, .T. ) ;
#26244=PLANE ( 'NONE',  #19132 ) ;
#26245=FACE_OUTER_BOUND ( 'NONE', #4632, .T. ) ;
#26251=VERTEX_POINT ( 'NONE', #8566 ) ;
#26253=EDGE_CURVE ( 'NONE', #9664, #25774, #4458, .T. ) ;
#26254=CARTESIAN_POINT ( 'NONE',  ( 157.0152310637605240, -1.999999999999974021, -15.61832212156129707 ) ) ;
#26256=EDGE_CURVE ( 'NONE', #24657, #25565, #26126, .T. ) ;
#26258=LINE ( 'NONE', #21360, #17513 ) ;
#26260=ADVANCED_FACE ( 'NONE', ( #4604 ), #14041, .T. ) ;
#26261=ORIENTED_EDGE ( 'NONE', *, *, #8492, .F. ) ;
#26264=EDGE_LOOP ( 'NONE', ( #9622, #5039, #18687, #16761, #17644 ) ) ;
#26266=DIRECTION ( 'NONE',  ( -2.698458740408365879E-16, 1.000000000000000000, 0.000000000000000000 ) ) ;
#26267=ORIENTED_EDGE ( 'NONE', *, *, #20242, .T. ) ;
#26268=LINE ( 'NONE', #21820, #29137 ) ;
#26269=ORIENTED_EDGE ( 'NONE', *, *, #8452, .T. ) ;
#26271=VERTEX_POINT ( 'NONE', #23834 ) ;
#26275=LINE ( 'NONE', #772, #11120 ) ;
#26276=DIRECTION ( 'NONE',  ( -0.5877852522924731371, -1.586114251531760728E-16, -0.8090169943749474513 ) ) ;
#26278=ORIENTED_EDGE ( 'NONE', *, *, #24952, .F. ) ;
#26280=AXIS2_PLACEMENT_3D ( 'NONE', #16706, #23893, #5561 ) ;
#26282=VECTOR ( 'NONE', #14554, 1000.000000000000000 ) ;
#26285=FACE_BOUND ( 'NONE', #3319, .T. ) ;
#26286=LINE ( 'NONE', #787, #10633 ) ;
#26291=CARTESIAN_POINT ( 'NONE',  ( 142.2287565553230309, -1.999999999999978018, -12.16987298107780369 ) ) ;
#26292=ORIENTED_EDGE ( 'NONE', *, *, #25040, .T. ) ;
#26295=ORIENTED_EDGE ( 'NONE', *, *, #19479, .F. ) ;
#26297=ORIENTED_EDGE ( 'NONE', *, *, #10143, .T. ) ;
#26299=DIRECTION ( 'NONE',  ( 0.3090169943749475623, 8.338696094058001131E-17, 0.9510565162951536422 ) ) ;
#26300=FACE_OUTER_BOUND ( 'NONE', #9911, .T. ) ;
#26301=LINE ( 'NONE', #26604, #1012 ) ;
#26303=VERTEX_POINT ( 'NONE', #19089 ) ;
#26304=FACE_OUTER_BOUND ( 'NONE', #2696, .T. ) ;
#26310=CARTESIAN_POINT ( 'NONE',  ( 154.7287565553229456, -10.00000000000000178, -7.839745962155603820 ) ) ;
#26312=ORIENTED_EDGE ( 'NONE', *, *, #19479, .T. ) ;
#26317=EDGE_LOOP ( 'NONE', ( #8613, #29348, #3599, #21026 ) ) ;
#26318=CARTESIAN_POINT ( 'NONE',  ( 151.1922820468853672, -10.00000000000000178, -4.936203717676158398 ) ) ;
#26319=ORIENTED_EDGE ( 'NONE', *, *, #29711, .F. ) ;
#26320=EDGE_CURVE ( 'NONE', #11833, #14224, #7492, .T. ) ;
#26321=CARTESIAN_POINT ( 'NONE',  ( 173.6922820468852819, -1.999999999999970468, -9.266330736598359152 ) ) ;
#26322=AXIS2_PLACEMENT_3D ( 'NONE', #4282, #13585, #20145 ) ;
#26324=VECTOR ( 'NONE', #20410, 1000.000000000000000 ) ;
#26326=VECTOR ( 'NONE', #24668, 999.9999999999998863 ) ;
#26328=CARTESIAN_POINT ( 'NONE',  ( 171.1922820468853388, -9.999999999999996447, -22.25671179336496053 ) ) ;
#26329=DIRECTION ( 'NONE',  ( 0.5877852522924731371, 0.000000000000000000, 0.8090169943749474513 ) ) ;
#26336=CARTESIAN_POINT ( 'NONE',  ( 152.0152310637604671, -1.999999999999976241, -0.06116980274991495881 ) ) ;
#26337=CARTESIAN_POINT ( 'NONE',  ( 161.1922820468853956, -1.999999999999973577, -28.06379628232387446 ) ) ;
#26339=CARTESIAN_POINT ( 'NONE',  ( 146.1922820468853956, -10.00000000000000355, -2.083034168790677043 ) ) ;
#26344=CARTESIAN_POINT ( 'NONE',  ( 167.0152310637605524, -4.999999999999971578, -32.93883019725009120 ) ) ;
#26346=AXIS2_PLACEMENT_3D ( 'NONE', #804, #659, #7518 ) ;
#26348=CARTESIAN_POINT ( 'NONE',  ( 166.1922820468853672, -1.999999999999971800, -22.25671179336496053 ) ) ;
#26352=ORIENTED_EDGE ( 'NONE', *, *, #24389, .T. ) ;
#26357=EDGE_LOOP ( 'NONE', ( #21356, #14027, #4516, #3850, #1019 ) ) ;
#26358=ORIENTED_EDGE ( 'NONE', *, *, #27487, .T. ) ;
#26359=VECTOR ( 'NONE', #13983, 1000.000000000000000 ) ;
#26360=ADVANCED_FACE ( 'NONE', ( #32 ), #16798, .T. ) ;
#26361=EDGE_CURVE ( 'NONE', #14364, #19566, #14497, .T. ) ;
#26362=VECTOR ( 'NONE', #26189, 1000.000000000000000 ) ;
#26365=CARTESIAN_POINT ( 'NONE',  ( 174.7287565553228887, -4.999999999999970690, -16.50000000000000000 ) ) ;
#26366=FACE_OUTER_BOUND ( 'NONE', #1358, .T. ) ;
#26368=DIRECTION ( 'NONE',  ( -0.9510565162951536422, -2.566386769018988323E-16, 0.3090169943749475623 ) ) ;
#26369=CARTESIAN_POINT ( 'NONE',  ( 173.6922820468853104, -9.999999999999994671, -15.07341522555727664 ) ) ;
#26370=DIRECTION ( 'NONE',  ( -0.8090169943749474513, -2.183098979609982436E-16, 0.5877852522924731371 ) ) ;
#26373=CARTESIAN_POINT ( 'NONE',  ( 174.7287565553229456, -9.999999999999994671, -33.82050807568879947 ) ) ;
#26374=LINE ( 'NONE', #426, #3671 ) ;
#26378=FACE_OUTER_BOUND ( 'NONE', #18359, .T. ) ;
#26379=VECTOR ( 'NONE', #19489, 999.9999999999998863 ) ;
#26380=ORIENTED_EDGE ( 'NONE', *, *, #5670, .F. ) ;
#26381=AXIS2_PLACEMENT_3D ( 'NONE', #12839, #22151, #3995 ) ;
#26382=FACE_OUTER_BOUND ( 'NONE', #15737, .T. ) ;
#26385=ORIENTED_EDGE ( 'NONE', *, *, #7945, .F. ) ;
#26391=DIRECTION ( 'NONE',  ( 0.5877852522924731371, 0.000000000000000000, 0.8090169943749474513 ) ) ;
#26392=DIRECTION ( 'NONE',  ( -0.9510565162951536422, 0.000000000000000000, -0.3090169943749472292 ) ) ;
#26393=CARTESIAN_POINT ( 'NONE',  ( 164.5152310637604671, -1.999999999999972244, -11.28819510263909542 ) ) ;
#26394=ADVANCED_FACE ( 'NONE', ( #7049 ), #18940, .T. ) ;
#26395=ADVANCED_FACE ( 'NONE', ( #9621 ), #16339, .T. ) ;
#26396=CARTESIAN_POINT ( 'NONE',  ( 139.7287565553230309, -10.00000000000000533, -7.839745962155603820 ) ) ;
#26397=LINE ( 'NONE', #7758, #6002 ) ;
#26398=DIRECTION ( 'NONE',  ( 0.3090169943749472292, 8.338696094057992503E-17, -0.9510565162951536422 ) ) ;
#26400=CARTESIAN_POINT ( 'NONE',  ( 158.6922820468853388, -4.999999999999975131, -6.413161187712876909 ) ) ;
#26401=LINE ( 'NONE', #17223, #23595 ) ;
#26404=ORIENTED_EDGE ( 'NONE', *, *, #19402, .F. ) ;
#26408=FACE_BOUND ( 'NONE', #3867, .T. ) ;
#26410=ORIENTED_EDGE ( 'NONE', *, *, #13817, .T. ) ;
#26411=ORIENTED_EDGE ( 'NONE', *, *, #24318, .F. ) ;
#26413=CARTESIAN_POINT ( 'NONE',  ( 136.1922820468854241, -1.999999999999980016, -19.40354224447947473 ) ) ;
#26417=PLANE ( 'NONE',  #17855 ) ;
#26420=VERTEX_POINT ( 'NONE', #9318 ) ;
#26425=ORIENTED_EDGE ( 'NONE', *, *, #21482, .T. ) ;
#26426=VERTEX_POINT ( 'NONE', #21078 ) ;
#26427=CARTESIAN_POINT ( 'NONE',  ( 137.0152310637606092, -10.00000000000000533, -32.93883019725009120 ) ) ;
#26429=EDGE_LOOP ( 'NONE', ( #19785, #27377, #23482, #24646 ) ) ;
#26433=EDGE_CURVE ( 'NONE', #21693, #7797, #185, .T. ) ;
#26434=ADVANCED_FACE ( 'NONE', ( #9772 ), #18788, .T. ) ;
#26435=LINE ( 'NONE', #19388, #16391 ) ;
#26438=VECTOR ( 'NONE', #13896, 1000.000000000000000 ) ;
#26441=FACE_OUTER_BOUND ( 'NONE', #9463, .T. ) ;
#26444=DIRECTION ( 'NONE',  ( 0.3090169943749472292, 8.338696094057992503E-17, -0.9510565162951536422 ) ) ;
#26445=PLANE ( 'NONE',  #22703 ) ;
#26448=VERTEX_POINT ( 'NONE', #26576 ) ;
#26449=VECTOR ( 'NONE', #6568, 1000.000000000000000 ) ;
#26451=DIRECTION ( 'NONE',  ( -0.8090169943749474513, -2.183098979609982436E-16, 0.5877852522924731371 ) ) ;
#26452=CARTESIAN_POINT ( 'NONE',  ( 136.1922820468854241, -4.999999999999980460, -13.59645775552055547 ) ) ;
#26455=EDGE_LOOP ( 'NONE', ( #28105, #16369, #5222, #8507, #2435 ) ) ;
#26456=FACE_OUTER_BOUND ( 'NONE', #25318, .T. ) ;
#26457=VERTEX_POINT ( 'NONE', #10069 ) ;
#26459=ORIENTED_EDGE ( 'NONE', *, *, #26147, .F. ) ;
#26462=ORIENTED_EDGE ( 'NONE', *, *, #14909, .F. ) ;
#26463=ORIENTED_EDGE ( 'NONE', *, *, #19476, .T. ) ;
#26464=PLANE ( 'NONE',  #7701 ) ;
#26465=VECTOR ( 'NONE', #5624, 1000.000000000000000 ) ;
#26467=EDGE_LOOP ( 'NONE', ( #27881, #13144, #3188, #20197 ) ) ;
#26468=CARTESIAN_POINT ( 'NONE',  ( 136.1922820468854241, -10.00000000000000533, -2.083034168790677043 ) ) ;
#26472=ORIENTED_EDGE ( 'NONE', *, *, #14439, .T. ) ;
#26473=DIRECTION ( 'NONE',  ( -2.698458740408365879E-16, 1.000000000000000000, 0.000000000000000000 ) ) ;
#26474=EDGE_CURVE ( 'NONE', #12566, #25860, #29193, .T. ) ;
#26475=VERTEX_POINT ( 'NONE', #10679 ) ;
#26476=CARTESIAN_POINT ( 'NONE',  ( 143.6922820468854241, -10.00000000000000355, -6.413161187712876909 ) ) ;
#26478=LINE ( 'NONE', #19428, #18685 ) ;
#26480=DIRECTION ( 'NONE',  ( -0.5877852522924731371, -1.586114251531760235E-16, 0.8090169943749474513 ) ) ;
#26487=VERTEX_POINT ( 'NONE', #3088 ) ;
#26488=CARTESIAN_POINT ( 'NONE',  ( 169.5152310637604671, -9.999999999999996447, -11.28819510263909542 ) ) ;
#26489=CARTESIAN_POINT ( 'NONE',  ( 161.1922820468853388, -1.999999999999973133, -10.74328820663507678 ) ) ;
#26490=DIRECTION ( 'NONE',  ( 1.000000000000000000, 2.698458740408365879E-16, -1.110223024625156540E-16 ) ) ;
#26491=CARTESIAN_POINT ( 'NONE',  ( 167.0152310637605240, -1.999999999999970468, -34.70218595412750773 ) ) ;
#26493=DIRECTION ( 'NONE',  ( -0.5877852522924731371, -1.586114251531760235E-16, 0.8090169943749474513 ) ) ;
#26495=ORIENTED_EDGE ( 'NONE', *, *, #2108, .T. ) ;
#26498=EDGE_CURVE ( 'NONE', #16948, #17144, #3375, .T. ) ;
#26500=DIRECTION ( 'NONE',  ( -1.110223024625156540E-16, 0.000000000000000000, -1.000000000000000000 ) ) ;
#26503=ORIENTED_EDGE ( 'NONE', *, *, #1931, .T. ) ;
#26508=VECTOR ( 'NONE', #10611, 1000.000000000000000 ) ;
#26511=ORIENTED_EDGE ( 'NONE', *, *, #295, .T. ) ;
#26512=FACE_OUTER_BOUND ( 'NONE', #4219, .T. ) ;
#26513=VERTEX_POINT ( 'NONE', #17541 ) ;
#26514=ORIENTED_EDGE ( 'NONE', *, *, #1379, .F. ) ;
#26517=DIRECTION ( 'NONE',  ( 0.5877852522924731371, 0.000000000000000000, 0.8090169943749474513 ) ) ;
#26522=CARTESIAN_POINT ( 'NONE',  ( 173.6922820468853388, -4.999999999999970690, -26.58683881228715862 ) ) ;
#26523=CARTESIAN_POINT ( 'NONE',  ( 96.69761215121324938, -4.999999999999991118, 70.25492758442437946 ) ) ;
#26525=CARTESIAN_POINT ( 'NONE',  ( 104.5111766707794203, -4.999999999999988454, 75.93181450320298609 ) ) ;
#26526=DIRECTION ( 'NONE',  ( -0.5877852522924731371, -1.586114251531760235E-16, 0.8090169943749474513 ) ) ;
#26527=EDGE_CURVE ( 'NONE', #2080, #23514, #14941, .T. ) ;
#26528=EDGE_CURVE ( 'NONE', #26028, #29734, #26899, .T. ) ;
#26529=ORIENTED_EDGE ( 'NONE', *, *, #29988, .F. ) ;
#26532=EDGE_CURVE ( 'NONE', #21981, #5728, #5359, .T. ) ;
#26533=DIRECTION ( 'NONE',  ( -2.698458740408365879E-16, 1.000000000000000000, 0.000000000000000000 ) ) ;
#26534=ORIENTED_EDGE ( 'NONE', *, *, #7572, .F. ) ;
#26536=EDGE_LOOP ( 'NONE', ( #16640, #24114, #18574, #19380 ) ) ;
#26538=ORIENTED_EDGE ( 'NONE', *, *, #12270, .F. ) ;
#26541=CARTESIAN_POINT ( 'NONE',  ( 103.4180702440655324, -4.999999999999989342, -75.13762619655935282 ) ) ;
#26544=VECTOR ( 'NONE', #22216, 999.9999999999998863 ) ;
#26546=CARTESIAN_POINT ( 'NONE',  ( 144.5152310637606092, -1.999999999999977129, -28.60870317832789311 ) ) ;
#26547=LINE ( 'NONE', #21951, #8907 ) ;
#26549=PLANE ( 'NONE',  #10260 ) ;
#26550=LINE ( 'NONE', #17072, #22129 ) ;
#26551=VECTOR ( 'NONE', #17973, 1000.000000000000000 ) ;
#26554=VERTEX_POINT ( 'NONE', #12662 ) ;
#26558=FACE_BOUND ( 'NONE', #29275, .T. ) ;
#26562=LINE ( 'NONE', #17377, #29718 ) ;
#26566=LINE ( 'NONE', #21971, #3787 ) ;
#26567=EDGE_CURVE ( 'NONE', #22102, #2770, #12965, .T. ) ;
#26569=DIRECTION ( 'NONE',  ( -0.8090169943749474513, -2.183098979609982436E-16, -0.5877852522924731371 ) ) ;
#26570=VERTEX_POINT ( 'NONE', #12506 ) ;
#26572=VERTEX_POINT ( 'NONE', #28902 ) ;
#26575=ORIENTED_EDGE ( 'NONE', *, *, #16024, .F. ) ;
#26576=CARTESIAN_POINT ( 'NONE',  ( 152.0152310637605524, -4.999999999999976907, -26.04193191628311155 ) ) ;
#26577=ORIENTED_EDGE ( 'NONE', *, *, #8617, .T. ) ;
#26580=ORIENTED_EDGE ( 'NONE', *, *, #17873, .F. ) ;
#26584=LINE ( 'NONE', #28909, #25967 ) ;
#26585=VECTOR ( 'NONE', #19245, 1000.000000000000000 ) ;
#26589=CARTESIAN_POINT ( 'NONE',  ( 93.84789618117305565, -4.999999999999992006, 68.18448773945412711 ) ) ;
#26591=FACE_OUTER_BOUND ( 'NONE', #14152, .T. ) ;
#26592=VERTEX_POINT ( 'NONE', #22280 ) ;
#26594=VERTEX_POINT ( 'NONE', #15092 ) ;
#26599=LINE ( 'NONE', #26151, #16580 ) ;
#26601=EDGE_CURVE ( 'NONE', #16501, #21693, #10371, .T. ) ;
#26602=EDGE_CURVE ( 'NONE', #20364, #12263, #19989, .T. ) ;
#26604=CARTESIAN_POINT ( 'NONE',  ( 141.1922820468854525, -10.00000000000000533, -22.25671179336495697 ) ) ;
#26605=ORIENTED_EDGE ( 'NONE', *, *, #487, .T. ) ;
#26606=CARTESIAN_POINT ( 'NONE',  ( 139.5152310637606092, -1.999999999999978684, -19.94844914048349338 ) ) ;
#26607=EDGE_CURVE ( 'NONE', #25583, #27966, #7934, .T. ) ;
#26608=ORIENTED_EDGE ( 'NONE', *, *, #6856, .T. ) ;
#26610=ORIENTED_EDGE ( 'NONE', *, *, #10863, .T. ) ;
#26611=AXIS2_PLACEMENT_3D ( 'NONE', #4846, #3183, #7741 ) ;
#26614=ORIENTED_EDGE ( 'NONE', *, *, #12374, .F. ) ;
#26616=LINE ( 'NONE', #811, #20847 ) ;
#26618=DIRECTION ( 'NONE',  ( 0.5877852522924731371, 0.000000000000000000, 0.8090169943749474513 ) ) ;
#26620=ORIENTED_EDGE ( 'NONE', *, *, #14950, .T. ) ;
#26624=VERTEX_POINT ( 'NONE', #3522 ) ;
#26625=ORIENTED_EDGE ( 'NONE', *, *, #5290, .T. ) ;
#26628=DIRECTION ( 'NONE',  ( 0.5877852522924731371, 1.586114251531760728E-16, -0.8090169943749474513 ) ) ;
#26629=VECTOR ( 'NONE', #29183, 1000.000000000000000 ) ;
#26630=DIRECTION ( 'NONE',  ( 1.000000000000000000, 2.698458740408365879E-16, -1.110223024625156540E-16 ) ) ;
#26631=DIRECTION ( 'NONE',  ( 0.5877852522924731371, 1.586114251531760728E-16, -0.8090169943749474513 ) ) ;
#26633=VECTOR ( 'NONE', #25566, 1000.000000000000000 ) ;
#26634=LINE ( 'NONE', #16850, #30035 ) ;
#26644=EDGE_CURVE ( 'NONE', #8141, #22102, #17390, .T. ) ;
#26645=CARTESIAN_POINT ( 'NONE',  ( 141.1922820468854525, -4.999999999999978684, -28.06379628232387446 ) ) ;
#26650=EDGE_CURVE ( 'NONE', #9309, #17686, #26275, .T. ) ;
#26656=LINE ( 'NONE', #10598, #24749 ) ;
#26658=ORIENTED_EDGE ( 'NONE', *, *, #21002, .T. ) ;
#26662=AXIS2_PLACEMENT_3D ( 'NONE', #21853, #3549, #12841 ) ;
#26665=ORIENTED_EDGE ( 'NONE', *, *, #2351, .T. ) ;
#26667=PRODUCT_DEFINITION_SHAPE ( 'NONE', 'NONE',  #735 ) ;
#26668=ORIENTED_EDGE ( 'NONE', *, *, #22109, .T. ) ;
#26669=DIRECTION ( 'NONE',  ( -2.698458740408365879E-16, 1.000000000000000000, 0.000000000000000000 ) ) ;
#26670=EDGE_LOOP ( 'NONE', ( #22200, #8292, #3669, #19610 ) ) ;
#26672=ORIENTED_EDGE ( 'NONE', *, *, #29517, .F. ) ;
#26673=CARTESIAN_POINT ( 'NONE',  ( 152.0152310637604955, -1.999999999999975797, -8.721423840594312082 ) ) ;
#26674=CARTESIAN_POINT ( 'NONE',  ( 172.0152310637604103, -9.999999999999996447, -8.721423840594312082 ) ) ;
#26675=DIRECTION ( 'NONE',  ( -2.698458740408365879E-16, 1.000000000000000000, 0.000000000000000000 ) ) ;
#26676=AXIS2_PLACEMENT_3D ( 'NONE', #18071, #16379, #22968 ) ;
#26682=DIRECTION ( 'NONE',  ( -2.698458740408365879E-16, 1.000000000000000000, 0.000000000000000000 ) ) ;
#26683=LINE ( 'NONE', #26523, #14879 ) ;
#26685=PLANE ( 'NONE',  #13 ) ;
#26686=LINE ( 'NONE', #28995, #23752 ) ;
#26687=ORIENTED_EDGE ( 'NONE', *, *, #15969, .T. ) ;
#26688=DIRECTION ( 'NONE',  ( 1.110223024625156540E-16, 2.995891024602366092E-32, 1.000000000000000000 ) ) ;
#26689=LINE ( 'NONE', #15047, #14165 ) ;
#26690=ORIENTED_EDGE ( 'NONE', *, *, #3171, .T. ) ;
#26693=ORIENTED_EDGE ( 'NONE', *, *, #5155, .T. ) ;
#26694=ORIENTED_EDGE ( 'NONE', *, *, #9375, .F. ) ;
#26700=LINE ( 'NONE', #1200, #17947 ) ;
#26701=LINE ( 'NONE', #28707, #12102 ) ;
#26702=CARTESIAN_POINT ( 'NONE',  ( 173.6922820468853104, -1.999999999999970024, -17.92658477444275889 ) ) ;
#26703=AXIS2_PLACEMENT_3D ( 'NONE', #23258, #8604, #27429 ) ;
#26704=ORIENTED_EDGE ( 'NONE', *, *, #18656, .F. ) ;
#26705=DIRECTION ( 'NONE',  ( -2.698458740408365879E-16, 1.000000000000000000, 0.000000000000000000 ) ) ;
#26706=EDGE_CURVE ( 'NONE', #888, #16025, #11278, .T. ) ;
#26709=EDGE_CURVE ( 'NONE', #8269, #29449, #20433, .T. ) ;
#26710=CARTESIAN_POINT ( 'NONE',  ( 162.0152310637605240, -1.999999999999971800, -34.70218595412750773 ) ) ;
#26711=DIRECTION ( 'NONE',  ( -2.698458740408365879E-16, 1.000000000000000000, 0.000000000000000000 ) ) ;
#26717=AXIS2_PLACEMENT_3D ( 'NONE', #1840, #15839, #8527 ) ;
#26720=FACE_BOUND ( 'NONE', #11431, .T. ) ;
#26721=ORIENTED_EDGE ( 'NONE', *, *, #30020, .T. ) ;
#26723=FACE_OUTER_BOUND ( 'NONE', #2366, .T. ) ;
#26725=DIRECTION ( 'NONE',  ( -0.9510565162951536422, 0.000000000000000000, -0.3090169943749472292 ) ) ;
#26727=DIRECTION ( 'NONE',  ( -0.5877852522924731371, 0.000000000000000000, 0.8090169943749474513 ) ) ;
#26728=EDGE_LOOP ( 'NONE', ( #6260, #29188, #8056, #9819 ) ) ;
#26740=VECTOR ( 'NONE', #27444, 1000.000000000000000 ) ;
#26741=ORIENTED_EDGE ( 'NONE', *, *, #20160, .T. ) ;
#26742=DIRECTION ( 'NONE',  ( -1.110223024625156540E-16, 0.000000000000000000, -1.000000000000000000 ) ) ;
#26743=EDGE_CURVE ( 'NONE', #2635, #13495, #22897, .T. ) ;
#26744=FACE_BOUND ( 'NONE', #8231, .T. ) ;
#26746=VECTOR ( 'NONE', #292, 1000.000000000000000 ) ;
#26747=EDGE_CURVE ( 'NONE', #13010, #16269, #16003, .T. ) ;
#26749=FACE_OUTER_BOUND ( 'NONE', #25953, .T. ) ;
#26751=CARTESIAN_POINT ( 'NONE',  ( 134.5152310637605524, -10.00000000000000533, -21.71180489736090991 ) ) ;
#26753=DIRECTION ( 'NONE',  ( 0.9510565162951536422, 2.566386769018988816E-16, 0.3090169943749472292 ) ) ;
#26757=DIRECTION ( 'NONE',  ( -0.9510565162951536422, -2.566386769018988323E-16, 0.3090169943749475623 ) ) ;
#26758=ORIENTED_EDGE ( 'NONE', *, *, #10987, .F. ) ;
#26760=ORIENTED_EDGE ( 'NONE', *, *, #18897, .F. ) ;
#26762=DIRECTION ( 'NONE',  ( -0.9510565162951536422, -2.566386769018988816E-16, -0.3090169943749472292 ) ) ;
#26764=ORIENTED_EDGE ( 'NONE', *, *, #19480, .T. ) ;
#26765=EDGE_LOOP ( 'NONE', ( #16574, #5091, #13676, #11548, #15983 ) ) ;
#26766=CARTESIAN_POINT ( 'NONE',  ( 151.1922820468854241, -10.00000000000000178, -22.25671179336496053 ) ) ;
#26767=ORIENTED_EDGE ( 'NONE', *, *, #861, .F. ) ;
#26769=VERTEX_POINT ( 'NONE', #6560 ) ;
#26770=VECTOR ( 'NONE', #9671, 1000.000000000000000 ) ;
#26776=DIRECTION ( 'NONE',  ( -0.5877852522924731371, -1.586114251531760235E-16, 0.8090169943749474513 ) ) ;
#26777=FACE_OUTER_BOUND ( 'NONE', #11778, .T. ) ;
#26778=ADVANCED_FACE ( 'NONE', ( #11132 ), #13717, .T. ) ;
#26779=VECTOR ( 'NONE', #22378, 1000.000000000000000 ) ;
#26783=PLANE ( 'NONE',  #6923 ) ;
#26785=CARTESIAN_POINT ( 'NONE',  ( 136.1922820468854241, -1.999999999999980016, -28.06379628232387446 ) ) ;
#26788=CARTESIAN_POINT ( 'NONE',  ( 174.5152310637604387, -9.999999999999994671, -11.28819510263909542 ) ) ;
#26790=LINE ( 'NONE', #829, #1826 ) ;
#26792=DIRECTION ( 'NONE',  ( 0.3090169943749472292, 8.338696094057992503E-17, -0.9510565162951536422 ) ) ;
#26793=CARTESIAN_POINT ( 'NONE',  ( 158.6922820468854241, -4.999999999999974243, -32.39392330124607611 ) ) ;
#26795=AXIS2_PLACEMENT_3D ( 'NONE', #3568, #13865, #13016 ) ;
#26798=VERTEX_POINT ( 'NONE', #4272 ) ;
#26802=DIRECTION ( 'NONE',  ( -2.698458740408365879E-16, 1.000000000000000000, 0.000000000000000000 ) ) ;
#26803=DIRECTION ( 'NONE',  ( 1.000000000000000000, 2.168404344971006896E-16, 0.000000000000000000 ) ) ;
#26804=CARTESIAN_POINT ( 'NONE',  ( 131.1922820468854241, -1.999999999999981792, -19.40354224447947118 ) ) ;
#26806=ORIENTED_EDGE ( 'NONE', *, *, #22532, .T. ) ;
#26811=DIRECTION ( 'NONE',  ( 0.9510565162951535312, 2.566386769018988816E-16, -0.3090169943749475623 ) ) ;
#26815=EDGE_LOOP ( 'NONE', ( #10307, #3356, #17688, #16625, #26124 ) ) ;
#26816=LINE ( 'NONE', #6034, #12018 ) ;
#26818=VECTOR ( 'NONE', #22578, 1000.000000000000114 ) ;
#26823=ADVANCED_FACE ( 'NONE', ( #6105 ), #20281, .T. ) ;
#26825=ORIENTED_EDGE ( 'NONE', *, *, #8936, .T. ) ;
#26826=EDGE_CURVE ( 'NONE', #20048, #10103, #22442, .T. ) ;
#26827=CARTESIAN_POINT ( 'NONE',  ( 167.0152310637604387, -9.999999999999998224, 1.702185954127501066 ) ) ;
#26829=ORIENTED_EDGE ( 'NONE', *, *, #17211, .T. ) ;
#26831=CARTESIAN_POINT ( 'NONE',  ( 158.6922820468853956, -1.999999999999973577, -26.58683881228715862 ) ) ;
#26832=CARTESIAN_POINT ( 'NONE',  ( 107.1134392459000395, -4.999999999999988454, -77.82246893306485447 ) ) ;
#26835=DIRECTION ( 'NONE',  ( -0.5877852522924731371, -1.586114251531760235E-16, 0.8090169943749474513 ) ) ;
#26837=VECTOR ( 'NONE', #14142, 1000.000000000000000 ) ;
#26838=CARTESIAN_POINT ( 'NONE',  ( 129.5152310637605524, -10.00000000000000888, -21.71180489736090991 ) ) ;
#26841=CARTESIAN_POINT ( 'NONE',  ( 157.0152310637604387, -4.999999999999975131, -0.06116980274991495881 ) ) ;
#26842=VECTOR ( 'NONE', #1555, 1000.000000000000000 ) ;
#26844=DIRECTION ( 'NONE',  ( 0.3090169943749475623, 8.338696094058001131E-17, 0.9510565162951536422 ) ) ;
#26846=CARTESIAN_POINT ( 'NONE',  ( 158.6922820468853388, -1.999999999999974465, -9.266330736598359152 ) ) ;
#26847=ORIENTED_EDGE ( 'NONE', *, *, #26320, .T. ) ;
#26848=LINE ( 'NONE', #3624, #23691 ) ;
#26850=CARTESIAN_POINT ( 'NONE',  ( 167.0152310637605240, -1.999999999999970912, -24.27857615940569502 ) ) ;
#26851=VERTEX_POINT ( 'NONE', #8835 ) ;
#26852=ORIENTED_EDGE ( 'NONE', *, *, #11440, .T. ) ;
#26853=ORIENTED_EDGE ( 'NONE', *, *, #5049, .T. ) ;
#26858=VECTOR ( 'NONE', #26961, 1000.000000000000000 ) ;
#26860=DIRECTION ( 'NONE',  ( 0.5877852522924731371, 1.586114251531760728E-16, -0.8090169943749474513 ) ) ;
#26861=DIRECTION ( 'NONE',  ( 1.000000000000000000, 2.698458740408365879E-16, -1.110223024625156540E-16 ) ) ;
#26862=LINE ( 'NONE', #12628, #27472 ) ;
#26863=VECTOR ( 'NONE', #25152, 1000.000000000000000 ) ;
#26864=VECTOR ( 'NONE', #30045, 1000.000000000000000 ) ;
#26866=EDGE_CURVE ( 'NONE', #2849, #5527, #27508, .T. ) ;
#26867=CARTESIAN_POINT ( 'NONE',  ( 171.1922820468852819, -1.999999999999971356, -4.936203717676158398 ) ) ;
#26869=DIRECTION ( 'NONE',  ( -0.5877852522924731371, -1.586114251531760235E-16, 0.8090169943749474513 ) ) ;
#26871=DIRECTION ( 'NONE',  ( -0.5877852522924731371, -1.586114251531760728E-16, -0.8090169943749474513 ) ) ;
#26872=VECTOR ( 'NONE', #16898, 999.9999999999998863 ) ;
#26875=VERTEX_POINT ( 'NONE', #6868 ) ;
#26876=AXIS2_PLACEMENT_3D ( 'NONE', #6064, #1048, #10632 ) ;
#26878=ORIENTED_EDGE ( 'NONE', *, *, #8792, .T. ) ;
#26881=FACE_BOUND ( 'NONE', #23363, .T. ) ;
#26883=VERTEX_POINT ( 'NONE', #25778 ) ;
#26884=LINE ( 'NONE', #20269, #12591 ) ;
#26885=ORIENTED_EDGE ( 'NONE', *, *, #22323, .F. ) ;
#26887=CARTESIAN_POINT ( 'NONE',  ( 164.5152310637604955, -9.999999999999998224, -19.94844914048349693 ) ) ;
#26888=ORIENTED_EDGE ( 'NONE', *, *, #9404, .T. ) ;
#26889=LINE ( 'NONE', #10210, #15450 ) ;
#26890=ORIENTED_EDGE ( 'NONE', *, *, #17404, .T. ) ;
#26892=EDGE_CURVE ( 'NONE', #29151, #19118, #444, .T. ) ;
#26893=ORIENTED_EDGE ( 'NONE', *, *, #485, .F. ) ;
#26897=VERTEX_POINT ( 'NONE', #4856 ) ;
#26899=LINE ( 'NONE', #24129, #1866 ) ;
#26900=VERTEX_POINT ( 'NONE', #13856 ) ;
#26901=LINE ( 'NONE', #12508, #2568 ) ;
#26902=VECTOR ( 'NONE', #9383, 1000.000000000000000 ) ;
#26906=ORIENTED_EDGE ( 'NONE', *, *, #9341, .F. ) ;
#26907=CARTESIAN_POINT ( 'NONE',  ( 159.7287565553228603, -4.999999999999974243, 0.8205080756887861426 ) ) ;
#26909=DIRECTION ( 'NONE',  ( 0.000000000000000000, 0.000000000000000000, -1.000000000000000000 ) ) ;
#26910=DIRECTION ( 'NONE',  ( 0.5877852522924731371, 1.586114251531760728E-16, -0.8090169943749474513 ) ) ;
#26912=ORIENTED_EDGE ( 'NONE', *, *, #7405, .T. ) ;
#26914=ORIENTED_EDGE ( 'NONE', *, *, #19998, .T. ) ;
#26916=DIRECTION ( 'NONE',  ( -0.5877852522924731371, 0.000000000000000000, 0.8090169943749474513 ) ) ;
#26919=DIRECTION ( 'NONE',  ( -0.8090169943749474513, -2.183098979609982436E-16, -0.5877852522924731371 ) ) ;
#26922=ORIENTED_EDGE ( 'NONE', *, *, #12759, .T. ) ;
#26923=LINE ( 'NONE', #20016, #1315 ) ;
#26927=EDGE_CURVE ( 'NONE', #8651, #11101, #18452, .T. ) ;
#26932=EDGE_CURVE ( 'NONE', #13701, #7028, #14302, .T. ) ;
#26933=VERTEX_POINT ( 'NONE', #25474 ) ;
#26934=DIRECTION ( 'NONE',  ( -2.698458740408365879E-16, 1.000000000000000000, 0.000000000000000000 ) ) ;
#26935=EDGE_CURVE ( 'NONE', #7167, #27514, #20879, .T. ) ;
#26937=DIRECTION ( 'NONE',  ( -2.698458740408365879E-16, 1.000000000000000000, 0.000000000000000000 ) ) ;
#26938=CARTESIAN_POINT ( 'NONE',  ( 137.2287565553230309, -10.00000000000000533, -29.49038105676660138 ) ) ;
#26939=ORIENTED_EDGE ( 'NONE', *, *, #3644, .T. ) ;
#26943=ORIENTED_EDGE ( 'NONE', *, *, #1109, .T. ) ;
#26944=VERTEX_POINT ( 'NONE', #12019 ) ;
#26945=DIRECTION ( 'NONE',  ( 0.9510565162951536422, 0.000000000000000000, -0.3090169943749475623 ) ) ;
#26947=CARTESIAN_POINT ( 'NONE',  ( 156.1922820468853388, -10.00000000000000178, -2.083034168790677043 ) ) ;
#26948=DIRECTION ( 'NONE',  ( 1.000000000000000000, 2.698458740408365879E-16, -1.110223024625156540E-16 ) ) ;
#26949=PLANE ( 'NONE',  #6309 ) ;
#26950=VECTOR ( 'NONE', #16205, 1000.000000000000000 ) ;
#26955=ORIENTED_EDGE ( 'NONE', *, *, #2938, .F. ) ;
#26956=DIRECTION ( 'NONE',  ( -0.9510565162951536422, -2.566386769018988323E-16, 0.3090169943749475623 ) ) ;
#26958=ORIENTED_EDGE ( 'NONE', *, *, #18976, .T. ) ;
#26960=AXIS2_PLACEMENT_3D ( 'NONE', #6526, #23008, #17952 ) ;
#26961=DIRECTION ( 'NONE',  ( -1.110223024625156540E-16, 0.000000000000000000, -1.000000000000000000 ) ) ;
#26962=DIRECTION ( 'NONE',  ( 0.5877852522924731371, 1.586114251531760728E-16, 0.8090169943749474513 ) ) ;
#26964=ORIENTED_EDGE ( 'NONE', *, *, #18035, .F. ) ;
#26967=ADVANCED_FACE ( 'NONE', ( #144 ), #29794, .T. ) ;
#26970=EDGE_CURVE ( 'NONE', #14514, #24876, #28095, .T. ) ;
#26971=EDGE_CURVE ( 'NONE', #11270, #22429, #2735, .T. ) ;
#26973=LINE ( 'NONE', #6031, #25707 ) ;
#26974=EDGE_CURVE ( 'NONE', #6553, #22761, #9728, .T. ) ;
#26976=VERTEX_POINT ( 'NONE', #21336 ) ;
#26977=DIRECTION ( 'NONE',  ( -0.9510565162951536422, -2.566386769018988816E-16, -0.3090169943749472292 ) ) ;
#26979=VECTOR ( 'NONE', #4575, 1000.000000000000000 ) ;
#26982=AXIS2_PLACEMENT_3D ( 'NONE', #18421, #16428, #16271 ) ;
#26983=DIRECTION ( 'NONE',  ( -2.698458740408365879E-16, 1.000000000000000000, 0.000000000000000000 ) ) ;
#26984=ORIENTED_EDGE ( 'NONE', *, *, #12170, .T. ) ;
#26985=CARTESIAN_POINT ( 'NONE',  ( 5.272361329723610268, -5.000000000000015987, 16.22665966652977332 ) ) ;
#26986=FACE_OUTER_BOUND ( 'NONE', #9459, .T. ) ;
#26987=CARTESIAN_POINT ( 'NONE',  ( 175.7287565553229456, -4.999999999999970690, -2.233642730705313717 ) ) ;
#26988=CARTESIAN_POINT ( 'NONE',  ( 177.2287565553228319, -9.999999999999994671, -3.509618943233403510 ) ) ;
#26993=CARTESIAN_POINT ( 'NONE',  ( 130.7287565553229456, -9.999999999999982236, 3.500000000000003109 ) ) ;
#26995=DIRECTION ( 'NONE',  ( -2.698458740408365879E-16, 1.000000000000000000, 0.000000000000000000 ) ) ;
#27001=ORIENTED_EDGE ( 'NONE', *, *, #5158, .F. ) ;
#27002=CARTESIAN_POINT ( 'NONE',  ( 174.7287565553228887, -9.999999999999994671, -16.50000000000000355 ) ) ;
#27004=ADVANCED_FACE ( 'NONE', ( #14456 ), #9273, .T. ) ;
#27005=EDGE_CURVE ( 'NONE', #3964, #9294, #27952, .T. ) ;
#27007=VECTOR ( 'NONE', #25868, 1000.000000000000000 ) ;
#27008=ORIENTED_EDGE ( 'NONE', *, *, #8413, .F. ) ;
#27009=EDGE_CURVE ( 'NONE', #15637, #15011, #11868, .T. ) ;
#27011=EDGE_CURVE ( 'NONE', #2723, #12166, #16299, .T. ) ;
#27014=ORIENTED_EDGE ( 'NONE', *, *, #28327, .F. ) ;
#27017=CARTESIAN_POINT ( 'NONE',  ( 111.1215651223918144, -4.999999999999986677, -80.73454283993487479 ) ) ;
#27018=DIRECTION ( 'NONE',  ( 0.5877852522924731371, 0.000000000000000000, 0.8090169943749474513 ) ) ;
#27020=VECTOR ( 'NONE', #22144, 1000.000000000000000 ) ;
#27021=EDGE_LOOP ( 'NONE', ( #18128, #12693, #10051, #20689, #11342 ) ) ;
#27022=PLANE ( 'NONE',  #17675 ) ;
#27023=CARTESIAN_POINT ( 'NONE',  ( 167.0152310637604955, -9.999999999999996447, -26.04193191628311155 ) ) ;
#27025=DIRECTION ( 'NONE',  ( 0.9510565162951536422, 0.000000000000000000, -0.3090169943749475623 ) ) ;
#27026=VECTOR ( 'NONE', #9359, 1000.000000000000000 ) ;
#27029=ORIENTED_EDGE ( 'NONE', *, *, #23052, .F. ) ;
#27031=ORIENTED_EDGE ( 'NONE', *, *, #14574, .T. ) ;
#27034=FACE_BOUND ( 'NONE', #5803, .T. ) ;
#27035=VECTOR ( 'NONE', #13703, 1000.000000000000000 ) ;
#27036=EDGE_LOOP ( 'NONE', ( #21463, #5000, #4793, #19250, #25480 ) ) ;
#27037=CARTESIAN_POINT ( 'NONE',  ( 149.5152310637606092, -1.999999999999975353, -28.60870317832789667 ) ) ;
#27038=EDGE_CURVE ( 'NONE', #14791, #5616, #7160, .T. ) ;
#27040=DIRECTION ( 'NONE',  ( 0.3090169943749472292, 8.338696094057992503E-17, -0.9510565162951536422 ) ) ;
#27041=ORIENTED_EDGE ( 'NONE', *, *, #14749, .T. ) ;
#27044=ORIENTED_EDGE ( 'NONE', *, *, #25176, .T. ) ;
#27047=VERTEX_POINT ( 'NONE', #22095 ) ;
#27052=ORIENTED_EDGE ( 'NONE', *, *, #26892, .F. ) ;
#27053=DIRECTION ( 'NONE',  ( -2.698458740408365879E-16, 1.000000000000000000, 0.000000000000000000 ) ) ;
#27055=FACE_OUTER_BOUND ( 'NONE', #26429, .T. ) ;
#27056=CARTESIAN_POINT ( 'NONE',  ( 167.0152310637604955, -9.999999999999996447, -15.61832212156129707 ) ) ;
#27057=ORIENTED_EDGE ( 'NONE', *, *, #16658, .F. ) ;
#27058=EDGE_CURVE ( 'NONE', #23159, #1963, #26700, .T. ) ;
#27059=DIRECTION ( 'NONE',  ( -2.698458740408365879E-16, 1.000000000000000000, 0.000000000000000000 ) ) ;
#27064=PLANE ( 'NONE',  #29574 ) ;
#27065=VECTOR ( 'NONE', #13975, 1000.000000000000000 ) ;
#27068=DIRECTION ( 'NONE',  ( 2.908569913943826047E-16, -1.000000000000000000, 6.826925868028107924E-18 ) ) ;
#27069=ORIENTED_EDGE ( 'NONE', *, *, #3608, .F. ) ;
#27070=LINE ( 'NONE', #24757, #2967 ) ;
#27071=VERTEX_POINT ( 'NONE', #24093 ) ;
#27073=FACE_OUTER_BOUND ( 'NONE', #6422, .T. ) ;
#27074=FACE_OUTER_BOUND ( 'NONE', #19678, .T. ) ;
#27075=EDGE_CURVE ( 'NONE', #27415, #25465, #16907, .T. ) ;
#27076=DIRECTION ( 'NONE',  ( 0.5877852522924731371, 1.586114251531760728E-16, -0.8090169943749474513 ) ) ;
#27077=ORIENTED_EDGE ( 'NONE', *, *, #11949, .F. ) ;
#27081=VERTEX_POINT ( 'NONE', #17354 ) ;
#27088=VECTOR ( 'NONE', #11024, 1000.000000000000000 ) ;
#27090=VERTEX_POINT ( 'NONE', #21795 ) ;
#27091=LINE ( 'NONE', #8574, #23026 ) ;
#27093=CARTESIAN_POINT ( 'NONE',  ( 130.7287565553229456, -4.999999999999983125, 3.500000000000003109 ) ) ;
#27094=VECTOR ( 'NONE', #18880, 1000.000000000000000 ) ;
#27095=ADVANCED_FACE ( 'NONE', ( #23956 ), #5774, .T. ) ;
#27096=DIRECTION ( 'NONE',  ( -2.698458740408365879E-16, 1.000000000000000000, 0.000000000000000000 ) ) ;
#27097=CARTESIAN_POINT ( 'NONE',  ( 144.5152310637605808, -1.999999999999977129, -30.37205893520530964 ) ) ;
#27098=EDGE_CURVE ( 'NONE', #14702, #11968, #29156, .T. ) ;
#27102=CARTESIAN_POINT ( 'NONE',  ( 154.7287565553229172, -10.00000000000000178, 0.8205080756887930260 ) ) ;
#27103=VERTEX_POINT ( 'NONE', #28706 ) ;
#27105=CARTESIAN_POINT ( 'NONE',  ( 172.7287565553229740, -9.999999999999971578, 8.500000000000003553 ) ) ;
#27106=ORIENTED_EDGE ( 'NONE', *, *, #1135, .F. ) ;
#27108=VECTOR ( 'NONE', #29209, 1000.000000000000000 ) ;
#27109=CARTESIAN_POINT ( 'NONE',  ( 133.6922820468854241, -10.00000000000000711, -26.58683881228715506 ) ) ;
#27110=CARTESIAN_POINT ( 'NONE',  ( 14.65125771044925784, -5.000000000000013323, -45.09193465436170101 ) ) ;
#27113=DIRECTION ( 'NONE',  ( -0.9510565162951536422, -2.566386769018988816E-16, -0.3090169943749472292 ) ) ;
#27115=DIRECTION ( 'NONE',  ( -0.5877852522924731371, -1.586114251531760235E-16, 0.8090169943749474513 ) ) ;
#27116=FACE_OUTER_BOUND ( 'NONE', #10843, .T. ) ;
#27120=ORIENTED_EDGE ( 'NONE', *, *, #20617, .T. ) ;
#27122=VECTOR ( 'NONE', #6362, 1000.000000000000000 ) ;
#27123=SURFACE_STYLE_USAGE ( .BOTH. , #4495 ) ;
#27126=VECTOR ( 'NONE', #23625, 1000.000000000000000 ) ;
#27127=ORIENTED_EDGE ( 'NONE', *, *, #23808, .F. ) ;
#27129=VECTOR ( 'NONE', #27113, 1000.000000000000000 ) ;
#27130=DIRECTION ( 'NONE',  ( 0.9510565162951535312, 2.566386769018988816E-16, -0.3090169943749475623 ) ) ;
#27133=LINE ( 'NONE', #19544, #3335 ) ;
#27134=EDGE_CURVE ( 'NONE', #12148, #7328, #19641, .T. ) ;
#27136=EDGE_CURVE ( 'NONE', #3561, #19213, #10482, .T. ) ;
#27139=CARTESIAN_POINT ( 'NONE',  ( 134.5152310637605808, -10.00000000000000533, -28.60870317832789311 ) ) ;
#27143=VECTOR ( 'NONE', #22695, 1000.000000000000000 ) ;
#27144=CARTESIAN_POINT ( 'NONE',  ( 168.6922820468853388, -4.999999999999972466, -17.92658477444275889 ) ) ;
#27148=VERTEX_POINT ( 'NONE', #10333 ) ;
#27149=DIRECTION ( 'NONE',  ( 2.908569913943825554E-16, -1.000000000000000000, 0.000000000000000000 ) ) ;
#27152=VECTOR ( 'NONE', #22153, 1000.000000000000000 ) ;
#27153=CARTESIAN_POINT ( 'NONE',  ( 146.1922820468854525, -1.999999999999977129, -30.91696583120935671 ) ) ;
#27154=FACE_OUTER_BOUND ( 'NONE', #2637, .T. ) ;
#27156=FACE_OUTER_BOUND ( 'NONE', #25992, .T. ) ;
#27157=ORIENTED_EDGE ( 'NONE', *, *, #16690, .F. ) ;
#27158=EDGE_LOOP ( 'NONE', ( #22604, #22772, #2333, #29230 ) ) ;
#27161=VERTEX_POINT ( 'NONE', #17506 ) ;
#27164=CARTESIAN_POINT ( 'NONE',  ( 104.5764801505170851, -4.999999999999988454, -75.97926025845912079 ) ) ;
#27165=PLANE ( 'NONE',  #24819 ) ;
#27166=LINE ( 'NONE', #4235, #11810 ) ;
#27168=ADVANCED_FACE ( 'NONE', ( #24243 ), #9881, .T. ) ;
#27170=EDGE_CURVE ( 'NONE', #29723, #6582, #5927, .T. ) ;
#27171=EDGE_LOOP ( 'NONE', ( #13911, #5584, #10676, #1920 ) ) ;
#27172=DIRECTION ( 'NONE',  ( -2.698458740408365879E-16, 1.000000000000000000, 0.000000000000000000 ) ) ;
#27173=EDGE_LOOP ( 'NONE', ( #25651, #4145, #1903, #17814 ) ) ;
#27174=LINE ( 'NONE', #13388, #17998 ) ;
#27175=AXIS2_PLACEMENT_3D ( 'NONE', #17830, #25173, #15393 ) ;
#27176=ORIENTED_EDGE ( 'NONE', *, *, #13073, .F. ) ;
#27177=EDGE_CURVE ( 'NONE', #21061, #17086, #3194, .T. ) ;
#27179=VECTOR ( 'NONE', #299, 999.9999999999998863 ) ;
#27180=FACE_OUTER_BOUND ( 'NONE', #26231, .T. ) ;
#27181=ADVANCED_FACE ( 'NONE', ( #19343 ), #3632, .T. ) ;
#27182=EDGE_CURVE ( 'NONE', #29771, #29222, #3343, .T. ) ;
#27183=ORIENTED_EDGE ( 'NONE', *, *, #16870, .F. ) ;
#27184=ADVANCED_FACE ( 'NONE', ( #19193 ), #10028, .T. ) ;
#27187=VECTOR ( 'NONE', #27549, 1000.000000000000000 ) ;
#27188=VERTEX_POINT ( 'NONE', #14755 ) ;
#27190=ORIENTED_EDGE ( 'NONE', *, *, #8991, .F. ) ;
#27193=CARTESIAN_POINT ( 'NONE',  ( 176.1922820468852535, -1.999999999999970024, -4.936203717676158398 ) ) ;
#27194=ORIENTED_EDGE ( 'NONE', *, *, #7321, .T. ) ;
#27195=LINE ( 'NONE', #12805, #6129 ) ;
#27198=CARTESIAN_POINT ( 'NONE',  ( 151.1922820468854525, -10.00000000000000178, -30.91696583120936026 ) ) ;
#27199=ORIENTED_EDGE ( 'NONE', *, *, #21041, .T. ) ;
#27200=VERTEX_POINT ( 'NONE', #894 ) ;
#27201=CARTESIAN_POINT ( 'NONE',  ( 168.6922820468853672, -9.999999999999996447, -26.58683881228715862 ) ) ;
#27202=ORIENTED_EDGE ( 'NONE', *, *, #9126, .T. ) ;
#27208=ORIENTED_EDGE ( 'NONE', *, *, #27730, .T. ) ;
#27209=FACE_OUTER_BOUND ( 'NONE', #22230, .T. ) ;
#27211=VERTEX_POINT ( 'NONE', #21944 ) ;
#27215=EDGE_CURVE ( 'NONE', #10352, #13853, #10185, .T. ) ;
#27216=VECTOR ( 'NONE', #1223, 1000.000000000000000 ) ;
#27217=ORIENTED_EDGE ( 'NONE', *, *, #18172, .T. ) ;
#27218=EDGE_CURVE ( 'NONE', #6733, #18145, #12625, .T. ) ;
#27219=EDGE_CURVE ( 'NONE', #8035, #23347, #8798, .T. ) ;
#27222=DIRECTION ( 'NONE',  ( 0.3090169943749472292, 8.338696094057992503E-17, -0.9510565162951536422 ) ) ;
#27223=VECTOR ( 'NONE', #26008, 1000.000000000000000 ) ;
#27224=VERTEX_POINT ( 'NONE', #8353 ) ;
#27225=EDGE_LOOP ( 'NONE', ( #3504, #10693, #11788, #12426 ) ) ;
#27226=CARTESIAN_POINT ( 'NONE',  ( 172.0152310637604671, -9.999999999999994671, -15.61832212156129707 ) ) ;
#27229=ORIENTED_EDGE ( 'NONE', *, *, #7364, .F. ) ;
#27230=DIRECTION ( 'NONE',  ( -0.5877852522924731371, 0.000000000000000000, 0.8090169943749474513 ) ) ;
#27232=PLANE ( 'NONE',  #9778 ) ;
#27233=LINE ( 'NONE', #22769, #18386 ) ;
#27234=ORIENTED_EDGE ( 'NONE', *, *, #19233, .F. ) ;
#27236=ORIENTED_EDGE ( 'NONE', *, *, #23014, .F. ) ;
#27242=AXIS2_PLACEMENT_3D ( 'NONE', #322, #13180, #1606 ) ;
#27243=CARTESIAN_POINT ( 'NONE',  ( 174.7287565553228319, -1.999999999999970024, 0.8205080756887930260 ) ) ;
#27244=LINE ( 'NONE', #1273, #19440 ) ;
#27245=PLANE ( 'NONE',  #24222 ) ;
#27246=EDGE_CURVE ( 'NONE', #1088, #18037, #8502, .T. ) ;
#27249=VECTOR ( 'NONE', #1425, 1000.000000000000000 ) ;
#27252=ORIENTED_EDGE ( 'NONE', *, *, #22670, .F. ) ;
#27253=FACE_OUTER_BOUND ( 'NONE', #11743, .T. ) ;
#27254=PLANE ( 'NONE',  #9188 ) ;
#27256=EDGE_CURVE ( 'NONE', #7125, #29656, #3788, .T. ) ;
#27258=FACE_OUTER_BOUND ( 'NONE', #21171, .T. ) ;
#27259=DIRECTION ( 'NONE',  ( 0.3090169943749475623, 8.338696094058001131E-17, 0.9510565162951536422 ) ) ;
#27260=VECTOR ( 'NONE', #10815, 1000.000000000000000 ) ;
#27265=EDGE_LOOP ( 'NONE', ( #10657, #7634, #24641, #17241 ) ) ;
#27268=DIRECTION ( 'NONE',  ( -2.698458740408366372E-16, 1.000000000000000000, 0.000000000000000000 ) ) ;
#27269=ORIENTED_EDGE ( 'NONE', *, *, #18942, .T. ) ;
#27271=DIRECTION ( 'NONE',  ( -2.698458740408365879E-16, 1.000000000000000000, 0.000000000000000000 ) ) ;
#27272=CARTESIAN_POINT ( 'NONE',  ( 159.5152310637604955, -9.999999999999998224, -21.71180489736091346 ) ) ;
#27273=LINE ( 'NONE', #16063, #16662 ) ;
#27275=EDGE_LOOP ( 'NONE', ( #25952, #13276, #4664, #13935 ) ) ;
#27277=ORIENTED_EDGE ( 'NONE', *, *, #11861, .T. ) ;
#27278=CARTESIAN_POINT ( 'NONE',  ( 164.5152310637604671, -1.999999999999972244, -13.05155085951651195 ) ) ;
#27281=CARTESIAN_POINT ( 'NONE',  ( 164.7287565553228887, -9.999999999999998224, 0.8205080756887930260 ) ) ;
#27283=CARTESIAN_POINT ( 'NONE',  ( 148.6922820468853956, -10.00000000000000178, -6.413161187712876909 ) ) ;
#27285=EDGE_LOOP ( 'NONE', ( #3300, #8866, #27983, #20425, #27349 ) ) ;
#27286=CARTESIAN_POINT ( 'NONE',  ( 137.2287565553230309, -4.999999999999980460, -20.83012701892219454 ) ) ;
#27287=EDGE_CURVE ( 'NONE', #18174, #3603, #20104, .T. ) ;
#27289=EDGE_CURVE ( 'NONE', #27662, #3793, #10642, .T. ) ;
#27291=ORIENTED_EDGE ( 'NONE', *, *, #17916, .T. ) ;
#27293=VECTOR ( 'NONE', #19293, 1000.000000000000000 ) ;
#27295=FACE_OUTER_BOUND ( 'NONE', #27790, .T. ) ;
#27296=AXIS2_PLACEMENT_3D ( 'NONE', #23645, #12181, #2744 ) ;
#27297=LINE ( 'NONE', #26985, #26326 ) ;
#27298=CARTESIAN_POINT ( 'NONE',  ( 17.99346030888765924, -5.000000000000012434, -55.37817656947992617 ) ) ;
#27299=CARTESIAN_POINT ( 'NONE',  ( 129.5152310637605524, -10.00000000000000888, -4.391296821672111328 ) ) ;
#27300=PLANE ( 'NONE',  #29739 ) ;
#27305=DIRECTION ( 'NONE',  ( 6.938893903907227392E-16, -0.000000000000000000, 1.000000000000000000 ) ) ;
#27307=PLANE ( 'NONE',  #25407 ) ;
#27308=CARTESIAN_POINT ( 'NONE',  ( 162.0152310637604387, -4.999999999999974243, -8.721423840594312082 ) ) ;
#27310=CARTESIAN_POINT ( 'NONE',  ( 24.67409968758932237, -5.000000000000010658, -75.93907040311476919 ) ) ;
#27311=CARTESIAN_POINT ( 'NONE',  ( 149.5152310637605240, -4.999999999999976907, -2.627941064794695691 ) ) ;
#27313=ORIENTED_EDGE ( 'NONE', *, *, #26147, .T. ) ;
#27315=LINE ( 'NONE', #17793, #11463 ) ;
#27316=CARTESIAN_POINT ( 'NONE',  ( 134.5152310637605524, -10.00000000000000533, -13.05155085951650840 ) ) ;
#27317=CARTESIAN_POINT ( 'NONE',  ( 162.0152310637604955, -9.999999999999998224, -26.04193191628311155 ) ) ;
#27318=VECTOR ( 'NONE', #11694, 1000.000000000000000 ) ;
#27322=EDGE_CURVE ( 'NONE', #6582, #4252, #20247, .T. ) ;
#27323=EDGE_CURVE ( 'NONE', #18221, #4117, #13240, .T. ) ;
#27327=CARTESIAN_POINT ( 'NONE',  ( 154.5152310637605524, -1.999999999999974021, -30.37205893520531319 ) ) ;
#27328=ADVANCED_FACE ( 'NONE', ( #13082 ), #24851, .T. ) ;
#27329=CARTESIAN_POINT ( 'NONE',  ( 149.5152310637605808, -10.00000000000000178, -19.94844914048349693 ) ) ;
#27331=ORIENTED_EDGE ( 'NONE', *, *, #16939, .F. ) ;
#27332=CARTESIAN_POINT ( 'NONE',  ( 167.0152310637604671, -1.999999999999971800, -6.958068083716895558 ) ) ;
#27334=EDGE_LOOP ( 'NONE', ( #25622, #29214, #11015, #1600 ) ) ;
#27337=CARTESIAN_POINT ( 'NONE',  ( 172.2287565553228887, -1.999999999999970024, -12.16987298107780369 ) ) ;
#27338=VECTOR ( 'NONE', #19924, 1000.000000000000000 ) ;
#27339=LINE ( 'NONE', #13393, #25355 ) ;
#27341=ORIENTED_EDGE ( 'NONE', *, *, #14203, .T. ) ;
#27347=CARTESIAN_POINT ( 'NONE',  ( 154.5152310637604955, -1.999999999999975353, -2.627941064794695691 ) ) ;
#27349=ORIENTED_EDGE ( 'NONE', *, *, #16999, .T. ) ;
#27351=DIRECTION ( 'NONE',  ( -2.698458740408365879E-16, 1.000000000000000000, 0.000000000000000000 ) ) ;
#27352=CARTESIAN_POINT ( 'NONE',  ( 125.7287565553229172, -4.000000000000003553, -33.50000000000000000 ) ) ;
#27353=DIRECTION ( 'NONE',  ( -0.9510565162951536422, 0.000000000000000000, -0.3090169943749472292 ) ) ;
#27354=DIRECTION ( 'NONE',  ( 0.5877852522924731371, 1.586114251531760728E-16, -0.8090169943749474513 ) ) ;
#27355=EDGE_LOOP ( 'NONE', ( #24902, #4746, #5703, #27236 ) ) ;
#27357=VECTOR ( 'NONE', #8634, 1000.000000000000000 ) ;
#27360=EDGE_CURVE ( 'NONE', #21077, #20122, #1509, .T. ) ;
#27361=VECTOR ( 'NONE', #15177, 1000.000000000000000 ) ;
#27362=CARTESIAN_POINT ( 'NONE',  ( 176.1922820468852819, -9.999999999999994671, -13.59645775552055902 ) ) ;
#27364=DIRECTION ( 'NONE',  ( -2.698458740408365879E-16, 1.000000000000000000, 0.000000000000000000 ) ) ;
#27367=EDGE_LOOP ( 'NONE', ( #2252, #12782, #9525, #18636 ) ) ;
#27369=VECTOR ( 'NONE', #5004, 999.9999999999998863 ) ;
#27370=CARTESIAN_POINT ( 'NONE',  ( 147.2287565553230024, -1.999999999999976685, -12.16987298107780369 ) ) ;
#27375=DIRECTION ( 'NONE',  ( -2.698458740408365879E-16, 1.000000000000000000, 0.000000000000000000 ) ) ;
#27377=ORIENTED_EDGE ( 'NONE', *, *, #16004, .F. ) ;
#27378=CARTESIAN_POINT ( 'NONE',  ( 14.41923689471965808, -5.000000000000014211, 44.37784800950869624 ) ) ;
#27385=LINE ( 'NONE', #1566, #20999 ) ;
#27387=EDGE_LOOP ( 'NONE', ( #2197, #13633, #13586, #8254 ) ) ;
#27388=ORIENTED_EDGE ( 'NONE', *, *, #14397, .F. ) ;
#27389=DIRECTION ( 'NONE',  ( -0.5877852522924731371, -1.586114251531760728E-16, -0.8090169943749474513 ) ) ;
#27392=AXIS2_PLACEMENT_3D ( 'NONE', #26373, #19624, #12606 ) ;
#27396=EDGE_CURVE ( 'NONE', #475, #2286, #4087, .T. ) ;
#27397=ADVANCED_FACE ( 'NONE', ( #1354 ), #19952, .T. ) ;
#27400=FACE_OUTER_BOUND ( 'NONE', #1045, .T. ) ;
#27403=ORIENTED_EDGE ( 'NONE', *, *, #6879, .T. ) ;
#27406=CARTESIAN_POINT ( 'NONE',  ( 169.5152310637604671, -1.999999999999970468, -21.71180489736091346 ) ) ;
#27407=DIRECTION ( 'NONE',  ( -2.698458740408365879E-16, 1.000000000000000000, 0.000000000000000000 ) ) ;
#27408=VECTOR ( 'NONE', #6818, 1000.000000000000000 ) ;
#27412=CARTESIAN_POINT ( 'NONE',  ( 172.0152310637604955, -1.999999999999969358, -34.70218595412750773 ) ) ;
#27413=ORIENTED_EDGE ( 'NONE', *, *, #1515, .F. ) ;
#27414=CARTESIAN_POINT ( 'NONE',  ( 174.7287565553228603, -1.999999999999969580, -7.839745962155603820 ) ) ;
#27415=VERTEX_POINT ( 'NONE', #15301 ) ;
#27417=LINE ( 'NONE', #25805, #16461 ) ;
#27419=CARTESIAN_POINT ( 'NONE',  ( 167.0152310637604671, -1.999999999999971356, -17.38167787843871182 ) ) ;
#27420=DIRECTION ( 'NONE',  ( -0.9510565162951536422, -2.566386769018988816E-16, -0.3090169943749472292 ) ) ;
#27422=VERTEX_POINT ( 'NONE', #19442 ) ;
#27423=ORIENTED_EDGE ( 'NONE', *, *, #16348, .F. ) ;
#27424=DIRECTION ( 'NONE',  ( 0.9510565162951536422, 2.566386769018988816E-16, 0.3090169943749472292 ) ) ;
#27427=LINE ( 'NONE', #22356, #28875 ) ;
#27429=DIRECTION ( 'NONE',  ( -2.698458740408365879E-16, 1.000000000000000000, 0.000000000000000000 ) ) ;
#27432=ORIENTED_EDGE ( 'NONE', *, *, #4643, .F. ) ;
#27433=ADVANCED_FACE ( 'NONE', ( #839 ), #24633, .T. ) ;
#27434=DIRECTION ( 'NONE',  ( -0.5877852522924731371, -1.586114251531760235E-16, 0.8090169943749474513 ) ) ;
#27437=ORIENTED_EDGE ( 'NONE', *, *, #11830, .T. ) ;
#27438=LINE ( 'NONE', #11354, #4887 ) ;
#27440=AXIS2_PLACEMENT_3D ( 'NONE', #537, #17292, #26945 ) ;
#27441=DIRECTION ( 'NONE',  ( -0.9510565162951536422, 0.000000000000000000, -0.3090169943749472292 ) ) ;
#27442=VERTEX_POINT ( 'NONE', #10584 ) ;
#27443=LINE ( 'NONE', #20078, #15095 ) ;
#27444=DIRECTION ( 'NONE',  ( -2.698458740408365879E-16, 1.000000000000000000, 0.000000000000000000 ) ) ;
#27445=CARTESIAN_POINT ( 'NONE',  ( 16.00468163665589572, -5.000000000000013323, -49.25734519086697105 ) ) ;
#27450=EDGE_CURVE ( 'NONE', #28182, #17358, #24336, .T. ) ;
#27452=ORIENTED_EDGE ( 'NONE', *, *, #307, .F. ) ;
#27453=DIRECTION ( 'NONE',  ( -2.698458740408365879E-16, 1.000000000000000000, 0.000000000000000000 ) ) ;
#27456=LINE ( 'NONE', #3769, #6392 ) ;
#27457=LINE ( 'NONE', #6507, #23670 ) ;
#27459=DIRECTION ( 'NONE',  ( -0.9510565162951536422, -2.566386769018988816E-16, -0.3090169943749472292 ) ) ;
#27460=EDGE_LOOP ( 'NONE', ( #21297, #7922, #14823, #19153 ) ) ;
#27461=CARTESIAN_POINT ( 'NONE',  ( 143.6922820468853956, -4.999999999999978684, 2.247092850131519715 ) ) ;
#27465=DIRECTION ( 'NONE',  ( 0.5877852522924731371, 1.586114251531760728E-16, 0.8090169943749474513 ) ) ;
#27466=CARTESIAN_POINT ( 'NONE',  ( 137.0152310637605524, -10.00000000000000533, -0.06116980274991495881 ) ) ;
#27467=ORIENTED_EDGE ( 'NONE', *, *, #5676, .F. ) ;
#27472=VECTOR ( 'NONE', #29158, 1000.000000000000000 ) ;
#27473=LINE ( 'NONE', #27769, #15712 ) ;
#27475=EDGE_LOOP ( 'NONE', ( #18029, #4147, #3887, #18919 ) ) ;
#27476=CARTESIAN_POINT ( 'NONE',  ( 15.60617273857451615, -5.000000000000013323, -48.03086091582405714 ) ) ;
#27479=CARTESIAN_POINT ( 'NONE',  ( 169.5152310637604955, -4.999999999999971578, -19.94844914048349693 ) ) ;
#27481=LINE ( 'NONE', #20855, #5859 ) ;
#27482=EDGE_CURVE ( 'NONE', #28787, #26475, #12569, .T. ) ;
#27483=EDGE_CURVE ( 'NONE', #4938, #12612, #3730, .T. ) ;
#27485=ORIENTED_EDGE ( 'NONE', *, *, #2008, .T. ) ;
#27487=EDGE_CURVE ( 'NONE', #24460, #14791, #19890, .T. ) ;
#27488=EDGE_LOOP ( 'NONE', ( #1090, #29001, #17391, #18634 ) ) ;
#27489=AXIS2_PLACEMENT_3D ( 'NONE', #23015, #13538, #4678 ) ;
#27490=DIRECTION ( 'NONE',  ( 0.9510565162951536422, 2.566386769018988816E-16, 0.3090169943749472292 ) ) ;
#27493=DIRECTION ( 'NONE',  ( 1.110223024625156540E-16, 2.995891024602366092E-32, 1.000000000000000000 ) ) ;
#27494=ORIENTED_EDGE ( 'NONE', *, *, #9715, .T. ) ;
#27495=ORIENTED_EDGE ( 'NONE', *, *, #3108, .F. ) ;
#27496=FACE_OUTER_BOUND ( 'NONE', #10471, .T. ) ;
#27498=LINE ( 'NONE', #19763, #19360 ) ;
#27499=ORIENTED_EDGE ( 'NONE', *, *, #9715, .F. ) ;
#27500=ORIENTED_EDGE ( 'NONE', *, *, #17246, .T. ) ;
#27501=LINE ( 'NONE', #19980, #12501 ) ;
#27502=ORIENTED_EDGE ( 'NONE', *, *, #6640, .F. ) ;
#27508=LINE ( 'NONE', #15850, #3340 ) ;
#27509=CARTESIAN_POINT ( 'NONE',  ( 161.1922820468853956, -9.999999999999998224, -30.91696583120936026 ) ) ;
#27511=VECTOR ( 'NONE', #987, 1000.000000000000000 ) ;
#27512=CARTESIAN_POINT ( 'NONE',  ( 166.1922820468853104, -9.999999999999998224, -4.936203717676158398 ) ) ;
#27513=DIRECTION ( 'NONE',  ( 0.5877852522924731371, 0.000000000000000000, 0.8090169943749474513 ) ) ;
#27514=VERTEX_POINT ( 'NONE', #24047 ) ;
#27515=DIRECTION ( 'NONE',  ( -0.5877852522924731371, -1.586114251531760728E-16, -0.8090169943749474513 ) ) ;
#27517=CARTESIAN_POINT ( 'NONE',  ( 134.7287565553230024, -10.00000000000000711, -7.839745962155602044 ) ) ;
#27519=ORIENTED_EDGE ( 'NONE', *, *, #26970, .F. ) ;
#27520=EDGE_CURVE ( 'NONE', #15766, #28338, #15153, .T. ) ;
#27521=ORIENTED_EDGE ( 'NONE', *, *, #28913, .T. ) ;
#27522=DIRECTION ( 'NONE',  ( -0.9510565162951536422, -2.566386769018988323E-16, 0.3090169943749475623 ) ) ;
#27523=ADVANCED_FACE ( 'NONE', ( #7851 ), #12722, .T. ) ;
#27528=DIRECTION ( 'NONE',  ( -1.110223024625156540E-16, 0.000000000000000000, -1.000000000000000000 ) ) ;
#27529=VECTOR ( 'NONE', #16916, 1000.000000000000000 ) ;
#27531=CARTESIAN_POINT ( 'NONE',  ( 137.2287565553230309, -1.999999999999979572, -12.16987298107780013 ) ) ;
#27532=DIRECTION ( 'NONE',  ( 6.938893903907227392E-16, -0.000000000000000000, 1.000000000000000000 ) ) ;
#27533=EDGE_LOOP ( 'NONE', ( #4834, #2700, #23671, #22870 ) ) ;
#27534=DIRECTION ( 'NONE',  ( 0.5877852522924731371, 0.000000000000000000, 0.8090169943749474513 ) ) ;
#27539=ORIENTED_EDGE ( 'NONE', *, *, #9796, .T. ) ;
#27541=LINE ( 'NONE', #33, #6454 ) ;
#27545=ORIENTED_EDGE ( 'NONE', *, *, #7774, .T. ) ;
#27546=DIRECTION ( 'NONE',  ( -2.698458740408365879E-16, 1.000000000000000000, 0.000000000000000000 ) ) ;
#27547=VECTOR ( 'NONE', #6499, 1000.000000000000000 ) ;
#27548=ORIENTED_EDGE ( 'NONE', *, *, #13147, .T. ) ;
#27549=DIRECTION ( 'NONE',  ( -0.5877852522924731371, -1.586114251531760235E-16, 0.8090169943749474513 ) ) ;
#27551=EDGE_CURVE ( 'NONE', #16634, #6979, #3582, .T. ) ;
#27553=ADVANCED_FACE ( 'NONE', ( #8143 ), #29261, .T. ) ;
#27554=EDGE_CURVE ( 'NONE', #13154, #22282, #3145, .T. ) ;
#27556=EDGE_CURVE ( 'NONE', #22891, #28379, #28813, .T. ) ;
#27558=ORIENTED_EDGE ( 'NONE', *, *, #897, .T. ) ;
#27559=PLANE ( 'NONE',  #12002 ) ;
#27560=EDGE_LOOP ( 'NONE', ( #3927, #8169, #7541, #29190 ) ) ;
#27563=PLANE ( 'NONE',  #11709 ) ;
#27564=DIRECTION ( 'NONE',  ( -0.9510565162951536422, -2.566386769018988323E-16, 0.3090169943749475623 ) ) ;
#27567=PLANE ( 'NONE',  #18344 ) ;
#27570=CARTESIAN_POINT ( 'NONE',  ( 156.1922820468853672, -10.00000000000000000, -13.59645775552055902 ) ) ;
#27581=LINE ( 'NONE', #6637, #532 ) ;
#27582=DIRECTION ( 'NONE',  ( -0.9510565162951536422, -2.566386769018988323E-16, 0.3090169943749475623 ) ) ;
#27585=EDGE_CURVE ( 'NONE', #16407, #9840, #14848, .T. ) ;
#27586=DIRECTION ( 'NONE',  ( -2.698458740408365879E-16, 1.000000000000000000, 0.000000000000000000 ) ) ;
#27587=AXIS2_PLACEMENT_3D ( 'NONE', #15866, #11294, #14020 ) ;
#27588=EDGE_CURVE ( 'NONE', #12381, #25113, #11567, .T. ) ;
#27589=CARTESIAN_POINT ( 'NONE',  ( 174.5152310637604955, -9.999999999999994671, -28.60870317832789667 ) ) ;
#27597=DIRECTION ( 'NONE',  ( 1.000000000000000000, 2.698458740408365879E-16, -1.110223024625156540E-16 ) ) ;
#27600=ORIENTED_EDGE ( 'NONE', *, *, #9446, .F. ) ;
#27601=CARTESIAN_POINT ( 'NONE',  ( 125.7287565553229456, -9.999999999999994671, 0.5000000000000143219 ) ) ;
#27603=VECTOR ( 'NONE', #28655, 1000.000000000000000 ) ;
#27605=CARTESIAN_POINT ( 'NONE',  ( 154.5152310637605524, -10.00000000000000000, -30.37205893520531319 ) ) ;
#27606=DIRECTION ( 'NONE',  ( 0.5877852522924731371, 1.586114251531760728E-16, -0.8090169943749474513 ) ) ;
#27607=CARTESIAN_POINT ( 'NONE',  ( 139.5152310637605808, -1.999999999999978684, -13.05155085951651195 ) ) ;
#27608=ORIENTED_EDGE ( 'NONE', *, *, #16347, .T. ) ;
#27612=VECTOR ( 'NONE', #3252, 1000.000000000000000 ) ;
#27617=EDGE_CURVE ( 'NONE', #22145, #12691, #16498, .T. ) ;
#27619=ORIENTED_EDGE ( 'NONE', *, *, #26253, .T. ) ;
#27621=CARTESIAN_POINT ( 'NONE',  ( 144.7287565553230309, -1.999999999999977129, -16.50000000000000355 ) ) ;
#27622=ORIENTED_EDGE ( 'NONE', *, *, #14651, .F. ) ;
#27623=LINE ( 'NONE', #6689, #10919 ) ;
#27624=VECTOR ( 'NONE', #15390, 1000.000000000000000 ) ;
#27625=CARTESIAN_POINT ( 'NONE',  ( 175.7287565553229456, -4.999999999999970690, 3.500000000000003109 ) ) ;
#27627=VECTOR ( 'NONE', #12131, 1000.000000000000000 ) ;
#27630=VECTOR ( 'NONE', #8442, 1000.000000000000000 ) ;
#27632=CARTESIAN_POINT ( 'NONE',  ( 137.0152310637605808, -4.999999999999980460, -1.521174642513229767E-14 ) ) ;
#27635=CARTESIAN_POINT ( 'NONE',  ( 137.0152310637605524, -10.00000000000000533, -0.06116980274991495881 ) ) ;
#27636=ORIENTED_EDGE ( 'NONE', *, *, #3640, .T. ) ;
#27637=DIRECTION ( 'NONE',  ( 0.5877852522924731371, 1.586114251531760728E-16, 0.8090169943749474513 ) ) ;
#27639=EDGE_LOOP ( 'NONE', ( #7271, #16430, #24416, #27838, #20320 ) ) ;
#27640=VERTEX_POINT ( 'NONE', #4954 ) ;
#27641=DIRECTION ( 'NONE',  ( 1.000000000000000000, 2.698458740408365879E-16, -1.110223024625156540E-16 ) ) ;
#27642=ORIENTED_EDGE ( 'NONE', *, *, #26974, .T. ) ;
#27649=DIRECTION ( 'NONE',  ( -0.8090169943749474513, -2.183098979609982436E-16, 0.5877852522924731371 ) ) ;
#27650=EDGE_CURVE ( 'NONE', #20619, #3306, #21273, .T. ) ;
#27651=EDGE_CURVE ( 'NONE', #5801, #21069, #26027, .T. ) ;
#27653=EDGE_CURVE ( 'NONE', #22172, #11987, #5410, .T. ) ;
#27656=VECTOR ( 'NONE', #8770, 1000.000000000000000 ) ;
#27657=LINE ( 'NONE', #18907, #21270 ) ;
#27658=DIRECTION ( 'NONE',  ( -2.698458740408365879E-16, 1.000000000000000000, 0.000000000000000000 ) ) ;
#27660=LINE ( 'NONE', #25191, #16476 ) ;
#27661=CARTESIAN_POINT ( 'NONE',  ( 133.7287565553229456, -4.999999999999982236, 0.5000000000000029976 ) ) ;
#27662=VERTEX_POINT ( 'NONE', #2671 ) ;
#27663=ORIENTED_EDGE ( 'NONE', *, *, #12409, .F. ) ;
#27664=DIRECTION ( 'NONE',  ( -0.9510565162951536422, 0.000000000000000000, -0.3090169943749472292 ) ) ;
#27669=ORIENTED_EDGE ( 'NONE', *, *, #28327, .T. ) ;
#27670=ORIENTED_EDGE ( 'NONE', *, *, #307, .T. ) ;
#27671=ORIENTED_EDGE ( 'NONE', *, *, #15559, .T. ) ;
#27672=AXIS2_PLACEMENT_3D ( 'NONE', #176, #5040, #23 ) ;
#27674=VECTOR ( 'NONE', #17790, 1000.000000000000000 ) ;
#27676=DIRECTION ( 'NONE',  ( -0.7071067811865481278, 0.7071067811865469066, 0.000000000000000000 ) ) ;
#27677=DIRECTION ( 'NONE',  ( 1.000000000000000000, 2.698458740408365879E-16, -1.110223024625156540E-16 ) ) ;
#27678=VERTEX_POINT ( 'NONE', #28641 ) ;
#27680=ORIENTED_EDGE ( 'NONE', *, *, #5812, .F. ) ;
#27682=AXIS2_PLACEMENT_3D ( 'NONE', #29413, #24625, #15603 ) ;
#27685=ORIENTED_EDGE ( 'NONE', *, *, #23050, .F. ) ;
#27686=ORIENTED_EDGE ( 'NONE', *, *, #24775, .T. ) ;
#27687=PLANE ( 'NONE',  #4784 ) ;
#27688=CARTESIAN_POINT ( 'NONE',  ( 149.7287565553229740, -10.00000000000000178, -7.839745962155603820 ) ) ;
#27689=ORIENTED_EDGE ( 'NONE', *, *, #10346, .F. ) ;
#27690=EDGE_CURVE ( 'NONE', #23715, #28996, #9970, .T. ) ;
#27691=EDGE_CURVE ( 'NONE', #13196, #5499, #831, .T. ) ;
#27693=ADVANCED_FACE ( 'NONE', ( #19283 ), #14696, .T. ) ;
#27696=EDGE_CURVE ( 'NONE', #288, #16032, #10121, .T. ) ;
#27697=ORIENTED_EDGE ( 'NONE', *, *, #13347, .T. ) ;
#27698=FACE_OUTER_BOUND ( 'NONE', #21540, .T. ) ;
#27699=VECTOR ( 'NONE', #4636, 1000.000000000000000 ) ;
#27702=DIRECTION ( 'NONE',  ( -0.5877852522924731371, -1.586114251531760235E-16, 0.8090169943749474513 ) ) ;
#27707=CARTESIAN_POINT ( 'NONE',  ( 157.0152310637605808, -9.999999999999998224, -32.93883019725009120 ) ) ;
#27708=ORIENTED_EDGE ( 'NONE', *, *, #21164, .T. ) ;
#27710=AXIS2_PLACEMENT_3D ( 'NONE', #29131, #10308, #1480 ) ;
#27712=LINE ( 'NONE', #57, #14622 ) ;
#27715=ORIENTED_EDGE ( 'NONE', *, *, #14200, .T. ) ;
#27717=CARTESIAN_POINT ( 'NONE',  ( 89.30687414754424935, -4.999999999999992895, 64.88524211141340459 ) ) ;
#27724=ORIENTED_EDGE ( 'NONE', *, *, #19578, .T. ) ;
#27725=CARTESIAN_POINT ( 'NONE',  ( 132.0152310637605808, -10.00000000000000711, -32.93883019725009120 ) ) ;
#27726=( NAMED_UNIT ( * ) PLANE_ANGLE_UNIT ( ) SI_UNIT ( $, .RADIAN. ) );
#27727=VECTOR ( 'NONE', #25672, 1000.000000000000000 ) ;
#27730=EDGE_CURVE ( 'NONE', #11670, #2626, #2539, .T. ) ;
#27731=EDGE_CURVE ( 'NONE', #2212, #5854, #14243, .T. ) ;
#27732=EDGE_CURVE ( 'NONE', #28465, #16324, #14390, .T. ) ;
#27734=DIRECTION ( 'NONE',  ( -2.698458740408365879E-16, 1.000000000000000000, 0.000000000000000000 ) ) ;
#27735=VECTOR ( 'NONE', #11038, 1000.000000000000000 ) ;
#27736=LINE ( 'NONE', #14087, #13317 ) ;
#27737=PLANE ( 'NONE',  #6147 ) ;
#27738=VECTOR ( 'NONE', #15706, 1000.000000000000000 ) ;
#27739=LINE ( 'NONE', #8474, #29701 ) ;
#27740=PLANE ( 'NONE',  #14804 ) ;
#27741=CARTESIAN_POINT ( 'NONE',  ( 172.7287565553229456, -9.999999999999980460, -41.50000000000000711 ) ) ;
#27749=CARTESIAN_POINT ( 'NONE',  ( 138.6922820468854525, -10.00000000000000533, -32.39392330124607611 ) ) ;
#27752=ORIENTED_EDGE ( 'NONE', *, *, #18176, .F. ) ;
#27753=CARTESIAN_POINT ( 'NONE',  ( 25.62901471571457890, -5.000000000000010658, -78.87799666457712533 ) ) ;
#27755=ORIENTED_EDGE ( 'NONE', *, *, #819, .F. ) ;
#27756=DIRECTION ( 'NONE',  ( -0.9510565162951536422, -2.566386769018988816E-16, -0.3090169943749472292 ) ) ;
#27757=LINE ( 'NONE', #15957, #24433 ) ;
#27758=DIRECTION ( 'NONE',  ( -0.8090169943749474513, -2.183098979609982436E-16, -0.5877852522924731371 ) ) ;
#27762=VECTOR ( 'NONE', #17151, 1000.000000000000000 ) ;
#27764=EDGE_CURVE ( 'NONE', #13474, #1407, #679, .T. ) ;
#27766=EDGE_CURVE ( 'NONE', #18100, #19125, #24037, .T. ) ;
#27769=CARTESIAN_POINT ( 'NONE',  ( 114.8169341242263215, -4.999999999999985789, -83.41938557644036223 ) ) ;
#27770=ADVANCED_FACE ( 'NONE', ( #7404 ), #14545, .T. ) ;
#27773=FACE_OUTER_BOUND ( 'NONE', #6395, .T. ) ;
#27775=ORIENTED_EDGE ( 'NONE', *, *, #22974, .F. ) ;
#27776=ORIENTED_EDGE ( 'NONE', *, *, #9472, .F. ) ;
#27777=DIRECTION ( 'NONE',  ( -2.698458740408365879E-16, 1.000000000000000000, 0.000000000000000000 ) ) ;
#27780=VECTOR ( 'NONE', #990, 1000.000000000000000 ) ;
#27784=FACE_OUTER_BOUND ( 'NONE', #6398, .T. ) ;
#27787=DIRECTION ( 'NONE',  ( -2.698458740408365879E-16, 1.000000000000000000, 0.000000000000000000 ) ) ;
#27788=VECTOR ( 'NONE', #14425, 1000.000000000000000 ) ;
#27789=CARTESIAN_POINT ( 'NONE',  ( 129.5152310637605524, -10.00000000000000888, -4.391296821672111328 ) ) ;
#27790=EDGE_LOOP ( 'NONE', ( #28934, #22783, #2520, #24689, #2127, #10116 ) ) ;
#27792=DIRECTION ( 'NONE',  ( 1.110223024625156540E-16, 2.995891024602366092E-32, 1.000000000000000000 ) ) ;
#27794=EDGE_LOOP ( 'NONE', ( #9149, #25443, #5229, #24277 ) ) ;
#27795=DIRECTION ( 'NONE',  ( -2.698458740408365879E-16, 1.000000000000000000, 0.000000000000000000 ) ) ;
#27796=ORIENTED_EDGE ( 'NONE', *, *, #5158, .T. ) ;
#27801=CARTESIAN_POINT ( 'NONE',  ( 138.6922820468854241, -10.00000000000000533, -0.6060766987539614181 ) ) ;
#27802=CARTESIAN_POINT ( 'NONE',  ( 133.6922820468854241, -1.999999999999981348, -9.266330736598357376 ) ) ;
#27804=CARTESIAN_POINT ( 'NONE',  ( 8.930358392086997554, -5.000000000000015099, 27.48481700440100184 ) ) ;
#27805=ADVANCED_FACE ( 'NONE', ( #3573 ), #24782, .T. ) ;
#27809=SURFACE_SIDE_STYLE ('',( #13863 ) ) ;
#27810=LINE ( 'NONE', #13722, #8406 ) ;
#27811=LINE ( 'NONE', #8279, #21881 ) ;
#27812=DIRECTION ( 'NONE',  ( -2.698458740408365879E-16, 1.000000000000000000, 0.000000000000000000 ) ) ;
#27813=DIRECTION ( 'NONE',  ( 0.5877852522924731371, 1.586114251531760728E-16, -0.8090169943749474513 ) ) ;
#27816=PLANE ( 'NONE',  #28291 ) ;
#27817=ORIENTED_EDGE ( 'NONE', *, *, #14652, .F. ) ;
#27819=LINE ( 'NONE', #9139, #23170 ) ;
#27824=EDGE_CURVE ( 'NONE', #18145, #10339, #12864, .T. ) ;
#27826=ORIENTED_EDGE ( 'NONE', *, *, #13137, .F. ) ;
#27828=VECTOR ( 'NONE', #14239, 999.9999999999998863 ) ;
#27830=FACE_OUTER_BOUND ( 'NONE', #19457, .T. ) ;
#27831=CARTESIAN_POINT ( 'NONE',  ( 147.0152310637605524, -10.00000000000000178, -17.38167787843871182 ) ) ;
#27832=ORIENTED_EDGE ( 'NONE', *, *, #24740, .F. ) ;
#27833=VECTOR ( 'NONE', #7730, 1000.000000000000000 ) ;
#27835=FACE_OUTER_BOUND ( 'NONE', #113, .T. ) ;
#27836=ORIENTED_EDGE ( 'NONE', *, *, #9629, .F. ) ;
#27838=ORIENTED_EDGE ( 'NONE', *, *, #14059, .T. ) ;
#27843=EDGE_LOOP ( 'NONE', ( #14820, #18924, #1261, #5890, #24233 ) ) ;
#27844=DIRECTION ( 'NONE',  ( 0.5877852522924731371, 1.586114251531760728E-16, -0.8090169943749474513 ) ) ;
#27847=VECTOR ( 'NONE', #2652, 1000.000000000000000 ) ;
#27849=ORIENTED_EDGE ( 'NONE', *, *, #1667, .T. ) ;
#27850=CARTESIAN_POINT ( 'NONE',  ( 129.5152310637605808, -1.999999999999982236, -11.28819510263909187 ) ) ;
#27852=LINE ( 'NONE', #6913, #23797 ) ;
#27853=CARTESIAN_POINT ( 'NONE',  ( 153.6922820468854241, -4.999999999999976907, -26.58683881228715862 ) ) ;
#27854=CARTESIAN_POINT ( 'NONE',  ( 157.0152310637605524, -9.999999999999998224, -34.70218595412750773 ) ) ;
#27858=AXIS2_PLACEMENT_3D ( 'NONE', #21785, #3778, #5920 ) ;
#27859=ADVANCED_FACE ( 'NONE', ( #13019 ), #20041, .T. ) ;
#27860=EDGE_CURVE ( 'NONE', #16811, #1407, #17736, .T. ) ;
#27861=ORIENTED_EDGE ( 'NONE', *, *, #3570, .T. ) ;
#27862=CARTESIAN_POINT ( 'NONE',  ( 156.1922820468853956, -4.999999999999975131, -19.40354224447947828 ) ) ;
#27864=VECTOR ( 'NONE', #7745, 1000.000000000000000 ) ;
#27867=ADVANCED_FACE ( 'NONE', ( #13168 ), #19728, .T. ) ;
#27869=CARTESIAN_POINT ( 'NONE',  ( 14.89669440878228635, -5.000000000000013323, 45.84731114023986720 ) ) ;
#27870=LINE ( 'NONE', #22651, #11148 ) ;
#27871=EDGE_CURVE ( 'NONE', #6983, #27422, #1286, .T. ) ;
#27873=VERTEX_POINT ( 'NONE', #27097 ) ;
#27874=ORIENTED_EDGE ( 'NONE', *, *, #17587, .F. ) ;
#27879=PLANE ( 'NONE',  #10594 ) ;
#27881=ORIENTED_EDGE ( 'NONE', *, *, #15125, .T. ) ;
#27882=PLANE ( 'NONE',  #13483 ) ;
#27886=VERTEX_POINT ( 'NONE', #29247 ) ;
#27887=VECTOR ( 'NONE', #14734, 1000.000000000000000 ) ;
#27888=CARTESIAN_POINT ( 'NONE',  ( 151.1922820468853956, -10.00000000000000178, -13.59645775552055902 ) ) ;
#27890=LINE ( 'NONE', #11805, #12837 ) ;
#27892=LINE ( 'NONE', #13795, #3658 ) ;
#27896=EDGE_CURVE ( 'NONE', #3964, #7930, #1593, .T. ) ;
#27899=LINE ( 'NONE', #16558, #8218 ) ;
#27901=ADVANCED_FACE ( 'NONE', ( #27258 ), #26949, .T. ) ;
#27903=DIRECTION ( 'NONE',  ( -0.8090169943749474513, -2.183098979609982436E-16, -0.5877852522924731371 ) ) ;
#27904=ADVANCED_FACE ( 'NONE', ( #6006 ), #15293, .T. ) ;
#27907=LINE ( 'NONE', #22995, #8085 ) ;
#27910=FACE_OUTER_BOUND ( 'NONE', #27988, .T. ) ;
#27911=CARTESIAN_POINT ( 'NONE',  ( 166.1922820468853672, -1.999999999999972244, -28.06379628232387446 ) ) ;
#27913=EDGE_LOOP ( 'NONE', ( #868, #5535, #16067, #22986 ) ) ;
#27914=ORIENTED_EDGE ( 'NONE', *, *, #11210, .T. ) ;
#27919=VECTOR ( 'NONE', #16005, 1000.000000000000000 ) ;
#27920=VERTEX_POINT ( 'NONE', #24178 ) ;
#27922=CARTESIAN_POINT ( 'NONE',  ( 147.0152310637604955, -10.00000000000000355, -0.06116980274991495881 ) ) ;
#27923=ORIENTED_EDGE ( 'NONE', *, *, #15202, .T. ) ;
#27924=ORIENTED_EDGE ( 'NONE', *, *, #1203, .F. ) ;
#27925=LINE ( 'NONE', #18268, #22142 ) ;
#27926=LINE ( 'NONE', #27625, #11678 ) ;
#27930=EDGE_CURVE ( 'NONE', #23167, #21077, #12559, .T. ) ;
#27931=VECTOR ( 'NONE', #5211, 1000.000000000000000 ) ;
#27933=LINE ( 'NONE', #9708, #17076 ) ;
#27934=DIRECTION ( 'NONE',  ( 1.110223024625156540E-16, 2.995891024602366092E-32, 1.000000000000000000 ) ) ;
#27935=EDGE_CURVE ( 'NONE', #24083, #7486, #14994, .T. ) ;
#27937=DIRECTION ( 'NONE',  ( -2.908569913943826047E-16, 1.000000000000000000, 6.826925868028084813E-18 ) ) ;
#27939=DIRECTION ( 'NONE',  ( 0.3090169943749472292, 8.338696094057992503E-17, -0.9510565162951536422 ) ) ;
#27940=EDGE_LOOP ( 'NONE', ( #12658, #6589, #15802, #25472, #4757 ) ) ;
#27941=CARTESIAN_POINT ( 'NONE',  ( 142.0152310637605240, -1.999999999999978684, -0.06116980274991495881 ) ) ;
#27943=VECTOR ( 'NONE', #9237, 1000.000000000000000 ) ;
#27944=ORIENTED_EDGE ( 'NONE', *, *, #19721, .F. ) ;
#27945=ORIENTED_EDGE ( 'NONE', *, *, #62, .T. ) ;
#27946=CARTESIAN_POINT ( 'NONE',  ( 100.5683542740252960, -4.999999999999990230, -73.06718635158908626 ) ) ;
#27947=ORIENTED_EDGE ( 'NONE', *, *, #27487, .F. ) ;
#27952=LINE ( 'NONE', #7009, #20866 ) ;
#27953=LINE ( 'NONE', #27802, #912 ) ;
#27956=ORIENTED_EDGE ( 'NONE', *, *, #23952, .T. ) ;
#27958=CARTESIAN_POINT ( 'NONE',  ( 162.0152310637605240, -9.999999999999998224, -34.70218595412750773 ) ) ;
#27959=CARTESIAN_POINT ( 'NONE',  ( 152.0152310637606092, -10.00000000000000000, -32.93883019725009120 ) ) ;
#27960=CARTESIAN_POINT ( 'NONE',  ( 169.7287565553229456, -9.999999999999996447, -25.16025403784440329 ) ) ;
#27963=DIRECTION ( 'NONE',  ( -0.9510565162951536422, -2.566386769018988323E-16, 0.3090169943749475623 ) ) ;
#27964=ORIENTED_EDGE ( 'NONE', *, *, #11286, .T. ) ;
#27966=VERTEX_POINT ( 'NONE', #8727 ) ;
#27967=EDGE_CURVE ( 'NONE', #2772, #20312, #29871, .T. ) ;
#27973=EDGE_CURVE ( 'NONE', #12642, #26976, #13905, .T. ) ;
#27974=ORIENTED_EDGE ( 'NONE', *, *, #10654, .F. ) ;
#27977=CARTESIAN_POINT ( 'NONE',  ( 166.1922820468853672, -9.999999999999998224, -22.25671179336496053 ) ) ;
#27979=CARTESIAN_POINT ( 'NONE',  ( 154.5152310637605524, -10.00000000000000000, -19.94844914048349693 ) ) ;
#27980=CARTESIAN_POINT ( 'NONE',  ( 132.0152310637605524, -10.00000000000000711, -17.38167787843870826 ) ) ;
#27981=ORIENTED_EDGE ( 'NONE', *, *, #14357, .T. ) ;
#27983=ORIENTED_EDGE ( 'NONE', *, *, #28618, .T. ) ;
#27985=ORIENTED_EDGE ( 'NONE', *, *, #28212, .F. ) ;
#27988=EDGE_LOOP ( 'NONE', ( #16468, #14265, #29528, #23683 ) ) ;
#27989=DIRECTION ( 'NONE',  ( -0.8090169943749474513, -2.183098979609982436E-16, 0.5877852522924731371 ) ) ;
#27990=VECTOR ( 'NONE', #1137, 1000.000000000000000 ) ;
#27997=AXIS2_PLACEMENT_3D ( 'NONE', #19845, #793, #17117 ) ;
#27998=PLANE ( 'NONE',  #22552 ) ;
#28001=LINE ( 'NONE', #27854, #16803 ) ;
#28003=EDGE_CURVE ( 'NONE', #29073, #14905, #8879, .T. ) ;
#28005=PLANE ( 'NONE',  #28309 ) ;
#28006=VERTEX_POINT ( 'NONE', #18498 ) ;
#28008=VERTEX_POINT ( 'NONE', #27853 ) ;
#28010=ORIENTED_EDGE ( 'NONE', *, *, #22321, .F. ) ;
#28012=DIRECTION ( 'NONE',  ( -0.9510565162951536422, -2.566386769018988323E-16, 0.3090169943749475623 ) ) ;
#28015=VERTEX_POINT ( 'NONE', #22638 ) ;
#28020=ORIENTED_EDGE ( 'NONE', *, *, #6987, .T. ) ;
#28021=ORIENTED_EDGE ( 'NONE', *, *, #5294, .T. ) ;
#28022=EDGE_LOOP ( 'NONE', ( #9346, #21154, #16807, #20477 ) ) ;
#28023=FACE_OUTER_BOUND ( 'NONE', #15840, .T. ) ;
#28025=EDGE_LOOP ( 'NONE', ( #27539, #142, #24397, #2105 ) ) ;
#28026=CARTESIAN_POINT ( 'NONE',  ( 131.1922820468854241, -10.00000000000000888, -13.59645775552055547 ) ) ;
#28027=ORIENTED_EDGE ( 'NONE', *, *, #8988, .F. ) ;
#28032=ADVANCED_FACE ( 'NONE', ( #6914 ), #20483, .T. ) ;
#28033=DIRECTION ( 'NONE',  ( 0.9510565162951535312, 2.566386769018988816E-16, -0.3090169943749475623 ) ) ;
#28034=EDGE_CURVE ( 'NONE', #24158, #4384, #16207, .T. ) ;
#28035=VECTOR ( 'NONE', #7660, 1000.000000000000000 ) ;
#28037=DIRECTION ( 'NONE',  ( -2.698458740408365879E-16, 1.000000000000000000, 0.000000000000000000 ) ) ;
#28039=PLANE ( 'NONE',  #25549 ) ;
#28044=ORIENTED_EDGE ( 'NONE', *, *, #11471, .T. ) ;
#28047=VECTOR ( 'NONE', #15455, 1000.000000000000000 ) ;
#28048=DIRECTION ( 'NONE',  ( -0.5877852522924731371, -1.586114251531760728E-16, -0.8090169943749474513 ) ) ;
#28049=CARTESIAN_POINT ( 'NONE',  ( 176.1922820468852535, -9.999999999999994671, -4.936203717676158398 ) ) ;
#28050=CARTESIAN_POINT ( 'NONE',  ( 146.1922820468854241, -10.00000000000000355, -13.59645775552055902 ) ) ;
#28051=ORIENTED_EDGE ( 'NONE', *, *, #21958, .T. ) ;
#28055=LINE ( 'NONE', #25734, #22740 ) ;
#28056=LINE ( 'NONE', #7110, #11259 ) ;
#28057=ORIENTED_EDGE ( 'NONE', *, *, #25415, .T. ) ;
#28060=VERTEX_POINT ( 'NONE', #20932 ) ;
#28062=ORIENTED_EDGE ( 'NONE', *, *, #16484, .T. ) ;
#28067=EDGE_CURVE ( 'NONE', #23858, #14791, #2192, .T. ) ;
#28068=EDGE_CURVE ( 'NONE', #26594, #13044, #25523, .T. ) ;
#28069=VECTOR ( 'NONE', #25344, 999.9999999999998863 ) ;
#28070=ORIENTED_EDGE ( 'NONE', *, *, #2270, .T. ) ;
#28071=EDGE_CURVE ( 'NONE', #25350, #26426, #20630, .T. ) ;
#28072=CARTESIAN_POINT ( 'NONE',  ( 142.0152310637605524, -10.00000000000000355, -8.721423840594312082 ) ) ;
#28073=FACE_OUTER_BOUND ( 'NONE', #22521, .T. ) ;
#28074=VERTEX_POINT ( 'NONE', #2345 ) ;
#28075=LINE ( 'NONE', #9099, #7536 ) ;
#28076=DIRECTION ( 'NONE',  ( 0.9510565162951535312, 2.566386769018988816E-16, -0.3090169943749475623 ) ) ;
#28080=DIRECTION ( 'NONE',  ( 0.5877852522924731371, 1.586114251531760728E-16, 0.8090169943749474513 ) ) ;
#28081=FACE_OUTER_BOUND ( 'NONE', #21487, .T. ) ;
#28083=DIRECTION ( 'NONE',  ( 1.000000000000000000, 2.891205793294675861E-16, 0.000000000000000000 ) ) ;
#28084=DIRECTION ( 'NONE',  ( -1.110223024625156540E-16, 0.000000000000000000, -1.000000000000000000 ) ) ;
#28086=DIRECTION ( 'NONE',  ( 0.5877852522924731371, 0.000000000000000000, 0.8090169943749474513 ) ) ;
#28088=LINE ( 'NONE', #9417, #13492 ) ;
#28091=ADVANCED_FACE ( 'NONE', ( #11620 ), #15747, .T. ) ;
#28095=LINE ( 'NONE', #27801, #23812 ) ;
#28097=FACE_OUTER_BOUND ( 'NONE', #12457, .T. ) ;
#28098=VECTOR ( 'NONE', #4995, 1000.000000000000000 ) ;
#28101=AXIS2_PLACEMENT_3D ( 'NONE', #20095, #22232, #15663 ) ;
#28102=EDGE_CURVE ( 'NONE', #28590, #28404, #1738, .T. ) ;
#28103=ADVANCED_FACE ( 'NONE', ( #15898 ), #25229, .T. ) ;
#28105=ORIENTED_EDGE ( 'NONE', *, *, #19745, .T. ) ;
#28106=EDGE_CURVE ( 'NONE', #9002, #13085, #2044, .T. ) ;
#28107=DIRECTION ( 'NONE',  ( -0.9510565162951536422, 0.000000000000000000, -0.3090169943749472292 ) ) ;
#28108=LINE ( 'NONE', #14164, #23342 ) ;
#28109=VECTOR ( 'NONE', #12281, 1000.000000000000000 ) ;
#28117=ORIENTED_EDGE ( 'NONE', *, *, #16348, .T. ) ;
#28119=VERTEX_POINT ( 'NONE', #6757 ) ;
#28120=CARTESIAN_POINT ( 'NONE',  ( 167.0152310637604955, -4.999999999999972466, -26.04193191628311155 ) ) ;
#28123=DIRECTION ( 'NONE',  ( 0.9510565162951536422, 2.566386769018988816E-16, 0.3090169943749472292 ) ) ;
#28125=VERTEX_POINT ( 'NONE', #25375 ) ;
#28127=PLANE ( 'NONE',  #6243 ) ;
#28128=VECTOR ( 'NONE', #4969, 1000.000000000000000 ) ;
#28130=CARTESIAN_POINT ( 'NONE',  ( 152.2287565553229740, -4.999999999999976907, -12.16987298107781434 ) ) ;
#28131=DIRECTION ( 'NONE',  ( -1.110223024625156540E-16, 0.000000000000000000, -1.000000000000000000 ) ) ;
#28132=ORIENTED_EDGE ( 'NONE', *, *, #14575, .T. ) ;
#28134=ORIENTED_EDGE ( 'NONE', *, *, #16759, .T. ) ;
#28142=AXIS2_PLACEMENT_3D ( 'NONE', #27707, #11034, #10740 ) ;
#28143=CARTESIAN_POINT ( 'NONE',  ( 136.1922820468854241, -10.00000000000000533, -22.25671179336495697 ) ) ;
#28146=EDGE_LOOP ( 'NONE', ( #26022, #12089, #13808, #22889 ) ) ;
#28149=EDGE_CURVE ( 'NONE', #26420, #15422, #4469, .T. ) ;
#28150=EDGE_CURVE ( 'NONE', #22770, #23142, #7061, .T. ) ;
#28151=EDGE_CURVE ( 'NONE', #14407, #17627, #21088, .T. ) ;
#28152=ORIENTED_EDGE ( 'NONE', *, *, #23879, .T. ) ;
#28153=FACE_OUTER_BOUND ( 'NONE', #3519, .T. ) ;
#28155=PLANE ( 'NONE',  #19877 ) ;
#28156=CARTESIAN_POINT ( 'NONE',  ( 21.57250875526980849, -5.000000000000011546, -66.39335505166295093 ) ) ;
#28157=AXIS2_PLACEMENT_3D ( 'NONE', #1382, #29353, #8378 ) ;
#28162=CARTESIAN_POINT ( 'NONE',  ( 129.5152310637605808, -1.999999999999982236, -11.28819510263909187 ) ) ;
#28164=DIRECTION ( 'NONE',  ( -0.9510565162951536422, -2.566386769018988816E-16, -0.3090169943749472292 ) ) ;
#28165=ORIENTED_EDGE ( 'NONE', *, *, #20027, .T. ) ;
#28168=CARTESIAN_POINT ( 'NONE',  ( 142.0152310637606092, -1.999999999999978018, -15.61832212156129707 ) ) ;
#28169=PLANE ( 'NONE',  #6199 ) ;
#28172=FACE_OUTER_BOUND ( 'NONE', #3309, .T. ) ;
#28174=ORIENTED_EDGE ( 'NONE', *, *, #10346, .T. ) ;
#28176=FACE_OUTER_BOUND ( 'NONE', #19700, .T. ) ;
#28178=DIRECTION ( 'NONE',  ( -0.8090169943749474513, -2.183098979609982436E-16, -0.5877852522924731371 ) ) ;
#28180=ORIENTED_EDGE ( 'NONE', *, *, #26866, .F. ) ;
#28181=CARTESIAN_POINT ( 'NONE',  ( 143.6922820468854525, -1.999999999999978018, -17.92658477444275889 ) ) ;
#28182=VERTEX_POINT ( 'NONE', #16664 ) ;
#28185=VECTOR ( 'NONE', #13782, 1000.000000000000000 ) ;
#28187=ADVANCED_FACE ( 'NONE', ( #9931 ), #26137, .T. ) ;
#28188=ORIENTED_EDGE ( 'NONE', *, *, #27653, .F. ) ;
#28189=EDGE_CURVE ( 'NONE', #22328, #2206, #11771, .T. ) ;
#28190=ORIENTED_EDGE ( 'NONE', *, *, #1757, .F. ) ;
#28191=DIRECTION ( 'NONE',  ( -2.698458740408365879E-16, 1.000000000000000000, 0.000000000000000000 ) ) ;
#28193=CARTESIAN_POINT ( 'NONE',  ( 172.2287565553228887, -9.999999999999996447, -12.16987298107780369 ) ) ;
#28194=PLANE ( 'NONE',  #20738 ) ;
#28197=VECTOR ( 'NONE', #17630, 1000.000000000000000 ) ;
#28202=VERTEX_POINT ( 'NONE', #7656 ) ;
#28203=LINE ( 'NONE', #9520, #7593 ) ;
#28206=LINE ( 'NONE', #14253, #9313 ) ;
#28207=CARTESIAN_POINT ( 'NONE',  ( 134.5152310637605524, -4.999999999999981348, -30.37205893520530964 ) ) ;
#28209=VERTEX_POINT ( 'NONE', #19244 ) ;
#28210=CARTESIAN_POINT ( 'NONE',  ( 173.6922820468852535, -1.999999999999970024, 2.247092850131519715 ) ) ;
#28212=EDGE_CURVE ( 'NONE', #102, #9595, #28599, .T. ) ;
#28216=DIRECTION ( 'NONE',  ( 0.9510565162951536422, 0.000000000000000000, -0.3090169943749475623 ) ) ;
#28221=EDGE_LOOP ( 'NONE', ( #1381, #2485, #24540, #14487 ) ) ;
#28225=AXIS2_PLACEMENT_3D ( 'NONE', #3098, #21685, #5213 ) ;
#28229=FACE_OUTER_BOUND ( 'NONE', #14738, .T. ) ;
#28231=CARTESIAN_POINT ( 'NONE',  ( 157.0152310637604671, -4.999999999999975131, -1.743219247438259813E-14 ) ) ;
#28236=CARTESIAN_POINT ( 'NONE',  ( 152.0152310637605240, -1.999999999999975797, -6.958068083716895558 ) ) ;
#28237=PLANE ( 'NONE',  #13888 ) ;
#28239=DIRECTION ( 'NONE',  ( 0.5877852522924731371, 1.586114251531760728E-16, -0.8090169943749474513 ) ) ;
#28243=ORIENTED_EDGE ( 'NONE', *, *, #3987, .F. ) ;
#28244=VECTOR ( 'NONE', #26480, 1000.000000000000000 ) ;
#28246=EDGE_CURVE ( 'NONE', #20619, #319, #5374, .T. ) ;
#28247=CARTESIAN_POINT ( 'NONE',  ( 154.5152310637604955, -10.00000000000000000, -13.05155085951651195 ) ) ;
#28248=ORIENTED_EDGE ( 'NONE', *, *, #24466, .T. ) ;
#28250=CARTESIAN_POINT ( 'NONE',  ( 133.6922820468854241, -1.999999999999980904, -15.07341522555727309 ) ) ;
#28251=ORIENTED_EDGE ( 'NONE', *, *, #8071, .T. ) ;
#28259=LINE ( 'NONE', #21187, #4225 ) ;
#28260=VERTEX_POINT ( 'NONE', #2502 ) ;
#28261=CARTESIAN_POINT ( 'NONE',  ( 132.2287565553230024, -10.00000000000000888, -29.49038105676660138 ) ) ;
#28263=DIRECTION ( 'NONE',  ( -0.5877852522924731371, -1.586114251531760728E-16, -0.8090169943749474513 ) ) ;
#28264=PLANE ( 'NONE',  #5856 ) ;
#28265=LINE ( 'NONE', #16772, #5064 ) ;
#28266=VECTOR ( 'NONE', #25483, 1000.000000000000000 ) ;
#28268=LINE ( 'NONE', #10042, #7726 ) ;
#28276=CARTESIAN_POINT ( 'NONE',  ( 125.7287565553229172, -9.999999999999994671, -33.50000000000000000 ) ) ;
#28278=EDGE_CURVE ( 'NONE', #30251, #23755, #349, .T. ) ;
#28282=EDGE_CURVE ( 'NONE', #9388, #24164, #2639, .T. ) ;
#28284=DIRECTION ( 'NONE',  ( -2.698458740408365879E-16, 1.000000000000000000, 0.000000000000000000 ) ) ;
#28285=EDGE_CURVE ( 'NONE', #16899, #7751, #18799, .T. ) ;
#28286=ORIENTED_EDGE ( 'NONE', *, *, #25976, .F. ) ;
#28287=LINE ( 'NONE', #8073, #2792 ) ;
#28288=ORIENTED_EDGE ( 'NONE', *, *, #10523, .T. ) ;
#28291=AXIS2_PLACEMENT_3D ( 'NONE', #25493, #4581, #20292 ) ;
#28295=DIRECTION ( 'NONE',  ( -0.8090169943749474513, -2.183098979609982436E-16, -0.5877852522924731371 ) ) ;
#28301=ORIENTED_EDGE ( 'NONE', *, *, #12111, .F. ) ;
#28302=FACE_BOUND ( 'NONE', #25512, .T. ) ;
#28304=CARTESIAN_POINT ( 'NONE',  ( 3.918937403516957740, -5.000000000000016875, 12.06124913002446597 ) ) ;
#28305=CARTESIAN_POINT ( 'NONE',  ( 171.1922820468853388, -1.999999999999970468, -22.25671179336496053 ) ) ;
#28306=VECTOR ( 'NONE', #14311, 1000.000000000000000 ) ;
#28307=DIRECTION ( 'NONE',  ( 1.110223024625156540E-16, 2.995891024602366092E-32, 1.000000000000000000 ) ) ;
#28308=CARTESIAN_POINT ( 'NONE',  ( 152.0152310637606092, -1.999999999999974465, -32.93883019725009120 ) ) ;
#28309=AXIS2_PLACEMENT_3D ( 'NONE', #23854, #11921, #504 ) ;
#28310=VECTOR ( 'NONE', #23156, 1000.000000000000000 ) ;
#28312=FACE_OUTER_BOUND ( 'NONE', #12715, .T. ) ;
#28313=LINE ( 'NONE', #21400, #12505 ) ;
#28314=EDGE_LOOP ( 'NONE', ( #13687, #13929, #18514, #27120 ) ) ;
#28316=ORIENTED_EDGE ( 'NONE', *, *, #2382, .F. ) ;
#28317=EDGE_CURVE ( 'NONE', #20741, #22085, #16806, .T. ) ;
#28318=EDGE_CURVE ( 'NONE', #14857, #19188, #21394, .T. ) ;
#28321=CARTESIAN_POINT ( 'NONE',  ( 163.6922820468853956, -1.999999999999971800, -35.24709285013155835 ) ) ;
#28322=LINE ( 'NONE', #18668, #11066 ) ;
#28323=EDGE_CURVE ( 'NONE', #10099, #28570, #23850, .T. ) ;
#28325=ORIENTED_EDGE ( 'NONE', *, *, #18172, .F. ) ;
#28326=DIRECTION ( 'NONE',  ( 0.3090169943749475623, 8.338696094058001131E-17, 0.9510565162951536422 ) ) ;
#28327=EDGE_CURVE ( 'NONE', #12785, #25944, #9636, .T. ) ;
#28329=AXIS2_PLACEMENT_3D ( 'NONE', #1682, #13406, #22732 ) ;
#28330=VERTEX_POINT ( 'NONE', #2950 ) ;
#28331=VECTOR ( 'NONE', #26493, 1000.000000000000000 ) ;
#28333=VECTOR ( 'NONE', #1906, 1000.000000000000000 ) ;
#28335=DIRECTION ( 'NONE',  ( 1.000000000000000000, 2.698458740408367851E-16, 0.000000000000000000 ) ) ;
#28338=VERTEX_POINT ( 'NONE', #5062 ) ;
#28340=AXIS2_PLACEMENT_3D ( 'NONE', #81, #20113, #19963 ) ;
#28343=EDGE_LOOP ( 'NONE', ( #10109, #25782, #16971, #14771, #27494 ) ) ;
#28344=DIRECTION ( 'NONE',  ( -0.9510565162951536422, -2.566386769018988323E-16, 0.3090169943749475623 ) ) ;
#28345=VERTEX_POINT ( 'NONE', #12228 ) ;
#28347=DIRECTION ( 'NONE',  ( 0.5877852522924731371, 1.586114251531760728E-16, -0.8090169943749474513 ) ) ;
#28348=VECTOR ( 'NONE', #20860, 1000.000000000000000 ) ;
#28349=CARTESIAN_POINT ( 'NONE',  ( 133.7287565553229456, -9.999999999999980460, 0.5000000000000029976 ) ) ;
#28351=VECTOR ( 'NONE', #23359, 1000.000000000000000 ) ;
#28352=DIRECTION ( 'NONE',  ( 1.110223024625156540E-16, 2.995891024602366092E-32, 1.000000000000000000 ) ) ;
#28357=ORIENTED_EDGE ( 'NONE', *, *, #26225, .T. ) ;
#28359=DIRECTION ( 'NONE',  ( 0.9510565162951536422, 2.566386769018988816E-16, 0.3090169943749472292 ) ) ;
#28360=ADVANCED_FACE ( 'NONE', ( #12077 ), #14352, .T. ) ;
#28361=CARTESIAN_POINT ( 'NONE',  ( 151.1922820468853956, -1.999999999999975797, -10.74328820663507678 ) ) ;
#28362=LINE ( 'NONE', #2549, #21716 ) ;
#28364=FACE_OUTER_BOUND ( 'NONE', #20953, .T. ) ;
#28365=EDGE_CURVE ( 'NONE', #18308, #19412, #17258, .T. ) ;
#28368=CARTESIAN_POINT ( 'NONE',  ( 133.6922820468854241, -10.00000000000000711, 2.247092850131519715 ) ) ;
#28373=AXIS2_PLACEMENT_3D ( 'NONE', #12003, #4548, #13837 ) ;
#28375=AXIS2_PLACEMENT_3D ( 'NONE', #22395, #13522, #1798 ) ;
#28379=VERTEX_POINT ( 'NONE', #21997 ) ;
#28380=LINE ( 'NONE', #21913, #18183 ) ;
#28381=EDGE_CURVE ( 'NONE', #13222, #2910, #24290, .T. ) ;
#28382=DIRECTION ( 'NONE',  ( 0.3090169943749472292, 8.338696094057992503E-17, -0.9510565162951536422 ) ) ;
#28383=ORIENTED_EDGE ( 'NONE', *, *, #4022, .F. ) ;
#28384=DIRECTION ( 'NONE',  ( 0.3090169943749472292, 8.338696094057992503E-17, -0.9510565162951536422 ) ) ;
#28385=LINE ( 'NONE', #26065, #29303 ) ;
#28389=ORIENTED_EDGE ( 'NONE', *, *, #23802, .F. ) ;
#28390=DIRECTION ( 'NONE',  ( 1.000000000000000000, 2.698458740408365879E-16, 0.000000000000000000 ) ) ;
#28393=EDGE_CURVE ( 'NONE', #5343, #21323, #22456, .T. ) ;
#28394=LINE ( 'NONE', #7447, #2949 ) ;
#28396=ORIENTED_EDGE ( 'NONE', *, *, #11687, .F. ) ;
#28397=DIRECTION ( 'NONE',  ( 0.9510565162951536422, 0.000000000000000000, -0.3090169943749475623 ) ) ;
#28399=ORIENTED_EDGE ( 'NONE', *, *, #28034, .T. ) ;
#28400=CARTESIAN_POINT ( 'NONE',  ( 162.0152310637605524, -4.999999999999973355, -32.93883019725009120 ) ) ;
#28401=ORIENTED_EDGE ( 'NONE', *, *, #22840, .F. ) ;
#28404=VERTEX_POINT ( 'NONE', #29373 ) ;
#28406=DIRECTION ( 'NONE',  ( 0.9510565162951536422, 2.566386769018988816E-16, 0.3090169943749472292 ) ) ;
#28407=CARTESIAN_POINT ( 'NONE',  ( 132.0152310637605524, -4.999999999999982236, -1.465663491281971624E-14 ) ) ;
#28408=DIRECTION ( 'NONE',  ( 0.9510565162951536422, 2.566386769018988816E-16, 0.3090169943749472292 ) ) ;
#28409=DIRECTION ( 'NONE',  ( -0.5877852522924731371, -1.586114251531760235E-16, 0.8090169943749474513 ) ) ;
#28411=DIRECTION ( 'NONE',  ( -0.8090169943749474513, -2.183098979609982436E-16, 0.5877852522924731371 ) ) ;
#28412=DIRECTION ( 'NONE',  ( 1.000000000000000000, 2.891205793294675861E-16, 0.000000000000000000 ) ) ;
#28413=EDGE_CURVE ( 'NONE', #13701, #12555, #29055, .T. ) ;
#28415=DIRECTION ( 'NONE',  ( 0.5877852522924731371, 1.586114251531760728E-16, 0.8090169943749474513 ) ) ;
#28417=CARTESIAN_POINT ( 'NONE',  ( 176.1922820468853104, -9.999999999999994671, -22.25671179336496053 ) ) ;
#28419=ORIENTED_EDGE ( 'NONE', *, *, #15787, .T. ) ;
#28426=CARTESIAN_POINT ( 'NONE',  ( 19.18522118495666007, -5.000000000000012434, -59.04603939800706058 ) ) ;
#28427=ORIENTED_EDGE ( 'NONE', *, *, #7768, .T. ) ;
#28431=CARTESIAN_POINT ( 'NONE',  ( 176.1922820468853388, -9.999999999999994671, -30.91696583120936026 ) ) ;
#28432=ORIENTED_EDGE ( 'NONE', *, *, #2863, .F. ) ;
#28433=CARTESIAN_POINT ( 'NONE',  ( 130.7287565553229456, -4.999999999999982236, -30.76635726929466585 ) ) ;
#28434=EDGE_LOOP ( 'NONE', ( #27945, #17936, #17419, #7897 ) ) ;
#28440=VECTOR ( 'NONE', #29200, 1000.000000000000000 ) ;
#28442=DIRECTION ( 'NONE',  ( 0.9510565162951535312, 2.566386769018988816E-16, -0.3090169943749475623 ) ) ;
#28443=VERTEX_POINT ( 'NONE', #17558 ) ;
#28444=LINE ( 'NONE', #25664, #10817 ) ;
#28448=VECTOR ( 'NONE', #23796, 1000.000000000000000 ) ;
#28449=ORIENTED_EDGE ( 'NONE', *, *, #26052, .T. ) ;
#28450=FACE_BOUND ( 'NONE', #9150, .T. ) ;
#28451=EDGE_CURVE ( 'NONE', #15396, #7245, #1247, .T. ) ;
#28454=DIRECTION ( 'NONE',  ( 0.9510565162951535312, 2.566386769018988816E-16, -0.3090169943749475623 ) ) ;
#28455=CARTESIAN_POINT ( 'NONE',  ( 138.6922820468854525, -1.999999999999979572, -17.92658477444275533 ) ) ;
#28456=DIRECTION ( 'NONE',  ( -0.9510565162951536422, -2.566386769018988816E-16, -0.3090169943749472292 ) ) ;
#28457=VECTOR ( 'NONE', #28873, 1000.000000000000000 ) ;
#28460=LINE ( 'NONE', #9480, #24102 ) ;
#28461=ORIENTED_EDGE ( 'NONE', *, *, #19814, .T. ) ;
#28465=VERTEX_POINT ( 'NONE', #3534 ) ;
#28466=AXIS2_PLACEMENT_3D ( 'NONE', #12297, #21612, #21464 ) ;
#28468=CARTESIAN_POINT ( 'NONE',  ( 149.5152310637605808, -1.999999999999975353, -30.37205893520531319 ) ) ;
#28469=CARTESIAN_POINT ( 'NONE',  ( 79.48924668973215546, -4.999999999999995559, 57.75231823919976648 ) ) ;
#28470=FACE_OUTER_BOUND ( 'NONE', #19107, .T. ) ;
#28471=ORIENTED_EDGE ( 'NONE', *, *, #8623, .T. ) ;
#28474=ORIENTED_EDGE ( 'NONE', *, *, #7665, .T. ) ;
#28477=ORIENTED_EDGE ( 'NONE', *, *, #18902, .F. ) ;
#28478=VERTEX_POINT ( 'NONE', #6117 ) ;
#28479=DIRECTION ( 'NONE',  ( 0.5877852522924731371, 1.586114251531760728E-16, 0.8090169943749474513 ) ) ;
#28482=ORIENTED_EDGE ( 'NONE', *, *, #3371, .F. ) ;
#28483=CARTESIAN_POINT ( 'NONE',  ( 168.6922820468853104, -1.999999999999971800, -9.266330736598359152 ) ) ;
#28486=ORIENTED_EDGE ( 'NONE', *, *, #16936, .F. ) ;
#28487=LINE ( 'NONE', #2259, #3557 ) ;
#28488=ORIENTED_EDGE ( 'NONE', *, *, #9998, .F. ) ;
#28490=LINE ( 'NONE', #28634, #27828 ) ;
#28491=EDGE_CURVE ( 'NONE', #10208, #19917, #28763, .T. ) ;
#28492=AXIS2_PLACEMENT_3D ( 'NONE', #10909, #17772, #10455 ) ;
#28494=ADVANCED_FACE ( 'NONE', ( #26441 ), #15260, .T. ) ;
#28495=DIRECTION ( 'NONE',  ( -1.110223024625156540E-16, 0.000000000000000000, -1.000000000000000000 ) ) ;
#28496=ADVANCED_FACE ( 'NONE', ( #3245 ), #24838, .T. ) ;
#28497=DIRECTION ( 'NONE',  ( -0.5877852522924731371, -1.586114251531760728E-16, -0.8090169943749474513 ) ) ;
#28498=CARTESIAN_POINT ( 'NONE',  ( 173.6922820468853104, -9.999999999999994671, -15.07341522555727664 ) ) ;
#28499=DIRECTION ( 'NONE',  ( 0.5877852522924731371, 1.586114251531760728E-16, 0.8090169943749474513 ) ) ;
#28505=CARTESIAN_POINT ( 'NONE',  ( 180.7287565553229740, -84.33034373659253902, 0.5000000000000029976 ) ) ;
#28507=LINE ( 'NONE', #12423, #14189 ) ;
#28508=LINE ( 'NONE', #11966, #14126 ) ;
#28510=ORIENTED_EDGE ( 'NONE', *, *, #24561, .F. ) ;
#28511=CARTESIAN_POINT ( 'NONE',  ( 133.6922820468854241, -1.999999999999981348, -26.58683881228715506 ) ) ;
#28513=CARTESIAN_POINT ( 'NONE',  ( 169.7287565553228887, -9.999999999999998224, -7.839745962155603820 ) ) ;
#28516=VECTOR ( 'NONE', #903, 999.9999999999998863 ) ;
#28518=EDGE_LOOP ( 'NONE', ( #3842, #20515, #920, #23237 ) ) ;
#28522=VERTEX_POINT ( 'NONE', #7807 ) ;
#28527=DIRECTION ( 'NONE',  ( -0.8090169943749474513, -2.183098979609982436E-16, -0.5877852522924731371 ) ) ;
#28528=ADVANCED_FACE ( 'NONE', ( #10234 ), #10692, .T. ) ;
#28529=CARTESIAN_POINT ( 'NONE',  ( 131.1922820468854241, -10.00000000000000888, -4.936203717676158398 ) ) ;
#28530=FACE_OUTER_BOUND ( 'NONE', #12968, .T. ) ;
#28531=AXIS2_PLACEMENT_3D ( 'NONE', #25752, #4681, #23306 ) ;
#28535=DIRECTION ( 'NONE',  ( -2.698458740408365879E-16, 1.000000000000000000, 0.000000000000000000 ) ) ;
#28536=CARTESIAN_POINT ( 'NONE',  ( 98.70167508945917234, -4.999999999999990230, 71.71096453785942515 ) ) ;
#28540=VERTEX_POINT ( 'NONE', #25048 ) ;
#28541=DIRECTION ( 'NONE',  ( -2.698458740408365879E-16, 1.000000000000000000, 0.000000000000000000 ) ) ;
#28543=ORIENTED_EDGE ( 'NONE', *, *, #14988, .F. ) ;
#28544=ORIENTED_EDGE ( 'NONE', *, *, #22070, .F. ) ;
#28549=CARTESIAN_POINT ( 'NONE',  ( 162.2287565553229456, -9.999999999999998224, -20.83012701892220520 ) ) ;
#28550=LINE ( 'NONE', #17064, #14047 ) ;
#28552=LINE ( 'NONE', #11722, #598 ) ;
#28554=LINE ( 'NONE', #12179, #28951 ) ;
#28555=FACE_OUTER_BOUND ( 'NONE', #21011, .T. ) ;
#28556=PLANE ( 'NONE',  #16013 ) ;
#28557=ADVANCED_FACE ( 'NONE', ( #18006 ), #20595, .T. ) ;
#28558=PLANE ( 'NONE',  #6864 ) ;
#28559=LINE ( 'NONE', #24101, #29989 ) ;
#28561=CARTESIAN_POINT ( 'NONE',  ( 164.7287565553228887, -1.999999999999972244, -7.839745962155603820 ) ) ;
#28562=PLANE ( 'NONE',  #10699 ) ;
#28563=ORIENTED_EDGE ( 'NONE', *, *, #2108, .F. ) ;
#28565=FACE_OUTER_BOUND ( 'NONE', #17740, .T. ) ;
#28569=CARTESIAN_POINT ( 'NONE',  ( 148.6922820468854525, -1.999999999999975797, -23.73366926340167637 ) ) ;
#28570=VERTEX_POINT ( 'NONE', #6883 ) ;
#28571=ORIENTED_EDGE ( 'NONE', *, *, #25754, .T. ) ;
#28577=CARTESIAN_POINT ( 'NONE',  ( 136.1922820468854241, -4.999999999999981348, -30.91696583120935671 ) ) ;
#28578=ORIENTED_EDGE ( 'NONE', *, *, #13651, .T. ) ;
#28580=EDGE_CURVE ( 'NONE', #24253, #16928, #4133, .T. ) ;
#28581=ORIENTED_EDGE ( 'NONE', *, *, #861, .T. ) ;
#28585=ADVANCED_FACE ( 'NONE', ( #16016 ), #13426, .T. ) ;
#28586=ORIENTED_EDGE ( 'NONE', *, *, #4234, .T. ) ;
#28587=VECTOR ( 'NONE', #22118, 1000.000000000000000 ) ;
#28588=CARTESIAN_POINT ( 'NONE',  ( 139.7287565553230024, -10.00000000000000533, 0.8205080756887930260 ) ) ;
#28589=ORIENTED_EDGE ( 'NONE', *, *, #7941, .T. ) ;
#28590=VERTEX_POINT ( 'NONE', #24900 ) ;
#28591=CARTESIAN_POINT ( 'NONE',  ( 142.2287565553230309, -10.00000000000000533, -20.83012701892220164 ) ) ;
#28593=VECTOR ( 'NONE', #8032, 1000.000000000000000 ) ;
#28596=CARTESIAN_POINT ( 'NONE',  ( 156.1922820468854241, -1.999999999999974021, -30.91696583120936026 ) ) ;
#28597=CARTESIAN_POINT ( 'NONE',  ( 164.5152310637604671, -1.999999999999972244, -13.05155085951651195 ) ) ;
#28598=DIRECTION ( 'NONE',  ( -2.698458740408365879E-16, 1.000000000000000000, 0.000000000000000000 ) ) ;
#28599=LINE ( 'NONE', #21235, #9693 ) ;
#28600=DIRECTION ( 'NONE',  ( 0.5877852522924731371, 0.000000000000000000, 0.8090169943749474513 ) ) ;
#28601=VECTOR ( 'NONE', #17022, 1000.000000000000000 ) ;
#28604=CARTESIAN_POINT ( 'NONE',  ( 84.03026872336096176, -4.999999999999994671, 61.05156386724048190 ) ) ;
#28605=ORIENTED_EDGE ( 'NONE', *, *, #4697, .F. ) ;
#28606=VECTOR ( 'NONE', #7858, 1000.000000000000000 ) ;
#28608=ORIENTED_EDGE ( 'NONE', *, *, #6640, .T. ) ;
#28610=FACE_OUTER_BOUND ( 'NONE', #25819, .T. ) ;
#28612=LINE ( 'NONE', #2456, #28306 ) ;
#28613=EDGE_LOOP ( 'NONE', ( #222, #22853, #1980, #27521 ) ) ;
#28616=EDGE_CURVE ( 'NONE', #15678, #8129, #6274, .T. ) ;
#28617=ORIENTED_EDGE ( 'NONE', *, *, #14577, .F. ) ;
#28618=EDGE_CURVE ( 'NONE', #11106, #11337, #22603, .T. ) ;
#28621=EDGE_CURVE ( 'NONE', #2945, #23086, #6724, .T. ) ;
#28622=DIRECTION ( 'NONE',  ( 1.110223024625156540E-16, 2.995891024602366092E-32, 1.000000000000000000 ) ) ;
#28631=DIRECTION ( 'NONE',  ( -0.8090169943749474513, -2.183098979609982436E-16, -0.5877852522924731371 ) ) ;
#28632=ORIENTED_EDGE ( 'NONE', *, *, #8980, .T. ) ;
#28633=ORIENTED_EDGE ( 'NONE', *, *, #4499, .F. ) ;
#28634=CARTESIAN_POINT ( 'NONE',  ( 5.351309945704854520, -5.000000000000015987, 16.46963852221801972 ) ) ;
#28635=AXIS2_PLACEMENT_3D ( 'NONE', #11931, #4931, #11786 ) ;
#28637=VECTOR ( 'NONE', #2198, 1000.000000000000000 ) ;
#28638=LINE ( 'NONE', #7689, #9405 ) ;
#28639=DIRECTION ( 'NONE',  ( 0.5877852522924731371, 0.000000000000000000, 0.8090169943749474513 ) ) ;
#28640=VECTOR ( 'NONE', #12558, 1000.000000000000000 ) ;
#28641=CARTESIAN_POINT ( 'NONE',  ( 134.5152310637605524, -4.999999999999981348, -13.05155085951650840 ) ) ;
#28642=CARTESIAN_POINT ( 'NONE',  ( 172.7287565553229456, -1.999999999999970468, -39.49999999999997868 ) ) ;
#28646=EDGE_CURVE ( 'NONE', #2890, #7231, #6575, .T. ) ;
#28648=ORIENTED_EDGE ( 'NONE', *, *, #27520, .F. ) ;
#28650=CARTESIAN_POINT ( 'NONE',  ( 154.7287565553230024, -10.00000000000000000, -25.16025403784440329 ) ) ;
#28652=DIRECTION ( 'NONE',  ( 0.3090169943749475623, 8.338696094058001131E-17, 0.9510565162951536422 ) ) ;
#28655=DIRECTION ( 'NONE',  ( -0.5877852522924731371, -1.586114251531760235E-16, 0.8090169943749474513 ) ) ;
#28658=DIRECTION ( 'NONE',  ( 0.9510565162951536422, 0.000000000000000000, -0.3090169943749475623 ) ) ;
#28660=VECTOR ( 'NONE', #17717, 1000.000000000000000 ) ;
#28661=DIRECTION ( 'NONE',  ( -1.110223024625156540E-16, 0.000000000000000000, -1.000000000000000000 ) ) ;
#28663=ADVANCED_FACE ( 'NONE', ( #1700 ), #8985, .T. ) ;
#28665=EDGE_CURVE ( 'NONE', #10103, #9448, #2012, .T. ) ;
#28666=ADVANCED_FACE ( 'NONE', ( #11429 ), #18306, .F. ) ;
#28668=ORIENTED_EDGE ( 'NONE', *, *, #1895, .F. ) ;
#28673=ORIENTED_EDGE ( 'NONE', *, *, #17041, .F. ) ;
#28675=VECTOR ( 'NONE', #28131, 1000.000000000000000 ) ;
#28676=DIRECTION ( 'NONE',  ( 0.9510565162951535312, 2.566386769018988816E-16, -0.3090169943749475623 ) ) ;
#28677=CARTESIAN_POINT ( 'NONE',  ( 144.5152310637605808, -1.999999999999977129, -21.71180489736091346 ) ) ;
#28679=LINE ( 'NONE', #3759, #28197 ) ;
#28680=DIRECTION ( 'NONE',  ( 0.3090169943749472292, 8.338696094057992503E-17, -0.9510565162951536422 ) ) ;
#28684=CARTESIAN_POINT ( 'NONE',  ( 157.2287565553230024, -1.999999999999973133, -29.49038105676660493 ) ) ;
#28685=DIRECTION ( 'NONE',  ( -0.9510565162951536422, -2.566386769018988816E-16, -0.3090169943749472292 ) ) ;
#28689=VERTEX_POINT ( 'NONE', #18464 ) ;
#28690=EDGE_LOOP ( 'NONE', ( #10849, #28617, #11524, #22477 ) ) ;
#28691=FACE_OUTER_BOUND ( 'NONE', #8736, .T. ) ;
#28693=ADVANCED_FACE ( 'NONE', ( #10984 ), #27816, .T. ) ;
#28694=EDGE_CURVE ( 'NONE', #22122, #9309, #23193, .T. ) ;
#28695=VECTOR ( 'NONE', #25956, 1000.000000000000000 ) ;
#28697=ORIENTED_EDGE ( 'NONE', *, *, #21341, .T. ) ;
#28698=VERTEX_POINT ( 'NONE', #19206 ) ;
#28699=ADVANCED_FACE ( 'NONE', ( #4722 ), #28562, .T. ) ;
#28703=VECTOR ( 'NONE', #6449, 1000.000000000000000 ) ;
#28706=CARTESIAN_POINT ( 'NONE',  ( 149.7287565553230024, -1.999999999999975797, -16.50000000000000355 ) ) ;
#28707=CARTESIAN_POINT ( 'NONE',  ( 174.7287565553228603, -9.999999999999996447, -7.839745962155603820 ) ) ;
#28708=LINE ( 'NONE', #7756, #21567 ) ;
#28709=CARTESIAN_POINT ( 'NONE',  ( 130.7287565553229456, -4.999999999999983125, 3.500000000000003109 ) ) ;
#28710=LINE ( 'NONE', #19503, #28457 ) ;
#28711=CARTESIAN_POINT ( 'NONE',  ( 141.1922820468854525, -10.00000000000000533, -13.59645775552055902 ) ) ;
#28713=CARTESIAN_POINT ( 'NONE',  ( 148.6922820468854525, -1.999999999999976241, -26.58683881228715862 ) ) ;
#28714=LINE ( 'NONE', #12638, #28516 ) ;
#28716=DIRECTION ( 'NONE',  ( 0.5877852522924731371, 1.586114251531760728E-16, 0.8090169943749474513 ) ) ;
#28718=VECTOR ( 'NONE', #6715, 1000.000000000000000 ) ;
#28719=ORIENTED_EDGE ( 'NONE', *, *, #20740, .F. ) ;
#28721=DIRECTION ( 'NONE',  ( 1.000000000000000000, 2.698458740408365879E-16, -1.110223024625156540E-16 ) ) ;
#28724=LINE ( 'NONE', #28426, #15061 ) ;
#28725=VECTOR ( 'NONE', #21493, 1000.000000000000000 ) ;
#28726=VERTEX_POINT ( 'NONE', #18915 ) ;
#28727=ORIENTED_EDGE ( 'NONE', *, *, #17621, .F. ) ;
#28728=VECTOR ( 'NONE', #2085, 999.9999999999998863 ) ;
#28729=VERTEX_POINT ( 'NONE', #7323 ) ;
#28733=CARTESIAN_POINT ( 'NONE',  ( 12.98686435253176796, -5.000000000000014211, 39.96945861731516203 ) ) ;
#28734=ORIENTED_EDGE ( 'NONE', *, *, #10861, .F. ) ;
#28736=LINE ( 'NONE', #1087, #3767 ) ;
#28737=ORIENTED_EDGE ( 'NONE', *, *, #18589, .F. ) ;
#28738=EDGE_CURVE ( 'NONE', #13474, #24401, #7032, .T. ) ;
#28746=VERTEX_POINT ( 'NONE', #16022 ) ;
#28747=ORIENTED_EDGE ( 'NONE', *, *, #13280, .F. ) ;
#28754=VECTOR ( 'NONE', #17213, 1000.000000000000000 ) ;
#28756=ORIENTED_EDGE ( 'NONE', *, *, #8530, .T. ) ;
#28758=CARTESIAN_POINT ( 'NONE',  ( 162.0152310637604103, -1.999999999999973577, -0.06116980274991495881 ) ) ;
#28759=LINE ( 'NONE', #1243, #28440 ) ;
#28760=EDGE_CURVE ( 'NONE', #26011, #5942, #8994, .T. ) ;
#28762=DIRECTION ( 'NONE',  ( -2.698458740408365879E-16, 1.000000000000000000, 0.000000000000000000 ) ) ;
#28763=LINE ( 'NONE', #24748, #23856 ) ;
#28768=VECTOR ( 'NONE', #28307, 1000.000000000000000 ) ;
#28772=ORIENTED_EDGE ( 'NONE', *, *, #16833, .F. ) ;
#28774=CARTESIAN_POINT ( 'NONE',  ( 157.2287565553230024, -10.00000000000000000, -29.49038105676660493 ) ) ;
#28775=DIRECTION ( 'NONE',  ( -2.698458740408365879E-16, 1.000000000000000000, 0.000000000000000000 ) ) ;
#28777=VECTOR ( 'NONE', #8202, 1000.000000000000000 ) ;
#28778=EDGE_LOOP ( 'NONE', ( #24999, #22994, #4603, #25129 ) ) ;
#28779=DIRECTION ( 'NONE',  ( 0.5877852522924731371, 1.586114251531760728E-16, 0.8090169943749474513 ) ) ;
#28780=ORIENTED_EDGE ( 'NONE', *, *, #29830, .T. ) ;
#28782=ORIENTED_EDGE ( 'NONE', *, *, #28881, .F. ) ;
#28785=FACE_OUTER_BOUND ( 'NONE', #11319, .T. ) ;
#28787=VERTEX_POINT ( 'NONE', #4140 ) ;
#28791=LINE ( 'NONE', #3129, #28936 ) ;
#28792=VERTEX_POINT ( 'NONE', #4440 ) ;
#28795=LINE ( 'NONE', #9506, #5964 ) ;
#28798=DIRECTION ( 'NONE',  ( -0.5877852522924731371, -1.586114251531760728E-16, -0.8090169943749474513 ) ) ;
#28801=EDGE_CURVE ( 'NONE', #29449, #21526, #22608, .T. ) ;
#28802=CARTESIAN_POINT ( 'NONE',  ( 147.0152310637605240, -1.999999999999977573, 1.702185954127501066 ) ) ;
#28803=DIRECTION ( 'NONE',  ( -2.698458740408365879E-16, 1.000000000000000000, 0.000000000000000000 ) ) ;
#28805=LINE ( 'NONE', #10273, #23149 ) ;
#28806=EDGE_CURVE ( 'NONE', #19636, #9848, #9752, .T. ) ;
#28811=ORIENTED_EDGE ( 'NONE', *, *, #7021, .T. ) ;
#28813=LINE ( 'NONE', #26489, #5307 ) ;
#28816=LINE ( 'NONE', #15007, #6419 ) ;
#28817=DIRECTION ( 'NONE',  ( 1.000000000000000000, 2.698458740408365879E-16, -1.110223024625156540E-16 ) ) ;
#28819=ORIENTED_EDGE ( 'NONE', *, *, #4537, .F. ) ;
#28820=CARTESIAN_POINT ( 'NONE',  ( 130.7287565553229456, -9.999999999999982236, 3.500000000000003109 ) ) ;
#28822=AXIS2_PLACEMENT_3D ( 'NONE', #28851, #12912, #7889 ) ;
#28824=DIRECTION ( 'NONE',  ( 0.3090169943749472292, 8.338696094057992503E-17, -0.9510565162951536422 ) ) ;
#28827=EDGE_LOOP ( 'NONE', ( #19645, #7105, #29394, #915, #15960 ) ) ;
#28832=VECTOR ( 'NONE', #7817, 1000.000000000000000 ) ;
#28833=ORIENTED_EDGE ( 'NONE', *, *, #23807, .F. ) ;
#28834=CARTESIAN_POINT ( 'NONE',  ( 152.0152310637605524, -4.999999999999976907, -1.687708096207002932E-14 ) ) ;
#28835=ORIENTED_EDGE ( 'NONE', *, *, #28102, .F. ) ;
#28836=EDGE_CURVE ( 'NONE', #10847, #23159, #25640, .T. ) ;
#28837=VECTOR ( 'NONE', #17809, 999.9999999999998863 ) ;
#28838=CARTESIAN_POINT ( 'NONE',  ( 134.5152310637605524, -10.00000000000000533, -4.391296821672111328 ) ) ;
#28839=ORIENTED_EDGE ( 'NONE', *, *, #22911, .T. ) ;
#28840=CARTESIAN_POINT ( 'NONE',  ( 125.7287565553229172, -9.999999999999982236, -33.50000000000000000 ) ) ;
#28841=EDGE_CURVE ( 'NONE', #26554, #21526, #26258, .T. ) ;
#28843=DIRECTION ( 'NONE',  ( -0.5877852522924731371, 0.000000000000000000, 0.8090169943749474513 ) ) ;
#28848=LINE ( 'NONE', #15192, #21983 ) ;
#28849=DIRECTION ( 'NONE',  ( 0.5877852522924731371, 1.586114251531760728E-16, -0.8090169943749474513 ) ) ;
#28851=CARTESIAN_POINT ( 'NONE',  ( 133.7287565553229456, -1.999999999999988010, 0.5000000000000029976 ) ) ;
#28852=LINE ( 'NONE', #17199, #15880 ) ;
#28853=VECTOR ( 'NONE', #28535, 1000.000000000000000 ) ;
#28854=ORIENTED_EDGE ( 'NONE', *, *, #6821, .F. ) ;
#28855=AXIS2_PLACEMENT_3D ( 'NONE', #27979, #16482, #13596 ) ;
#28856=DIRECTION ( 'NONE',  ( -0.8090169943749474513, -2.183098979609982436E-16, 0.5877852522924731371 ) ) ;
#28857=CARTESIAN_POINT ( 'NONE',  ( 162.0152310637604671, -1.999999999999973133, -6.958068083716895558 ) ) ;
#28858=ORIENTED_EDGE ( 'NONE', *, *, #11995, .T. ) ;
#28859=CARTESIAN_POINT ( 'NONE',  ( 159.5152310637604955, -1.999999999999973133, -21.71180489736091346 ) ) ;
#28860=ORIENTED_EDGE ( 'NONE', *, *, #12933, .F. ) ;
#28861=ORIENTED_EDGE ( 'NONE', *, *, #8153, .F. ) ;
#28862=ORIENTED_EDGE ( 'NONE', *, *, #15518, .F. ) ;
#28867=DIRECTION ( 'NONE',  ( -0.5877852522924731371, -1.586114251531760728E-16, -0.8090169943749474513 ) ) ;
#28868=CARTESIAN_POINT ( 'NONE',  ( 103.2426971230879786, -4.999999999999989342, 75.01021016590013346 ) ) ;
#28869=CARTESIAN_POINT ( 'NONE',  ( 139.5152310637606092, -10.00000000000000533, -11.28819510263909542 ) ) ;
#28871=DIRECTION ( 'NONE',  ( -0.9510565162951536422, 0.000000000000000000, -0.3090169943749472292 ) ) ;
#28872=CIRCLE ( 'NONE', #18097, 8.000000000000007105 ) ;
#28873=DIRECTION ( 'NONE',  ( -2.698458740408365879E-16, 1.000000000000000000, 0.000000000000000000 ) ) ;
#28875=VECTOR ( 'NONE', #15771, 1000.000000000000000 ) ;
#28876=EDGE_CURVE ( 'NONE', #21691, #6733, #21511, .T. ) ;
#28877=DIRECTION ( 'NONE',  ( 0.5877852522924731371, 1.586114251531760728E-16, -0.8090169943749474513 ) ) ;
#28878=CARTESIAN_POINT ( 'NONE',  ( 144.5152310637605524, -4.999999999999978684, -2.627941064794695691 ) ) ;
#28879=ADVANCED_FACE ( 'NONE', ( #25801 ), #11742, .T. ) ;
#28880=EDGE_CURVE ( 'NONE', #27071, #929, #21060, .T. ) ;
#28881=EDGE_CURVE ( 'NONE', #7141, #8863, #28724, .T. ) ;
#28884=ORIENTED_EDGE ( 'NONE', *, *, #29866, .F. ) ;
#28889=FACE_BOUND ( 'NONE', #7194, .T. ) ;
#28890=VERTEX_POINT ( 'NONE', #618 ) ;
#28891=VERTEX_POINT ( 'NONE', #18770 ) ;
#28892=CARTESIAN_POINT ( 'NONE',  ( 174.5152310637604671, -4.999999999999969802, -19.94844914048349693 ) ) ;
#28894=PLANE ( 'NONE',  #9627 ) ;
#28895=ORIENTED_EDGE ( 'NONE', *, *, #23730, .F. ) ;
#28896=CARTESIAN_POINT ( 'NONE',  ( 153.6922820468853388, -1.999999999999975797, 2.247092850131519715 ) ) ;
#28897=VERTEX_POINT ( 'NONE', #14479 ) ;
#28899=ORIENTED_EDGE ( 'NONE', *, *, #22453, .T. ) ;
#28902=CARTESIAN_POINT ( 'NONE',  ( 154.7287565553229172, -1.999999999999975353, 0.8205080756887930260 ) ) ;
#28906=VERTEX_POINT ( 'NONE', #12046 ) ;
#28909=CARTESIAN_POINT ( 'NONE',  ( 147.0152310637605524, -1.999999999999976685, -17.38167787843871182 ) ) ;
#28911=VECTOR ( 'NONE', #4006, 1000.000000000000000 ) ;
#28912=EDGE_CURVE ( 'NONE', #11271, #5507, #9602, .T. ) ;
#28913=EDGE_CURVE ( 'NONE', #12691, #23292, #7478, .T. ) ;
#28917=CARTESIAN_POINT ( 'NONE',  ( 152.2287565553230309, -10.00000000000000178, -29.49038105676660493 ) ) ;
#28920=LINE ( 'NONE', #12380, #15858 ) ;
#28921=VERTEX_POINT ( 'NONE', #7182 ) ;
#28923=VECTOR ( 'NONE', #11911, 1000.000000000000000 ) ;
#28925=CARTESIAN_POINT ( 'NONE',  ( 17.19644251272489299, -5.000000000000013323, -52.92520801939408415 ) ) ;
#28926=CARTESIAN_POINT ( 'NONE',  ( 144.5152310637605524, -10.00000000000000355, -2.627941064794695691 ) ) ;
#28927=FACE_OUTER_BOUND ( 'NONE', #2246, .T. ) ;
#28929=VERTEX_POINT ( 'NONE', #16474 ) ;
#28931=ORIENTED_EDGE ( 'NONE', *, *, #12336, .T. ) ;
#28934=ORIENTED_EDGE ( 'NONE', *, *, #13486, .F. ) ;
#28935=DIRECTION ( 'NONE',  ( 0.5877852522924731371, 1.586114251531760728E-16, 0.8090169943749474513 ) ) ;
#28936=VECTOR ( 'NONE', #14537, 1000.000000000000000 ) ;
#28938=DIRECTION ( 'NONE',  ( -1.110223024625156540E-16, 0.000000000000000000, -1.000000000000000000 ) ) ;
#28939=ADVANCED_FACE ( 'NONE', ( #4881, #23817, #14177, #23504, #16927, #2915, #2613, #12195, #11888, #318, #7333, #21203, #12950, #29026, #6091, #8371, #26408, #19516, #911, #15387, #21813, #29501, #17375, #12646, #8064, #1218, #24720, #1372, #14923, #10357, #3807, #17678, #29344, #13098, #5645, #19973, #8215, #17231, #22427, #17085, #12801, #28889, #5945, #26720, #21965, #10664, #27034, #1530, #10501, #10813, #24565, #17526, #24263, #15230, #20121, #19813, #26881, #3654, #1079, #19661, #14770, #10202, #5792, #3360, #5488, #24113, #3212, #12490, #7921, #15074, #29179, #26558, #24413, #3508, #22116, #22263, #1833, #25460, #9107, #20710, #4551, #3961, #4107, #13705, #13552, #22729 ), #20568, .T. ) ;
#28943=ORIENTED_EDGE ( 'NONE', *, *, #17654, .T. ) ;
#28944=EDGE_LOOP ( 'NONE', ( #7488, #20695, #5197, #3424, #20767 ) ) ;
#28947=DIRECTION ( 'NONE',  ( 0.5877852522924731371, 1.586114251531760728E-16, 0.8090169943749474513 ) ) ;
#28949=CARTESIAN_POINT ( 'NONE',  ( 147.0152310637605524, -10.00000000000000178, -6.958068083716895558 ) ) ;
#28951=VECTOR ( 'NONE', #26705, 1000.000000000000000 ) ;
#28952=EDGE_LOOP ( 'NONE', ( #11808, #21213, #2024, #26890, #17981 ) ) ;
#28956=ORIENTED_EDGE ( 'NONE', *, *, #6639, .T. ) ;
#28961=CARTESIAN_POINT ( 'NONE',  ( 132.0152310637605524, -4.999999999999982236, -1.465663491281971624E-14 ) ) ;
#28964=ORIENTED_EDGE ( 'NONE', *, *, #3481, .T. ) ;
#28965=ORIENTED_EDGE ( 'NONE', *, *, #17073, .F. ) ;
#28966=DIRECTION ( 'NONE',  ( 1.110223024625156540E-16, 2.995891024602366092E-32, 1.000000000000000000 ) ) ;
#28968=VECTOR ( 'NONE', #4254, 1000.000000000000000 ) ;
#28970=CARTESIAN_POINT ( 'NONE',  ( 147.2287565553229740, -10.00000000000000355, -3.509618943233403510 ) ) ;
#28972=CARTESIAN_POINT ( 'NONE',  ( 149.7287565553230309, -10.00000000000000178, -33.82050807568879947 ) ) ;
#28974=ORIENTED_EDGE ( 'NONE', *, *, #7623, .T. ) ;
#28975=CARTESIAN_POINT ( 'NONE',  ( 136.1922820468854241, -1.999999999999980016, -2.083034168790677043 ) ) ;
#28976=EDGE_CURVE ( 'NONE', #24463, #4011, #23030, .T. ) ;
#28979=ADVANCED_FACE ( 'NONE', ( #11116 ), #8670, .T. ) ;
#28981=AXIS2_PLACEMENT_3D ( 'NONE', #2079, #6643, #4502 ) ;
#28982=ORIENTED_EDGE ( 'NONE', *, *, #25616, .F. ) ;
#28984=DIRECTION ( 'NONE',  ( -0.5877852522924731371, -1.586114251531760728E-16, -0.8090169943749474513 ) ) ;
#28990=AXIS2_PLACEMENT_3D ( 'NONE', #27960, #11575, #21191 ) ;
#28991=CARTESIAN_POINT ( 'NONE',  ( 133.6922820468854241, -10.00000000000000711, -9.266330736598357376 ) ) ;
#28992=CARTESIAN_POINT ( 'NONE',  ( 161.1922820468853388, -1.999999999999973577, -13.59645775552055902 ) ) ;
#28994=CARTESIAN_POINT ( 'NONE',  ( 176.1922820468852819, -9.999999999999994671, -13.59645775552055902 ) ) ;
#28995=CARTESIAN_POINT ( 'NONE',  ( 142.0152310637605808, -1.999999999999978462, -6.958068083716895558 ) ) ;
#28996=VERTEX_POINT ( 'NONE', #17975 ) ;
#28998=DIRECTION ( 'NONE',  ( -2.698458740408365879E-16, 1.000000000000000000, 0.000000000000000000 ) ) ;
#29000=CARTESIAN_POINT ( 'NONE',  ( 147.0152310637605808, -4.999999999999977796, -26.04193191628311155 ) ) ;
#29001=ORIENTED_EDGE ( 'NONE', *, *, #4063, .F. ) ;
#29004=ADVANCED_FACE ( 'NONE', ( #18127 ), #13840, .T. ) ;
#29006=EDGE_CURVE ( 'NONE', #23288, #27071, #15541, .T. ) ;
#29008=DIRECTION ( 'NONE',  ( 0.5877852522924731371, 0.000000000000000000, 0.8090169943749474513 ) ) ;
#29010=ADVANCED_FACE ( 'NONE', ( #13259 ), #15834, .T. ) ;
#29011=CARTESIAN_POINT ( 'NONE',  ( 134.7287565553230024, -1.999999999999980460, 0.8205080756887930260 ) ) ;
#29012=VECTOR ( 'NONE', #1481, 1000.000000000000000 ) ;
#29013=EDGE_LOOP ( 'NONE', ( #2036, #217, #16214, #1232 ) ) ;
#29014=LINE ( 'NONE', #26546, #638 ) ;
#29015=LINE ( 'NONE', #5323, #10370 ) ;
#29016=DIRECTION ( 'NONE',  ( 0.9510565162951536422, 0.000000000000000000, -0.3090169943749475623 ) ) ;
#29017=LINE ( 'NONE', #5631, #14154 ) ;
#29018=CARTESIAN_POINT ( 'NONE',  ( 167.0152310637604671, -9.999999999999996447, -17.38167787843871182 ) ) ;
#29019=VECTOR ( 'NONE', #9639, 1000.000000000000000 ) ;
#29026=FACE_BOUND ( 'NONE', #10548, .T. ) ;
#29027=ORIENTED_EDGE ( 'NONE', *, *, #520, .T. ) ;
#29028=ORIENTED_EDGE ( 'NONE', *, *, #20404, .F. ) ;
#29029=CARTESIAN_POINT ( 'NONE',  ( 176.1922820468852819, -1.999999999999969580, -13.59645775552055902 ) ) ;
#29032=CARTESIAN_POINT ( 'NONE',  ( 139.7287565553230309, -10.00000000000000533, -33.82050807568879947 ) ) ;
#29033=ORIENTED_EDGE ( 'NONE', *, *, #7837, .F. ) ;
#29034=DIRECTION ( 'NONE',  ( -0.9510565162951536422, -2.566386769018988816E-16, -0.3090169943749472292 ) ) ;
#29037=ORIENTED_EDGE ( 'NONE', *, *, #28106, .T. ) ;
#29040=EDGE_CURVE ( 'NONE', #22270, #11002, #1984, .T. ) ;
#29041=CARTESIAN_POINT ( 'NONE',  ( 130.7287565553229172, -4.999999999999983125, -36.50000000000000711 ) ) ;
#29042=ADVANCED_FACE ( 'NONE', ( #20863 ), #13401, .T. ) ;
#29044=EDGE_CURVE ( 'NONE', #24164, #16231, #4407, .T. ) ;
#29045=EDGE_CURVE ( 'NONE', #10906, #27188, #29951, .T. ) ;
#29050=LINE ( 'NONE', #19835, #24690 ) ;
#29051=FACE_OUTER_BOUND ( 'NONE', #8016, .T. ) ;
#29052=VECTOR ( 'NONE', #315, 1000.000000000000000 ) ;
#29054=DIRECTION ( 'NONE',  ( 0.9510565162951535312, 2.566386769018988816E-16, -0.3090169943749475623 ) ) ;
#29055=LINE ( 'NONE', #1106, #2423 ) ;
#29057=DIRECTION ( 'NONE',  ( 0.3090169943749475623, 8.338696094058001131E-17, 0.9510565162951536422 ) ) ;
#29059=DIRECTION ( 'NONE',  ( -2.698458740408365879E-16, 1.000000000000000000, 0.000000000000000000 ) ) ;
#29061=EDGE_CURVE ( 'NONE', #1409, #13253, #1678, .T. ) ;
#29062=VERTEX_POINT ( 'NONE', #27347 ) ;
#29063=CARTESIAN_POINT ( 'NONE',  ( 136.1922820468854241, -1.999999999999980460, -4.936203717676158398 ) ) ;
#29064=ORIENTED_EDGE ( 'NONE', *, *, #23846, .F. ) ;
#29066=ORIENTED_EDGE ( 'NONE', *, *, #24880, .F. ) ;
#29069=DIRECTION ( 'NONE',  ( 0.9510565162951535312, 2.566386769018988816E-16, -0.3090169943749475623 ) ) ;
#29071=ORIENTED_EDGE ( 'NONE', *, *, #17232, .F. ) ;
#29073=VERTEX_POINT ( 'NONE', #6545 ) ;
#29077=ORIENTED_EDGE ( 'NONE', *, *, #10520, .F. ) ;
#29078=EDGE_CURVE ( 'NONE', #22429, #29689, #20267, .T. ) ;
#29080=VECTOR ( 'NONE', #2546, 1000.000000000000000 ) ;
#29081=LINE ( 'NONE', #15279, #8155 ) ;
#29083=ADVANCED_FACE ( 'NONE', ( #29654 ), #15693, .F. ) ;
#29084=EDGE_LOOP ( 'NONE', ( #23984, #13345, #9570, #27944 ) ) ;
#29086=LINE ( 'NONE', #8568, #5702 ) ;
#29090=ORIENTED_EDGE ( 'NONE', *, *, #15689, .F. ) ;
#29097=DIRECTION ( 'NONE',  ( 0.000000000000000000, 0.7071067811865456854, 0.7071067811865493491 ) ) ;
#29098=LINE ( 'NONE', #24627, #20694 ) ;
#29102=ORIENTED_EDGE ( 'NONE', *, *, #20740, .T. ) ;
#29103=FACE_OUTER_BOUND ( 'NONE', #1070, .T. ) ;
#29104=AXIS2_PLACEMENT_3D ( 'NONE', #23269, #2379, #80 ) ;
#29105=DIRECTION ( 'NONE',  ( -2.698458740408365879E-16, 1.000000000000000000, 0.000000000000000000 ) ) ;
#29107=CARTESIAN_POINT ( 'NONE',  ( 129.5152310637605808, -1.999999999999982236, -19.94844914048349338 ) ) ;
#29109=LINE ( 'NONE', #19447, #28331 ) ;
#29112=CARTESIAN_POINT ( 'NONE',  ( 13.53844545036150393, -5.000000000000014211, -41.66705068152283786 ) ) ;
#29115=CARTESIAN_POINT ( 'NONE',  ( 167.0152310637604671, -9.999999999999998224, -6.958068083716895558 ) ) ;
#29116=VECTOR ( 'NONE', #22850, 1000.000000000000000 ) ;
#29118=LINE ( 'NONE', #19602, #11073 ) ;
#29120=ORIENTED_EDGE ( 'NONE', *, *, #26142, .F. ) ;
#29128=PLANE ( 'NONE',  #8934 ) ;
#29129=EDGE_LOOP ( 'NONE', ( #8311, #26385, #12360, #18199 ) ) ;
#29130=CARTESIAN_POINT ( 'NONE',  ( 142.0152310637605808, -4.999999999999979572, -1.576685793744487594E-14 ) ) ;
#29131=CARTESIAN_POINT ( 'NONE',  ( 148.6922820468854525, -10.00000000000000178, -26.58683881228715862 ) ) ;
#29132=LINE ( 'NONE', #15646, #9451 ) ;
#29133=VECTOR ( 'NONE', #13341, 1000.000000000000000 ) ;
#29135=EDGE_CURVE ( 'NONE', #1558, #10211, #16285, .T. ) ;
#29137=VECTOR ( 'NONE', #921, 1000.000000000000000 ) ;
#29140=CARTESIAN_POINT ( 'NONE',  ( 176.1922820468852819, -1.999999999999969358, -19.40354224447947473 ) ) ;
#29145=ORIENTED_EDGE ( 'NONE', *, *, #14205, .F. ) ;
#29146=DIRECTION ( 'NONE',  ( -2.698458740408365879E-16, 1.000000000000000000, 0.000000000000000000 ) ) ;
#29147=CARTESIAN_POINT ( 'NONE',  ( 159.5152310637604671, -1.999999999999974021, -2.627941064794695691 ) ) ;
#29148=CARTESIAN_POINT ( 'NONE',  ( 162.2287565553229172, -4.999999999999973355, -3.509618943233400401 ) ) ;
#29149=VERTEX_POINT ( 'NONE', #6996 ) ;
#29150=VERTEX_POINT ( 'NONE', #7293 ) ;
#29151=VERTEX_POINT ( 'NONE', #21474 ) ;
#29156=LINE ( 'NONE', #26541, #21858 ) ;
#29157=CARTESIAN_POINT ( 'NONE',  ( 157.0152310637605240, -4.999999999999975131, -1.743219247438260444E-14 ) ) ;
#29158=DIRECTION ( 'NONE',  ( 0.5877852522924731371, 1.586114251531760728E-16, 0.8090169943749474513 ) ) ;
#29159=VECTOR ( 'NONE', #16756, 1000.000000000000000 ) ;
#29160=ORIENTED_EDGE ( 'NONE', *, *, #13523, .F. ) ;
#29161=CARTESIAN_POINT ( 'NONE',  ( 173.6922820468852535, -9.999999999999996447, 2.247092850131519715 ) ) ;
#29163=ORIENTED_EDGE ( 'NONE', *, *, #17546, .F. ) ;
#29164=CARTESIAN_POINT ( 'NONE',  ( 147.0152310637605808, -1.999999999999976685, -15.61832212156129707 ) ) ;
#29165=LINE ( 'NONE', #12482, #15289 ) ;
#29170=ORIENTED_EDGE ( 'NONE', *, *, #22591, .T. ) ;
#29174=VERTEX_POINT ( 'NONE', #19036 ) ;
#29176=EDGE_CURVE ( 'NONE', #1558, #22770, #16439, .T. ) ;
#29179=FACE_BOUND ( 'NONE', #29960, .T. ) ;
#29180=VERTEX_POINT ( 'NONE', #584 ) ;
#29182=AXIS2_PLACEMENT_3D ( 'NONE', #1578, #8868, #18181 ) ;
#29183=DIRECTION ( 'NONE',  ( -0.9510565162951536422, -2.566386769018988816E-16, -0.3090169943749472292 ) ) ;
#29185=FACE_OUTER_BOUND ( 'NONE', #2405, .T. ) ;
#29187=LINE ( 'NONE', #14934, #16910 ) ;
#29188=ORIENTED_EDGE ( 'NONE', *, *, #5438, .F. ) ;
#29190=ORIENTED_EDGE ( 'NONE', *, *, #28665, .F. ) ;
#29193=LINE ( 'NONE', #21829, #8650 ) ;
#29194=ORIENTED_EDGE ( 'NONE', *, *, #6986, .T. ) ;
#29200=DIRECTION ( 'NONE',  ( -2.698458740408365879E-16, 1.000000000000000000, 0.000000000000000000 ) ) ;
#29201=ORIENTED_EDGE ( 'NONE', *, *, #18481, .T. ) ;
#29203=PLANE ( 'NONE',  #7793 ) ;
#29204=EDGE_CURVE ( 'NONE', #25168, #20384, #2719, .T. ) ;
#29205=CARTESIAN_POINT ( 'NONE',  ( 167.2287565553229456, -1.999999999999970912, -20.83012701892220520 ) ) ;
#29206=CARTESIAN_POINT ( 'NONE',  ( 172.7287565553229456, -1.999999999999974021, 0.5000000000000029976 ) ) ;
#29207=ORIENTED_EDGE ( 'NONE', *, *, #16897, .T. ) ;
#29208=ADVANCED_FACE ( 'NONE', ( #26224 ), #5304, .T. ) ;
#29209=DIRECTION ( 'NONE',  ( -2.908569913943825554E-16, 1.000000000000000000, 0.000000000000000000 ) ) ;
#29210=EDGE_CURVE ( 'NONE', #7358, #27200, #28394, .T. ) ;
#29212=DIRECTION ( 'NONE',  ( -0.9510565162951536422, 0.000000000000000000, -0.3090169943749472292 ) ) ;
#29214=ORIENTED_EDGE ( 'NONE', *, *, #7665, .F. ) ;
#29216=ORIENTED_EDGE ( 'NONE', *, *, #9443, .F. ) ;
#29219=CARTESIAN_POINT ( 'NONE',  ( 176.1922820468852535, -9.999999999999994671, -2.083034168790677043 ) ) ;
#29220=CARTESIAN_POINT ( 'NONE',  ( 175.7287565553229456, -4.999999999999970690, -33.50000000000000000 ) ) ;
#29221=EDGE_LOOP ( 'NONE', ( #5830, #15286, #2056, #18595, #21547 ) ) ;
#29222=VERTEX_POINT ( 'NONE', #14590 ) ;
#29226=VECTOR ( 'NONE', #24697, 1000.000000000000000 ) ;
#29229=ORIENTED_EDGE ( 'NONE', *, *, #27696, .F. ) ;
#29230=ORIENTED_EDGE ( 'NONE', *, *, #612, .F. ) ;
#29235=VECTOR ( 'NONE', #9577, 1000.000000000000000 ) ;
#29236=LINE ( 'NONE', #1580, #17378 ) ;
#29240=VERTEX_POINT ( 'NONE', #25763 ) ;
#29241=EDGE_CURVE ( 'NONE', #20829, #13408, #16595, .T. ) ;
#29242=LINE ( 'NONE', #7983, #1576 ) ;
#29243=DIRECTION ( 'NONE',  ( -0.9510565162951536422, -2.566386769018988323E-16, 0.3090169943749475623 ) ) ;
#29244=DIRECTION ( 'NONE',  ( 0.9510565162951536422, 2.566386769018988816E-16, 0.3090169943749472292 ) ) ;
#29245=FACE_OUTER_BOUND ( 'NONE', #2205, .T. ) ;
#29246=VECTOR ( 'NONE', #5971, 1000.000000000000000 ) ;
#29247=CARTESIAN_POINT ( 'NONE',  ( 167.2287565553230024, -4.999999999999972466, -29.49038105676661559 ) ) ;
#29248=EDGE_CURVE ( 'NONE', #23660, #14857, #21168, .T. ) ;
#29249=EDGE_CURVE ( 'NONE', #4536, #17531, #12006, .T. ) ;
#29250=LINE ( 'NONE', #13169, #9980 ) ;
#29252=ORIENTED_EDGE ( 'NONE', *, *, #29293, .F. ) ;
#29256=CIRCLE ( 'NONE', #5312, 3.000000000000002665 ) ;
#29259=ORIENTED_EDGE ( 'NONE', *, *, #21975, .T. ) ;
#29261=PLANE ( 'NONE',  #14062 ) ;
#29262=LINE ( 'NONE', #24193, #8236 ) ;
#29263=FACE_OUTER_BOUND ( 'NONE', #15238, .T. ) ;
#29267=ORIENTED_EDGE ( 'NONE', *, *, #29655, .F. ) ;
#29270=LINE ( 'NONE', #8305, #791 ) ;
#29271=FACE_OUTER_BOUND ( 'NONE', #19000, .T. ) ;
#29273=CARTESIAN_POINT ( 'NONE',  ( 156.1922820468853956, -1.999999999999974465, -22.25671179336496053 ) ) ;
#29275=EDGE_LOOP ( 'NONE', ( #18120, #25008, #5795, #11000, #17034 ) ) ;
#29277=VECTOR ( 'NONE', #27375, 1000.000000000000000 ) ;
#29280=VECTOR ( 'NONE', #1967, 1000.000000000000000 ) ;
#29282=LINE ( 'NONE', #17771, #1015 ) ;
#29283=EDGE_LOOP ( 'NONE', ( #22446, #17177, #16493, #2981 ) ) ;
#29284=FACE_OUTER_BOUND ( 'NONE', #10128, .T. ) ;
#29285=EDGE_LOOP ( 'NONE', ( #14750, #25303, #8962, #525 ) ) ;
#29286=DIRECTION ( 'NONE',  ( 8.163404592832029035E-16, 2.202861047501738386E-31, 1.000000000000000000 ) ) ;
#29287=LINE ( 'NONE', #24366, #10105 ) ;
#29288=ADVANCED_FACE ( 'NONE', ( #14885 ), #26685, .T. ) ;
#29289=DIRECTION ( 'NONE',  ( 0.5877852522924731371, 0.000000000000000000, 0.8090169943749474513 ) ) ;
#29290=EDGE_CURVE ( 'NONE', #11499, #29523, #5760, .T. ) ;
#29293=EDGE_CURVE ( 'NONE', #12642, #11550, #21780, .T. ) ;
#29295=LINE ( 'NONE', #3764, #10222 ) ;
#29298=LINE ( 'NONE', #22685, #22211 ) ;
#29301=CARTESIAN_POINT ( 'NONE',  ( 172.2287565553228603, -4.999999999999970690, -3.509618943233400401 ) ) ;
#29302=CARTESIAN_POINT ( 'NONE',  ( 144.5152310637605808, -10.00000000000000178, -30.37205893520530964 ) ) ;
#29303=VECTOR ( 'NONE', #271, 1000.000000000000000 ) ;
#29305=PLANE ( 'NONE',  #17066 ) ;
#29306=CARTESIAN_POINT ( 'NONE',  ( 136.1922820468854241, -1.999999999999980016, -28.06379628232387446 ) ) ;
#29308=ORIENTED_EDGE ( 'NONE', *, *, #28285, .F. ) ;
#29309=VERTEX_POINT ( 'NONE', #22227 ) ;
#29310=DIRECTION ( 'NONE',  ( -1.110223024625156540E-16, 0.000000000000000000, -1.000000000000000000 ) ) ;
#29311=CARTESIAN_POINT ( 'NONE',  ( 177.2287565553228319, -9.999999999999994671, -3.509618943233403510 ) ) ;
#29312=DIRECTION ( 'NONE',  ( 0.5877852522924731371, 1.586114251531760728E-16, -0.8090169943749474513 ) ) ;
#29313=ORIENTED_EDGE ( 'NONE', *, *, #2717, .F. ) ;
#29316=AXIS2_PLACEMENT_3D ( 'NONE', #14101, #244, #552 ) ;
#29317=VECTOR ( 'NONE', #5574, 1000.000000000000000 ) ;
#29319=VECTOR ( 'NONE', #25848, 1000.000000000000000 ) ;
#29321=CARTESIAN_POINT ( 'NONE',  ( 139.5152310637605808, -1.999999999999979128, -2.627941064794695691 ) ) ;
#29322=DIRECTION ( 'NONE',  ( -0.8090169943749474513, -2.183098979609982436E-16, 0.5877852522924731371 ) ) ;
#29325=ADVANCED_FACE ( 'NONE', ( #12609 ), #29305, .T. ) ;
#29327=ORIENTED_EDGE ( 'NONE', *, *, #2382, .T. ) ;
#29330=PLANE ( 'NONE',  #5835 ) ;
#29333=CARTESIAN_POINT ( 'NONE',  ( 144.5152310637606092, -1.999999999999977129, -28.60870317832789311 ) ) ;
#29334=VECTOR ( 'NONE', #13524, 1000.000000000000000 ) ;
#29338=ORIENTED_EDGE ( 'NONE', *, *, #29040, .T. ) ;
#29339=VECTOR ( 'NONE', #16330, 1000.000000000000000 ) ;
#29344=FACE_BOUND ( 'NONE', #23976, .T. ) ;
#29345=ORIENTED_EDGE ( 'NONE', *, *, #3608, .T. ) ;
#29346=ORIENTED_EDGE ( 'NONE', *, *, #14477, .T. ) ;
#29347=( GEOMETRIC_REPRESENTATION_CONTEXT ( 3 ) GLOBAL_UNCERTAINTY_ASSIGNED_CONTEXT ( ( #18043 ) ) GLOBAL_UNIT_ASSIGNED_CONTEXT ( ( #29441, #15481, #10898 ) ) REPRESENTATION_CONTEXT ( 'NONE', 'WORKASPACE' ) );
#29348=ORIENTED_EDGE ( 'NONE', *, *, #957, .F. ) ;
#29349=DIRECTION ( 'NONE',  ( 1.000000000000000000, 2.698458740408365879E-16, 0.000000000000000000 ) ) ;
#29351=CARTESIAN_POINT ( 'NONE',  ( 151.1922820468854241, -10.00000000000000178, -19.40354224447947828 ) ) ;
#29353=DIRECTION ( 'NONE',  ( 1.000000000000000000, 2.698458740408365879E-16, -1.110223024625156540E-16 ) ) ;
#29354=ORIENTED_EDGE ( 'NONE', *, *, #21857, .T. ) ;
#29356=EDGE_LOOP ( 'NONE', ( #12073, #16221, #24914, #19596, #6551 ) ) ;
#29360=ORIENTED_EDGE ( 'NONE', *, *, #9581, .F. ) ;
#29362=AXIS2_PLACEMENT_3D ( 'NONE', #394, #20826, #23280 ) ;
#29363=ADVANCED_FACE ( 'NONE', ( #6059 ), #17339, .T. ) ;
#29364=AXIS2_PLACEMENT_3D ( 'NONE', #6177, #8747, #13335 ) ;
#29367=DIRECTION ( 'NONE',  ( 0.3090169943749475623, 8.338696094058001131E-17, 0.9510565162951536422 ) ) ;
#29368=FACE_BOUND ( 'NONE', #7413, .T. ) ;
#29370=ORIENTED_EDGE ( 'NONE', *, *, #10502, .T. ) ;
#29373=CARTESIAN_POINT ( 'NONE',  ( 174.7287565553228319, -4.999999999999969802, 0.8205080756888000204 ) ) ;
#29374=ORIENTED_EDGE ( 'NONE', *, *, #823, .F. ) ;
#29378=CARTESIAN_POINT ( 'NONE',  ( 174.5152310637604671, -9.999999999999994671, -30.37205893520531319 ) ) ;
#29379=EDGE_LOOP ( 'NONE', ( #16954, #18161, #14258, #10145 ) ) ;
#29380=VECTOR ( 'NONE', #27528, 1000.000000000000000 ) ;
#29382=ORIENTED_EDGE ( 'NONE', *, *, #12891, .F. ) ;
#29384=CARTESIAN_POINT ( 'NONE',  ( 138.6922820468854525, -10.00000000000000533, -15.07341522555727309 ) ) ;
#29385=CARTESIAN_POINT ( 'NONE',  ( 99.97015463715061401, -4.999999999999990230, 72.63256887516226357 ) ) ;
#29386=LINE ( 'NONE', #15732, #28660 ) ;
#29387=EDGE_LOOP ( 'NONE', ( #5143, #13956, #5768, #3980 ) ) ;
#29391=VERTEX_POINT ( 'NONE', #24682 ) ;
#29392=VERTEX_POINT ( 'NONE', #24081 ) ;
#29393=VERTEX_POINT ( 'NONE', #21624 ) ;
#29394=ORIENTED_EDGE ( 'NONE', *, *, #26709, .T. ) ;
#29396=AXIS2_PLACEMENT_3D ( 'NONE', #13902, #8723, #27546 ) ;
#29397=ORIENTED_EDGE ( 'NONE', *, *, #12031, .F. ) ;
#29398=CARTESIAN_POINT ( 'NONE',  ( 21.25294847316966695, -5.000000000000011546, -65.40984963230826565 ) ) ;
#29400=DIRECTION ( 'NONE',  ( 0.3090169943749475623, 8.338696094058001131E-17, 0.9510565162951536422 ) ) ;
#29403=EDGE_CURVE ( 'NONE', #4895, #4321, #3182, .T. ) ;
#29405=ORIENTED_EDGE ( 'NONE', *, *, #17446, .T. ) ;
#29406=VECTOR ( 'NONE', #27844, 1000.000000000000000 ) ;
#29407=ADVANCED_FACE ( 'NONE', ( #22083 ), #7739, .T. ) ;
#29408=VERTEX_POINT ( 'NONE', #19772 ) ;
#29409=VERTEX_POINT ( 'NONE', #15195 ) ;
#29410=PLANE ( 'NONE',  #4977 ) ;
#29411=DIRECTION ( 'NONE',  ( -0.5877852522924731371, 0.000000000000000000, 0.8090169943749474513 ) ) ;
#29413=CARTESIAN_POINT ( 'NONE',  ( 139.5152310637606092, -10.00000000000000533, -19.94844914048349338 ) ) ;
#29414=CARTESIAN_POINT ( 'NONE',  ( 147.0152310637605240, -1.999999999999977129, -8.721423840594312082 ) ) ;
#29416=DIRECTION ( 'NONE',  ( -1.110223024625156540E-16, 0.000000000000000000, -1.000000000000000000 ) ) ;
#29419=CARTESIAN_POINT ( 'NONE',  ( 151.1922820468853956, -10.00000000000000178, -10.74328820663507678 ) ) ;
#29420=VERTEX_POINT ( 'NONE', #5608 ) ;
#29422=FACE_OUTER_BOUND ( 'NONE', #21131, .T. ) ;
#29423=EDGE_LOOP ( 'NONE', ( #13161, #22003, #14019, #16531 ) ) ;
#29426=DIRECTION ( 'NONE',  ( 0.9510565162951536422, 0.000000000000000000, -0.3090169943749475623 ) ) ;
#29427=LINE ( 'NONE', #1151, #4872 ) ;
#29429=EDGE_LOOP ( 'NONE', ( #26503, #22862, #24249, #3725 ) ) ;
#29430=LINE ( 'NONE', #15468, #9053 ) ;
#29433=PLANE ( 'NONE',  #14665 ) ;
#29436=DIRECTION ( 'NONE',  ( -1.110223024625156540E-16, 0.000000000000000000, -1.000000000000000000 ) ) ;
#29439=CARTESIAN_POINT ( 'NONE',  ( 174.5152310637604671, -1.999999999999969358, -19.94844914048349693 ) ) ;
#29440=VERTEX_POINT ( 'NONE', #12454 ) ;
#29441=( LENGTH_UNIT ( ) NAMED_UNIT ( * ) SI_UNIT ( .MILLI., .METRE. ) );
#29443=VECTOR ( 'NONE', #9014, 1000.000000000000000 ) ;
#29445=EDGE_CURVE ( 'NONE', #25049, #18808, #24530, .T. ) ;
#29446=ADVANCED_FACE ( 'NONE', ( #880 ), #24370, .T. ) ;
#29448=EDGE_CURVE ( 'NONE', #22518, #4151, #22845, .T. ) ;
#29449=VERTEX_POINT ( 'NONE', #30060 ) ;
#29452=AXIS2_PLACEMENT_3D ( 'NONE', #114, #11251, #20553 ) ;
#29453=FACE_OUTER_BOUND ( 'NONE', #21370, .T. ) ;
#29454=ORIENTED_EDGE ( 'NONE', *, *, #13724, .T. ) ;
#29456=DIRECTION ( 'NONE',  ( -1.110223024625156540E-16, 0.000000000000000000, -1.000000000000000000 ) ) ;
#29457=CARTESIAN_POINT ( 'NONE',  ( 132.2287565553230024, -10.00000000000000888, -12.16987298107780013 ) ) ;
#29462=CARTESIAN_POINT ( 'NONE',  ( 130.7287565553229172, -4.999999999999983125, -33.50000000000000000 ) ) ;
#29464=LINE ( 'NONE', #1491, #13696 ) ;
#29465=CARTESIAN_POINT ( 'NONE',  ( 166.1922820468853104, -1.999999999999972244, -2.083034168790677043 ) ) ;
#29467=CARTESIAN_POINT ( 'NONE',  ( 130.7287565553229172, -9.999999999999982236, -33.50000000000000000 ) ) ;
#29468=VERTEX_POINT ( 'NONE', #22545 ) ;
#29469=CARTESIAN_POINT ( 'NONE',  ( 162.2287565553229456, -1.999999999999972244, -20.83012701892220520 ) ) ;
#29471=ADVANCED_FACE ( 'NONE', ( #11230 ), #6659, .T. ) ;
#29472=ORIENTED_EDGE ( 'NONE', *, *, #28880, .F. ) ;
#29473=DIRECTION ( 'NONE',  ( 1.110223024625156540E-16, 2.995891024602366092E-32, 1.000000000000000000 ) ) ;
#29475=CARTESIAN_POINT ( 'NONE',  ( 163.6922820468853104, -1.999999999999973133, -9.266330736598359152 ) ) ;
#29481=ADVANCED_FACE ( 'NONE', ( #25426 ), #25278, .T. ) ;
#29483=CARTESIAN_POINT ( 'NONE',  ( 14.09485158040538266, -5.000000000000014211, -43.37949266794227299 ) ) ;
#29484=DIRECTION ( 'NONE',  ( 0.9510565162951536422, 2.566386769018988816E-16, 0.3090169943749472292 ) ) ;
#29486=DIRECTION ( 'NONE',  ( 0.5877852522924731371, 1.586114251531760728E-16, 0.8090169943749474513 ) ) ;
#29487=EDGE_CURVE ( 'NONE', #24269, #5616, #4367, .T. ) ;
#29488=ORIENTED_EDGE ( 'NONE', *, *, #18366, .F. ) ;
#29489=ORIENTED_EDGE ( 'NONE', *, *, #17743, .T. ) ;
#29491=LINE ( 'NONE', #20253, #4378 ) ;
#29493=DIRECTION ( 'NONE',  ( 0.5877852522924731371, 1.586114251531760728E-16, -0.8090169943749474513 ) ) ;
#29498=ORIENTED_EDGE ( 'NONE', *, *, #1379, .T. ) ;
#29499=CARTESIAN_POINT ( 'NONE',  ( 21.65145737125105541, -5.000000000000011546, -66.63633390735121509 ) ) ;
#29501=FACE_BOUND ( 'NONE', #4161, .T. ) ;
#29502=EDGE_CURVE ( 'NONE', #619, #3067, #11080, .T. ) ;
#29503=VERTEX_POINT ( 'NONE', #6364 ) ;
#29504=LINE ( 'NONE', #25025, #10518 ) ;
#29505=ORIENTED_EDGE ( 'NONE', *, *, #22462, .F. ) ;
#29507=DIRECTION ( 'NONE',  ( -0.5877852522924731371, -1.586114251531760728E-16, -0.8090169943749474513 ) ) ;
#29508=CARTESIAN_POINT ( 'NONE',  ( 137.0152310637605808, -10.00000000000000533, -8.721423840594312082 ) ) ;
#29509=VERTEX_POINT ( 'NONE', #20677 ) ;
#29515=ORIENTED_EDGE ( 'NONE', *, *, #2565, .T. ) ;
#29516=LINE ( 'NONE', #6563, #10335 ) ;
#29517=EDGE_CURVE ( 'NONE', #5352, #20011, #9072, .T. ) ;
#29520=VECTOR ( 'NONE', #23131, 1000.000000000000000 ) ;
#29521=CARTESIAN_POINT ( 'NONE',  ( 146.1922820468854525, -4.999999999999978684, -22.25671179336496053 ) ) ;
#29523=VERTEX_POINT ( 'NONE', #22388 ) ;
#29526=CARTESIAN_POINT ( 'NONE',  ( 20.77549095910703869, -5.000000000000012434, -63.94038650157708759 ) ) ;
#29527=ORIENTED_EDGE ( 'NONE', *, *, #3402, .T. ) ;
#29528=ORIENTED_EDGE ( 'NONE', *, *, #16619, .F. ) ;
#29529=FACE_OUTER_BOUND ( 'NONE', #21354, .T. ) ;
#29535=CARTESIAN_POINT ( 'NONE',  ( 172.0152310637604103, -1.999999999999970468, -8.721423840594312082 ) ) ;
#29537=CARTESIAN_POINT ( 'NONE',  ( 15.52722412259326745, -5.000000000000013323, -47.78788206013580009 ) ) ;
#29539=EDGE_LOOP ( 'NONE', ( #24901, #11414, #24295, #16023 ) ) ;
#29546=ORIENTED_EDGE ( 'NONE', *, *, #16103, .F. ) ;
#29547=ORIENTED_EDGE ( 'NONE', *, *, #25839, .T. ) ;
#29548=ORIENTED_EDGE ( 'NONE', *, *, #25662, .T. ) ;
#29551=CARTESIAN_POINT ( 'NONE',  ( 174.7287565553229172, -1.999999999999968914, -25.16025403784440329 ) ) ;
#29556=ORIENTED_EDGE ( 'NONE', *, *, #5635, .T. ) ;
#29557=FACE_OUTER_BOUND ( 'NONE', #14918, .T. ) ;
#29558=FACE_OUTER_BOUND ( 'NONE', #252, .T. ) ;
#29559=DIRECTION ( 'NONE',  ( -2.698458740408365879E-16, 1.000000000000000000, 0.000000000000000000 ) ) ;
#29561=DIRECTION ( 'NONE',  ( -0.8090169943749474513, -2.183098979609982436E-16, 0.5877852522924731371 ) ) ;
#29562=DIRECTION ( 'NONE',  ( -2.698458740408365879E-16, 1.000000000000000000, 0.000000000000000000 ) ) ;
#29563=DIRECTION ( 'NONE',  ( -2.698458740408365879E-16, 1.000000000000000000, 0.000000000000000000 ) ) ;
#29567=EDGE_CURVE ( 'NONE', #7358, #23017, #13065, .T. ) ;
#29568=EDGE_CURVE ( 'NONE', #8986, #6652, #1494, .T. ) ;
#29569=DIRECTION ( 'NONE',  ( -2.698458740408365879E-16, 1.000000000000000000, 0.000000000000000000 ) ) ;
#29570=DIRECTION ( 'NONE',  ( -2.698458740408365879E-16, 1.000000000000000000, 0.000000000000000000 ) ) ;
#29571=VERTEX_POINT ( 'NONE', #29467 ) ;
#29574=AXIS2_PLACEMENT_3D ( 'NONE', #28917, #6120, #15568 ) ;
#29575=DIRECTION ( 'NONE',  ( -0.8090169943749474513, -2.183098979609982436E-16, -0.5877852522924731371 ) ) ;
#29577=CARTESIAN_POINT ( 'NONE',  ( 167.0152310637604387, -4.999999999999972466, -8.721423840594312082 ) ) ;
#29578=EDGE_CURVE ( 'NONE', #14185, #3020, #10923, .T. ) ;
#29580=ORIENTED_EDGE ( 'NONE', *, *, #17582, .T. ) ;
#29581=DIRECTION ( 'NONE',  ( 0.9510565162951536422, 2.566386769018988816E-16, 0.3090169943749472292 ) ) ;
#29583=FACE_OUTER_BOUND ( 'NONE', #8966, .T. ) ;
#29586=LINE ( 'NONE', #15475, #8629 ) ;
#29589=CARTESIAN_POINT ( 'NONE',  ( 91.42100672702999020, -4.999999999999992895, 66.42124934025146388 ) ) ;
#29590=ORIENTED_EDGE ( 'NONE', *, *, #19141, .F. ) ;
#29591=AXIS2_PLACEMENT_3D ( 'NONE', #4657, #27597, #20983 ) ;
#29598=EDGE_LOOP ( 'NONE', ( #23624, #20636, #25358, #11923 ) ) ;
#29600=VECTOR ( 'NONE', #3737, 1000.000000000000000 ) ;
#29602=CARTESIAN_POINT ( 'NONE',  ( 161.1922820468853104, -4.999999999999975131, -4.936203717676158398 ) ) ;
#29603=ORIENTED_EDGE ( 'NONE', *, *, #4777, .F. ) ;
#29604=CARTESIAN_POINT ( 'NONE',  ( 177.2287565553228887, -1.999999999999968470, -20.83012701892220520 ) ) ;
#29605=VECTOR ( 'NONE', #19282, 1000.000000000000000 ) ;
#29607=DIRECTION ( 'NONE',  ( 1.110223024625156540E-16, 2.995891024602366092E-32, 1.000000000000000000 ) ) ;
#29612=LINE ( 'NONE', #17637, #1748 ) ;
#29614=EDGE_CURVE ( 'NONE', #11825, #2371, #29620, .T. ) ;
#29615=AXIS2_PLACEMENT_3D ( 'NONE', #19905, #8156, #6176 ) ;
#29616=LINE ( 'NONE', #24679, #76 ) ;
#29617=PLANE ( 'NONE',  #15366 ) ;
#29618=ADVANCED_FACE ( 'NONE', ( #13516 ), #17935, .T. ) ;
#29620=LINE ( 'NONE', #1643, #11201 ) ;
#29621=CARTESIAN_POINT ( 'NONE',  ( 130.7287565553229172, -9.999999999999982236, -36.50000000000000711 ) ) ;
#29623=ORIENTED_EDGE ( 'NONE', *, *, #28801, .T. ) ;
#29624=VECTOR ( 'NONE', #24157, 1000.000000000000000 ) ;
#29626=CARTESIAN_POINT ( 'NONE',  ( 22.12891488531368367, -5.000000000000011546, -68.10579703808238605 ) ) ;
#29629=ORIENTED_EDGE ( 'NONE', *, *, #19686, .F. ) ;
#29634=DIRECTION ( 'NONE',  ( -0.5877852522924731371, -1.586114251531760728E-16, -0.8090169943749474513 ) ) ;
#29635=LINE ( 'NONE', #27329, #12797 ) ;
#29637=VECTOR ( 'NONE', #13157, 1000.000000000000000 ) ;
#29638=ORIENTED_EDGE ( 'NONE', *, *, #6474, .T. ) ;
#29639=DIRECTION ( 'NONE',  ( -0.8090169943749474513, -2.183098979609982436E-16, -0.5877852522924731371 ) ) ;
#29640=LINE ( 'NONE', #6388, #29280 ) ;
#29641=VECTOR ( 'NONE', #6552, 1000.000000000000000 ) ;
#29643=CARTESIAN_POINT ( 'NONE',  ( 131.1922820468854241, -1.999999999999981792, -19.40354224447947473 ) ) ;
#29644=LINE ( 'NONE', #13976, #8759 ) ;
#29646=VERTEX_POINT ( 'NONE', #2686 ) ;
#29648=EDGE_LOOP ( 'NONE', ( #1773, #20909, #3034, #26164, #10509 ) ) ;
#29649=EDGE_CURVE ( 'NONE', #8074, #20055, #26039, .T. ) ;
#29652=EDGE_CURVE ( 'NONE', #25166, #9388, #16065, .T. ) ;
#29654=FACE_OUTER_BOUND ( 'NONE', #21532, .T. ) ;
#29655=EDGE_CURVE ( 'NONE', #1559, #7167, #12534, .T. ) ;
#29656=VERTEX_POINT ( 'NONE', #10093 ) ;
#29657=LINE ( 'NONE', #15234, #21237 ) ;
#29658=VECTOR ( 'NONE', #27420, 1000.000000000000000 ) ;
#29660=LINE ( 'NONE', #10818, #2339 ) ;
#29661=PLANE ( 'NONE',  #27175 ) ;
#29664=VECTOR ( 'NONE', #22965, 1000.000000000000000 ) ;
#29668=DIRECTION ( 'NONE',  ( -0.9510565162951536422, -2.566386769018988323E-16, 0.3090169943749475623 ) ) ;
#29669=CARTESIAN_POINT ( 'NONE',  ( 174.5152310637604387, -1.999999999999969580, -11.28819510263909542 ) ) ;
#29670=VECTOR ( 'NONE', #6005, 1000.000000000000000 ) ;
#29672=VERTEX_POINT ( 'NONE', #24302 ) ;
#29673=LINE ( 'NONE', #24894, #336 ) ;
#29674=DIRECTION ( 'NONE',  ( -0.8090169943749474513, -2.183098979609982436E-16, 0.5877852522924731371 ) ) ;
#29676=ORIENTED_EDGE ( 'NONE', *, *, #3406, .F. ) ;
#29681=ORIENTED_EDGE ( 'NONE', *, *, #23879, .F. ) ;
#29682=ORIENTED_EDGE ( 'NONE', *, *, #27554, .F. ) ;
#29683=CARTESIAN_POINT ( 'NONE',  ( 132.0152310637605808, -4.999999999999982236, 1.702185954127501066 ) ) ;
#29688=VECTOR ( 'NONE', #14954, 1000.000000000000000 ) ;
#29689=VERTEX_POINT ( 'NONE', #7669 ) ;
#29692=PLANE ( 'NONE',  #12221 ) ;
#29693=CARTESIAN_POINT ( 'NONE',  ( 159.5152310637604387, -10.00000000000000000, -4.391296821672111328 ) ) ;
#29695=LINE ( 'NONE', #18024, #12022 ) ;
#29696=VERTEX_POINT ( 'NONE', #3114 ) ;
#29700=ORIENTED_EDGE ( 'NONE', *, *, #8754, .T. ) ;
#29701=VECTOR ( 'NONE', #17774, 1000.000000000000000 ) ;
#29702=PLANE ( 'NONE',  #29182 ) ;
#29703=DIRECTION ( 'NONE',  ( 1.110223024625156540E-16, 2.995891024602366092E-32, 1.000000000000000000 ) ) ;
#29709=ORIENTED_EDGE ( 'NONE', *, *, #2896, .F. ) ;
#29710=VERTEX_POINT ( 'NONE', #12387 ) ;
#29711=EDGE_CURVE ( 'NONE', #7341, #11438, #3396, .T. ) ;
#29712=DIRECTION ( 'NONE',  ( 0.000000000000000000, 0.000000000000000000, -1.000000000000000000 ) ) ;
#29713=VECTOR ( 'NONE', #21051, 1000.000000000000000 ) ;
#29715=CARTESIAN_POINT ( 'NONE',  ( 168.6922820468853104, -4.999999999999972466, -6.413161187712876909 ) ) ;
#29718=VECTOR ( 'NONE', #21363, 1000.000000000000000 ) ;
#29722=DIRECTION ( 'NONE',  ( -2.698458740408365879E-16, 1.000000000000000000, 0.000000000000000000 ) ) ;
#29723=VERTEX_POINT ( 'NONE', #26153 ) ;
#29724=LINE ( 'NONE', #6317, #27630 ) ;
#29725=VECTOR ( 'NONE', #13027, 1000.000000000000000 ) ;
#29727=ORIENTED_EDGE ( 'NONE', *, *, #24466, .F. ) ;
#29729=LINE ( 'NONE', #18927, #12085 ) ;
#29731=DIRECTION ( 'NONE',  ( -1.779203565104417375E-16, -4.801107411221739977E-32, -1.000000000000000000 ) ) ;
#29732=LINE ( 'NONE', #1907, #2072 ) ;
#29734=VERTEX_POINT ( 'NONE', #10244 ) ;
#29735=AXIS2_PLACEMENT_3D ( 'NONE', #17214, #14602, #14756 ) ;
#29736=EDGE_LOOP ( 'NONE', ( #17274, #17502, #1872, #7065 ) ) ;
#29739=AXIS2_PLACEMENT_3D ( 'NONE', #6802, #20522, #16091 ) ;
#29741=DIRECTION ( 'NONE',  ( 0.9510565162951536422, 0.000000000000000000, -0.3090169943749475623 ) ) ;
#29743=CARTESIAN_POINT ( 'NONE',  ( 142.0152310637605240, -10.00000000000000533, -0.06116980274991495881 ) ) ;
#29745=ORIENTED_EDGE ( 'NONE', *, *, #10485, .T. ) ;
#29746=FACE_OUTER_BOUND ( 'NONE', #1112, .T. ) ;
#29747=( LENGTH_UNIT ( ) NAMED_UNIT ( * ) SI_UNIT ( .MILLI., .METRE. ) );
#29750=ORIENTED_EDGE ( 'NONE', *, *, #21721, .T. ) ;
#29751=EDGE_CURVE ( 'NONE', #30179, #9897, #26301, .T. ) ;
#29753=FACE_OUTER_BOUND ( 'NONE', #1472, .T. ) ;
#29754=ADVANCED_FACE ( 'NONE', ( #14671 ), #9801, .T. ) ;
#29755=PLANE ( 'NONE',  #28492 ) ;
#29756=AXIS2_PLACEMENT_3D ( 'NONE', #1361, #26398, #10649 ) ;
#29757=EDGE_LOOP ( 'NONE', ( #19553, #13981, #20299, #23094 ) ) ;
#29758=DIRECTION ( 'NONE',  ( -0.9510565162951536422, -2.566386769018988816E-16, -0.3090169943749472292 ) ) ;
#29759=CARTESIAN_POINT ( 'NONE',  ( 133.7287565553229172, -9.999999999999982236, -36.50000000000000711 ) ) ;
#29761=DIRECTION ( 'NONE',  ( -2.698458740408365879E-16, 1.000000000000000000, 0.000000000000000000 ) ) ;
#29767=FACE_OUTER_BOUND ( 'NONE', #18261, .T. ) ;
#29770=CARTESIAN_POINT ( 'NONE',  ( 147.0152310637605240, -10.00000000000000178, -8.721423840594312082 ) ) ;
#29771=VERTEX_POINT ( 'NONE', #21699 ) ;
#29774=VERTEX_POINT ( 'NONE', #19115 ) ;
#29776=LINE ( 'NONE', #6516, #3248 ) ;
#29777=LINE ( 'NONE', #25284, #9792 ) ;
#29778=DIRECTION ( 'NONE',  ( -1.110223024625156540E-16, 0.000000000000000000, -1.000000000000000000 ) ) ;
#29779=AXIS2_PLACEMENT_3D ( 'NONE', #2705, #21153, #572 ) ;
#29780=VERTEX_POINT ( 'NONE', #5228 ) ;
#29785=CARTESIAN_POINT ( 'NONE',  ( 158.6922820468853104, -10.00000000000000000, -0.6060766987539614181 ) ) ;
#29786=DIRECTION ( 'NONE',  ( -0.5877852522924731371, -1.586114251531760728E-16, -0.8090169943749474513 ) ) ;
#29788=ADVANCED_FACE ( 'NONE', ( #28927 ), #2963, .T. ) ;
#29789=ADVANCED_FACE ( 'NONE', ( #28470 ), #21559, .T. ) ;
#29790=EDGE_LOOP ( 'NONE', ( #8665, #15614, #29037, #14933, #18002 ) ) ;
#29791=ADVANCED_FACE ( 'NONE', ( #17127 ), #22012, .T. ) ;
#29792=DIRECTION ( 'NONE',  ( 0.9510565162951536422, 2.566386769018988816E-16, 0.3090169943749472292 ) ) ;
#29793=ORIENTED_EDGE ( 'NONE', *, *, #9796, .F. ) ;
#29794=PLANE ( 'NONE',  #24287 ) ;
#29795=VECTOR ( 'NONE', #5342, 1000.000000000000000 ) ;
#29797=ORIENTED_EDGE ( 'NONE', *, *, #27005, .F. ) ;
#29799=DIRECTION ( 'NONE',  ( -0.5877852522924731371, 0.000000000000000000, 0.8090169943749474513 ) ) ;
#29801=AXIS2_PLACEMENT_3D ( 'NONE', #13051, #10767, #22375 ) ;
#29802=CARTESIAN_POINT ( 'NONE',  ( 133.7287565553229740, -84.33034373659253902, 8.500000000000007105 ) ) ;
#29804=EDGE_LOOP ( 'NONE', ( #6218, #25668, #22918, #4919, #4108 ) ) ;
#29806=ORIENTED_EDGE ( 'NONE', *, *, #20685, .T. ) ;
#29811=ORIENTED_EDGE ( 'NONE', *, *, #18976, .F. ) ;
#29812=VECTOR ( 'NONE', #23903, 1000.000000000000000 ) ;
#29813=DIRECTION ( 'NONE',  ( -0.9510565162951536422, -2.566386769018988816E-16, -0.3090169943749472292 ) ) ;
#29814=CARTESIAN_POINT ( 'NONE',  ( 152.0152310637605808, -10.00000000000000000, -24.27857615940569502 ) ) ;
#29815=CARTESIAN_POINT ( 'NONE',  ( 173.6922820468853104, -4.999999999999970690, -15.07341522555727664 ) ) ;
#29824=ORIENTED_EDGE ( 'NONE', *, *, #16549, .T. ) ;
#29827=CARTESIAN_POINT ( 'NONE',  ( 133.7287565553229172, -4.999999999999982236, -33.50000000000000000 ) ) ;
#29829=EDGE_CURVE ( 'NONE', #9909, #3561, #962, .T. ) ;
#29830=EDGE_CURVE ( 'NONE', #23305, #25136, #7806, .T. ) ;
#29831=EDGE_CURVE ( 'NONE', #17674, #30043, #28612, .T. ) ;
#29833=ADVANCED_FACE ( 'NONE', ( #6877 ), #11574, .T. ) ;
#29834=AXIS2_PLACEMENT_3D ( 'NONE', #6373, #16113, #8494 ) ;
#29835=PLANE ( 'NONE',  #4523 ) ;
#29836=VECTOR ( 'NONE', #2168, 1000.000000000000000 ) ;
#29837=EDGE_LOOP ( 'NONE', ( #26958, #673, #29590, #21212 ) ) ;
#29839=CARTESIAN_POINT ( 'NONE',  ( 167.2287565553228887, -1.999999999999971800, -3.509618943233403510 ) ) ;
#29841=ORIENTED_EDGE ( 'NONE', *, *, #3068, .F. ) ;
#29842=CARTESIAN_POINT ( 'NONE',  ( 172.0152310637603819, -4.999999999999970690, -1.909752701132032347E-14 ) ) ;
#29846=ORIENTED_EDGE ( 'NONE', *, *, #17440, .F. ) ;
#29847=CARTESIAN_POINT ( 'NONE',  ( 172.0152310637604103, -9.999999999999996447, 1.702185954127501066 ) ) ;
#29849=LINE ( 'NONE', #11303, #29339 ) ;
#29851=EDGE_LOOP ( 'NONE', ( #21661, #11181, #15080, #23310 ) ) ;
#29852=CARTESIAN_POINT ( 'NONE',  ( 95.60450572449933304, -4.999999999999991118, -69.46073927778073198 ) ) ;
#29856=VECTOR ( 'NONE', #19918, 1000.000000000000000 ) ;
#29858=FACE_OUTER_BOUND ( 'NONE', #9073, .T. ) ;
#29864=EDGE_CURVE ( 'NONE', #21320, #15396, #16166, .T. ) ;
#29865=ADVANCED_FACE ( 'NONE', ( #12032 ), #28264, .T. ) ;
#29866=EDGE_CURVE ( 'NONE', #21590, #25250, #152, .T. ) ;
#29868=LINE ( 'NONE', #11612, #10810 ) ;
#29869=VECTOR ( 'NONE', #2092, 1000.000000000000000 ) ;
#29871=LINE ( 'NONE', #13459, #11160 ) ;
#29872=VECTOR ( 'NONE', #2284, 1000.000000000000000 ) ;
#29873=CARTESIAN_POINT ( 'NONE',  ( 169.7287565553229456, -9.999999999999996447, -25.16025403784440329 ) ) ;
#29875=LINE ( 'NONE', #20487, #24372 ) ;
#29876=EDGE_LOOP ( 'NONE', ( #9550, #12844, #696, #9152 ) ) ;
#29877=FACE_OUTER_BOUND ( 'NONE', #15912, .T. ) ;
#29878=ORIENTED_EDGE ( 'NONE', *, *, #28278, .F. ) ;
#29881=CARTESIAN_POINT ( 'NONE',  ( 163.6922820468853956, -1.999999999999972689, -32.39392330124607611 ) ) ;
#29882=FACE_OUTER_BOUND ( 'NONE', #29084, .T. ) ;
#29884=VERTEX_POINT ( 'NONE', #23646 ) ;
#29885=ORIENTED_EDGE ( 'NONE', *, *, #26528, .T. ) ;
#29886=DIRECTION ( 'NONE',  ( 0.5877852522924731371, 1.586114251531760728E-16, 0.8090169943749474513 ) ) ;
#29888=EDGE_CURVE ( 'NONE', #7982, #18285, #2746, .T. ) ;
#29890=DIRECTION ( 'NONE',  ( 0.3090169943749475623, 8.338696094058001131E-17, 0.9510565162951536422 ) ) ;
#29894=ORIENTED_EDGE ( 'NONE', *, *, #6123, .F. ) ;
#29895=DIRECTION ( 'NONE',  ( 0.3090169943749472292, 8.338696094057992503E-17, -0.9510565162951536422 ) ) ;
#29896=FILL_AREA_STYLE_COLOUR ( '', #9290 ) ;
#29899=EDGE_LOOP ( 'NONE', ( #9700, #7176, #10274, #628 ) ) ;
#29900=ORIENTED_EDGE ( 'NONE', *, *, #11030, .F. ) ;
#29901=LINE ( 'NONE', #23117, #23414 ) ;
#29903=ORIENTED_EDGE ( 'NONE', *, *, #28694, .F. ) ;
#29905=CARTESIAN_POINT ( 'NONE',  ( 173.6922820468852535, -9.999999999999996447, -0.6060766987539614181 ) ) ;
#29906=CARTESIAN_POINT ( 'NONE',  ( 163.6922820468853388, -1.999999999999972689, -15.07341522555727664 ) ) ;
#29908=AXIS2_PLACEMENT_3D ( 'NONE', #24169, #24316, #3411 ) ;
#29909=LINE ( 'NONE', #27589, #24802 ) ;
#29913=CARTESIAN_POINT ( 'NONE',  ( 141.1922820468854525, -4.999999999999980460, -30.91696583120935671 ) ) ;
#29915=DIRECTION ( 'NONE',  ( 0.5877852522924731371, 1.586114251531760728E-16, 0.8090169943749474513 ) ) ;
#29916=DIRECTION ( 'NONE',  ( -1.110223024625156540E-16, 0.000000000000000000, -1.000000000000000000 ) ) ;
#29918=CARTESIAN_POINT ( 'NONE',  ( 146.1922820468854525, -10.00000000000000178, -28.06379628232387446 ) ) ;
#29920=VERTEX_POINT ( 'NONE', #5019 ) ;
#29921=FACE_OUTER_BOUND ( 'NONE', #11208, .T. ) ;
#29925=LINE ( 'NONE', #20537, #12475 ) ;
#29926=CARTESIAN_POINT ( 'NONE',  ( 96.27478563531609268, -4.999999999999991118, 69.94772613865674771 ) ) ;
#29928=AXIS2_PLACEMENT_3D ( 'NONE', #28261, #28411, #14005 ) ;
#29930=ORIENTED_EDGE ( 'NONE', *, *, #22279, .F. ) ;
#29935=VECTOR ( 'NONE', #26473, 1000.000000000000000 ) ;
#29939=CARTESIAN_POINT ( 'NONE',  ( 136.1922820468854241, -10.00000000000000533, -4.936203717676158398 ) ) ;
#29941=DIRECTION ( 'NONE',  ( -0.8090169943749474513, -2.183098979609982436E-16, 0.5877852522924731371 ) ) ;
#29942=DIRECTION ( 'NONE',  ( 0.5877852522924731371, 0.000000000000000000, 0.8090169943749474513 ) ) ;
#29943=ORIENTED_EDGE ( 'NONE', *, *, #11317, .T. ) ;
#29946=VERTEX_POINT ( 'NONE', #7467 ) ;
#29947=AXIS2_PLACEMENT_3D ( 'NONE', #19617, #417, #8018 ) ;
#29951=LINE ( 'NONE', #8819, #20931 ) ;
#29952=CARTESIAN_POINT ( 'NONE',  ( 167.0152310637605240, -9.999999999999996447, -24.27857615940569502 ) ) ;
#29953=EDGE_CURVE ( 'NONE', #29309, #6553, #14466, .T. ) ;
#29954=EDGE_CURVE ( 'NONE', #9641, #27224, #26095, .T. ) ;
#29955=EDGE_LOOP ( 'NONE', ( #9224, #22716, #21861, #10239, #14434 ) ) ;
#29956=LINE ( 'NONE', #13843, #12941 ) ;
#29959=LINE ( 'NONE', #6549, #29872 ) ;
#29960=EDGE_LOOP ( 'NONE', ( #22470, #15370, #5543, #17888, #22 ) ) ;
#29969=PLANE ( 'NONE',  #17632 ) ;
#29971=VERTEX_POINT ( 'NONE', #25939 ) ;
#29972=AXIS2_PLACEMENT_3D ( 'NONE', #13939, #13499, #2226 ) ;
#29973=CARTESIAN_POINT ( 'NONE',  ( 168.6922820468853104, -9.999999999999998224, -6.413161187712876909 ) ) ;
#29974=CARTESIAN_POINT ( 'NONE',  ( 106.6906127300029112, -4.999999999999988454, -77.51526748729723693 ) ) ;
#29975=ADVANCED_FACE ( 'NONE', ( #11876 ), #12182, .T. ) ;
#29978=CARTESIAN_POINT ( 'NONE',  ( 130.7287565553229456, -4.999999999999983125, -4.785595155761468433 ) ) ;
#29981=LINE ( 'NONE', #27378, #6113 ) ;
#29985=VERTEX_POINT ( 'NONE', #9891 ) ;
#29988=EDGE_CURVE ( 'NONE', #25448, #17086, #7316, .T. ) ;
#29989=VECTOR ( 'NONE', #14762, 1000.000000000000000 ) ;
#29991=CARTESIAN_POINT ( 'NONE',  ( 132.0152310637605524, -1.999999999999981348, -8.721423840594310306 ) ) ;
#29992=CARTESIAN_POINT ( 'NONE',  ( 172.7287565553229456, -9.999999999999971578, 0.5000000000000029976 ) ) ;
#29993=EDGE_CURVE ( 'NONE', #6774, #11681, #21501, .T. ) ;
#29994=ADVANCED_FACE ( 'NONE', ( #23340 ), #28558, .T. ) ;
#29995=VERTEX_POINT ( 'NONE', #3351 ) ;
#29996=CARTESIAN_POINT ( 'NONE',  ( 168.6922820468853104, -1.999999999999971800, -9.266330736598359152 ) ) ;
#29997=EDGE_CURVE ( 'NONE', #6014, #4559, #19803, .T. ) ;
#29998=ORIENTED_EDGE ( 'NONE', *, *, #20579, .T. ) ;
#30002=DIRECTION ( 'NONE',  ( -2.698458740408365879E-16, 1.000000000000000000, 0.000000000000000000 ) ) ;
#30010=CARTESIAN_POINT ( 'NONE',  ( 168.6922820468853104, -1.999999999999971356, -6.413161187712876909 ) ) ;
#30011=CARTESIAN_POINT ( 'NONE',  ( 137.0152310637606092, -1.999999999999979572, -15.61832212156129351 ) ) ;
#30014=CARTESIAN_POINT ( 'NONE',  ( 167.0152310637605524, -1.999999999999970468, -32.93883019725009120 ) ) ;
#30015=ORIENTED_EDGE ( 'NONE', *, *, #23954, .F. ) ;
#30016=DIRECTION ( 'NONE',  ( 1.000000000000000000, 2.698458740408365879E-16, -1.110223024625156540E-16 ) ) ;
#30019=ADVANCED_FACE ( 'NONE', ( #3054 ), #7611, .T. ) ;
#30020=EDGE_CURVE ( 'NONE', #21693, #23660, #7912, .T. ) ;
#30027=VERTEX_POINT ( 'NONE', #29164 ) ;
#30028=CARTESIAN_POINT ( 'NONE',  ( 172.0152310637604671, -4.999999999999970690, -1.909752701132033294E-14 ) ) ;
#30029=EDGE_CURVE ( 'NONE', #20364, #24609, #3642, .T. ) ;
#30034=ORIENTED_EDGE ( 'NONE', *, *, #2491, .F. ) ;
#30035=VECTOR ( 'NONE', #26029, 1000.000000000000000 ) ;
#30036=PLANE ( 'NONE',  #25227 ) ;
#30039=CARTESIAN_POINT ( 'NONE',  ( 149.7287565553230024, -10.00000000000000178, -16.50000000000000355 ) ) ;
#30043=VERTEX_POINT ( 'NONE', #17515 ) ;
#30044=VECTOR ( 'NONE', #5453, 1000.000000000000000 ) ;
#30045=DIRECTION ( 'NONE',  ( 0.5877852522924731371, 1.586114251531760728E-16, 0.8090169943749474513 ) ) ;
#30046=CARTESIAN_POINT ( 'NONE',  ( 162.0152310637604103, -4.999999999999974243, -0.06116980274991495881 ) ) ;
#30048=DIRECTION ( 'NONE',  ( -0.9510565162951536422, -2.566386769018988323E-16, 0.3090169943749475623 ) ) ;
#30049=DIRECTION ( 'NONE',  ( 0.9510565162951536422, 2.566386769018988816E-16, 0.3090169943749472292 ) ) ;
#30052=CARTESIAN_POINT ( 'NONE',  ( 139.7287565553230309, -1.999999999999978684, -7.839745962155603820 ) ) ;
#30057=DIRECTION ( 'NONE',  ( 0.5877852522924731371, 1.586114251531760728E-16, 0.8090169943749474513 ) ) ;
#30058=LINE ( 'NONE', #1789, #25149 ) ;
#30060=CARTESIAN_POINT ( 'NONE',  ( 159.5152310637604671, -4.999999999999974243, -13.05155085951651195 ) ) ;
#30061=ORIENTED_EDGE ( 'NONE', *, *, #8833, .T. ) ;
#30065=VECTOR ( 'NONE', #15040, 1000.000000000000000 ) ;
#30066=ORIENTED_EDGE ( 'NONE', *, *, #27896, .F. ) ;
#30067=DIRECTION ( 'NONE',  ( -0.5877852522924731371, -1.586114251531760235E-16, 0.8090169943749474513 ) ) ;
#30068=CARTESIAN_POINT ( 'NONE',  ( 131.1922820468854241, -1.999999999999982236, -22.25671179336495697 ) ) ;
#30069=AXIS2_PLACEMENT_3D ( 'NONE', #17497, #3475, #15350 ) ;
#30071=ORIENTED_EDGE ( 'NONE', *, *, #23918, .F. ) ;
#30076=VECTOR ( 'NONE', #9871, 1000.000000000000000 ) ;
#30078=VECTOR ( 'NONE', #4806, 999.9999999999998863 ) ;
#30079=FACE_OUTER_BOUND ( 'NONE', #10976, .T. ) ;
#30081=VECTOR ( 'NONE', #18992, 1000.000000000000000 ) ;
#30083=DIRECTION ( 'NONE',  ( 0.3090169943749475623, 8.338696094058001131E-17, 0.9510565162951536422 ) ) ;
#30084=EDGE_CURVE ( 'NONE', #24609, #13066, #24254, .T. ) ;
#30085=LINE ( 'NONE', #15822, #13616 ) ;
#30087=VERTEX_POINT ( 'NONE', #22104 ) ;
#30088=CARTESIAN_POINT ( 'NONE',  ( 143.6922820468854525, -10.00000000000000355, -23.73366926340167282 ) ) ;
#30089=AXIS2_PLACEMENT_3D ( 'NONE', #15015, #22055, #17461 ) ;
#30096=CARTESIAN_POINT ( 'NONE',  ( 161.1922820468853388, -4.999999999999974243, -10.74328820663507678 ) ) ;
#30098=CARTESIAN_POINT ( 'NONE',  ( 176.1922820468853104, -9.999999999999994671, -22.25671179336496053 ) ) ;
#30099=DIRECTION ( 'NONE',  ( -0.5877852522924731371, 0.000000000000000000, 0.8090169943749474513 ) ) ;
#30100=ORIENTED_EDGE ( 'NONE', *, *, #10605, .T. ) ;
#30101=VERTEX_POINT ( 'NONE', #26400 ) ;
#30105=CARTESIAN_POINT ( 'NONE',  ( 169.5152310637604387, -9.999999999999996447, -13.05155085951651195 ) ) ;
#30106=VERTEX_POINT ( 'NONE', #26710 ) ;
#30110=ORIENTED_EDGE ( 'NONE', *, *, #22315, .F. ) ;
#30115=VERTEX_POINT ( 'NONE', #1210 ) ;
#30116=VECTOR ( 'NONE', #16679, 1000.000000000000000 ) ;
#30118=AXIS2_PLACEMENT_3D ( 'NONE', #15710, #25039, #8237 ) ;
#30119=( NAMED_UNIT ( * ) SI_UNIT ( $, .STERADIAN. ) SOLID_ANGLE_UNIT ( ) );
#30120=ADVANCED_FACE ( 'NONE', ( #26245 ), #26549, .T. ) ;
#30122=EDGE_CURVE ( 'NONE', #2975, #12094, #29017, .T. ) ;
#30123=DIRECTION ( 'NONE',  ( 1.110223024625156540E-16, 2.995891024602366092E-32, 1.000000000000000000 ) ) ;
#30124=EDGE_CURVE ( 'NONE', #1065, #14964, #19202, .T. ) ;
#30125=EDGE_CURVE ( 'NONE', #23706, #5568, #741, .T. ) ;
#30128=DIRECTION ( 'NONE',  ( 0.9510565162951535312, 2.566386769018988816E-16, -0.3090169943749475623 ) ) ;
#30131=CARTESIAN_POINT ( 'NONE',  ( 6.464122205792598663, -5.000000000000015987, 19.89452249505685799 ) ) ;
#30132=VECTOR ( 'NONE', #18812, 1000.000000000000000 ) ;
#30136=ORIENTED_EDGE ( 'NONE', *, *, #1515, .T. ) ;
#30137=ORIENTED_EDGE ( 'NONE', *, *, #11412, .T. ) ;
#30138=VECTOR ( 'NONE', #7781, 1000.000000000000000 ) ;
#30141=LINE ( 'NONE', #11749, #19040 ) ;
#30143=ORIENTED_EDGE ( 'NONE', *, *, #15891, .T. ) ;
#30144=CARTESIAN_POINT ( 'NONE',  ( 157.0152310637604671, -10.00000000000000000, -8.721423840594312082 ) ) ;
#30145=ORIENTED_EDGE ( 'NONE', *, *, #7201, .T. ) ;
#30149=ORIENTED_EDGE ( 'NONE', *, *, #295, .F. ) ;
#30150=ORIENTED_EDGE ( 'NONE', *, *, #15650, .T. ) ;
#30151=CARTESIAN_POINT ( 'NONE',  ( 141.1922820468854525, -1.999999999999978462, -28.06379628232387446 ) ) ;
#30156=VECTOR ( 'NONE', #2961, 1000.000000000000000 ) ;
#30157=ORIENTED_EDGE ( 'NONE', *, *, #12445, .T. ) ;
#30158=ORIENTED_EDGE ( 'NONE', *, *, #27098, .F. ) ;
#30159=LINE ( 'NONE', #15745, #26950 ) ;
#30160=ADVANCED_FACE ( 'NONE', ( #5479 ), #14761, .T. ) ;
#30161=VECTOR ( 'NONE', #13042, 1000.000000000000000 ) ;
#30162=ADVANCED_FACE ( 'NONE', ( #902 ), #20255, .T. ) ;
#30163=EDGE_CURVE ( 'NONE', #21141, #28787, #15372, .T. ) ;
#30166=CARTESIAN_POINT ( 'NONE',  ( 143.6922820468854525, -10.00000000000000355, -35.24709285013155835 ) ) ;
#30167=LINE ( 'NONE', #47, #17776 ) ;
#30169=LINE ( 'NONE', #9330, #18017 ) ;
#30170=ORIENTED_EDGE ( 'NONE', *, *, #7321, .F. ) ;
#30171=CARTESIAN_POINT ( 'NONE',  ( 153.6922820468853388, -4.999999999999976019, -0.6060766987539614181 ) ) ;
#30172=ORIENTED_EDGE ( 'NONE', *, *, #13009, .T. ) ;
#30174=ORIENTED_EDGE ( 'NONE', *, *, #9367, .F. ) ;
#30177=DIRECTION ( 'NONE',  ( -0.5877852522924731371, -1.586114251531760728E-16, -0.8090169943749474513 ) ) ;
#30178=CARTESIAN_POINT ( 'NONE',  ( 174.5152310637604103, -1.999999999999970024, -2.627941064794695691 ) ) ;
#30179=VERTEX_POINT ( 'NONE', #24861 ) ;
#30180=EDGE_LOOP ( 'NONE', ( #12575, #26278, #9250, #29252 ) ) ;
#30181=DIRECTION ( 'NONE',  ( 0.000000000000000000, -1.000000000000000000, 0.000000000000000000 ) ) ;
#30183=AXIS2_PLACEMENT_3D ( 'NONE', #2486, #13893, #11906 ) ;
#30186=FACE_OUTER_BOUND ( 'NONE', #9755, .T. ) ;
#30190=EDGE_CURVE ( 'NONE', #1623, #13813, #4799, .T. ) ;
#30193=VERTEX_POINT ( 'NONE', #22412 ) ;
#30194=EDGE_CURVE ( 'NONE', #11751, #16627, #8656, .T. ) ;
#30195=VECTOR ( 'NONE', #19242, 1000.000000000000000 ) ;
#30196=EDGE_CURVE ( 'NONE', #9083, #9595, #15824, .T. ) ;
#30197=DIRECTION ( 'NONE',  ( -2.698458740408365879E-16, 1.000000000000000000, 0.000000000000000000 ) ) ;
#30198=ADVANCED_FACE ( 'NONE', ( #15679 ), #10949, .T. ) ;
#30200=VECTOR ( 'NONE', #1389, 1000.000000000000000 ) ;
#30201=DIRECTION ( 'NONE',  ( -0.5877852522924731371, 0.000000000000000000, 0.8090169943749474513 ) ) ;
#30207=VECTOR ( 'NONE', #23649, 1000.000000000000000 ) ;
#30208=CARTESIAN_POINT ( 'NONE',  ( 153.6922820468853388, -4.999999999999976019, -15.07341522555727309 ) ) ;
#30209=CARTESIAN_POINT ( 'NONE',  ( 144.7287565553230309, -10.00000000000000355, -16.50000000000000355 ) ) ;
#30210=DIRECTION ( 'NONE',  ( -0.5877852522924731371, 0.000000000000000000, 0.8090169943749474513 ) ) ;
#30212=ORIENTED_EDGE ( 'NONE', *, *, #9472, .T. ) ;
#30213=PLANE ( 'NONE',  #19778 ) ;
#30216=DIRECTION ( 'NONE',  ( -0.5877852522924731371, -1.586114251531760728E-16, -0.8090169943749474513 ) ) ;
#30217=LINE ( 'NONE', #25570, #23964 ) ;
#30219=ORIENTED_EDGE ( 'NONE', *, *, #8836, .T. ) ;
#30221=ORIENTED_EDGE ( 'NONE', *, *, #22240, .F. ) ;
#30222=EDGE_CURVE ( 'NONE', #19874, #8637, #13088, .T. ) ;
#30229=VECTOR ( 'NONE', #22217, 1000.000000000000000 ) ;
#30230=ADVANCED_FACE ( 'NONE', ( #25011 ), #7093, .T. ) ;
#30231=EDGE_LOOP ( 'NONE', ( #1476, #24888, #24420, #12313, #26829 ) ) ;
#30233=PLANE ( 'NONE',  #26982 ) ;
#30234=EDGE_CURVE ( 'NONE', #15731, #26001, #25715, .T. ) ;
#30236=ORIENTED_EDGE ( 'NONE', *, *, #10564, .F. ) ;
#30238=LINE ( 'NONE', #23020, #25836 ) ;
#30240=VECTOR ( 'NONE', #27407, 1000.000000000000000 ) ;
#30244=LINE ( 'NONE', #25594, #167 ) ;
#30247=AXIS2_PLACEMENT_3D ( 'NONE', #8362, #17664, #29016 ) ;
#30248=DIRECTION ( 'NONE',  ( -2.698458740408365879E-16, 1.000000000000000000, 0.000000000000000000 ) ) ;
#30249=VERTEX_POINT ( 'NONE', #11102 ) ;
#30250=DIRECTION ( 'NONE',  ( -0.9510565162951536422, 0.000000000000000000, -0.3090169943749472292 ) ) ;
#30251=VERTEX_POINT ( 'NONE', #17668 ) ;
#30252=DIRECTION ( 'NONE',  ( -0.5877852522924731371, 0.000000000000000000, 0.8090169943749474513 ) ) ;
#30253=EDGE_LOOP ( 'NONE', ( #9958, #9918, #26261, #9471 ) ) ;
#30254=CARTESIAN_POINT ( 'NONE',  ( 130.7287565553229456, -9.999999999999982236, 3.500000000000003109 ) ) ;
#30255=ORIENTED_EDGE ( 'NONE', *, *, #26253, .F. ) ;
#30260=VERTEX_POINT ( 'NONE', #27479 ) ;
ENDSEC;
END-ISO-10303-21;
